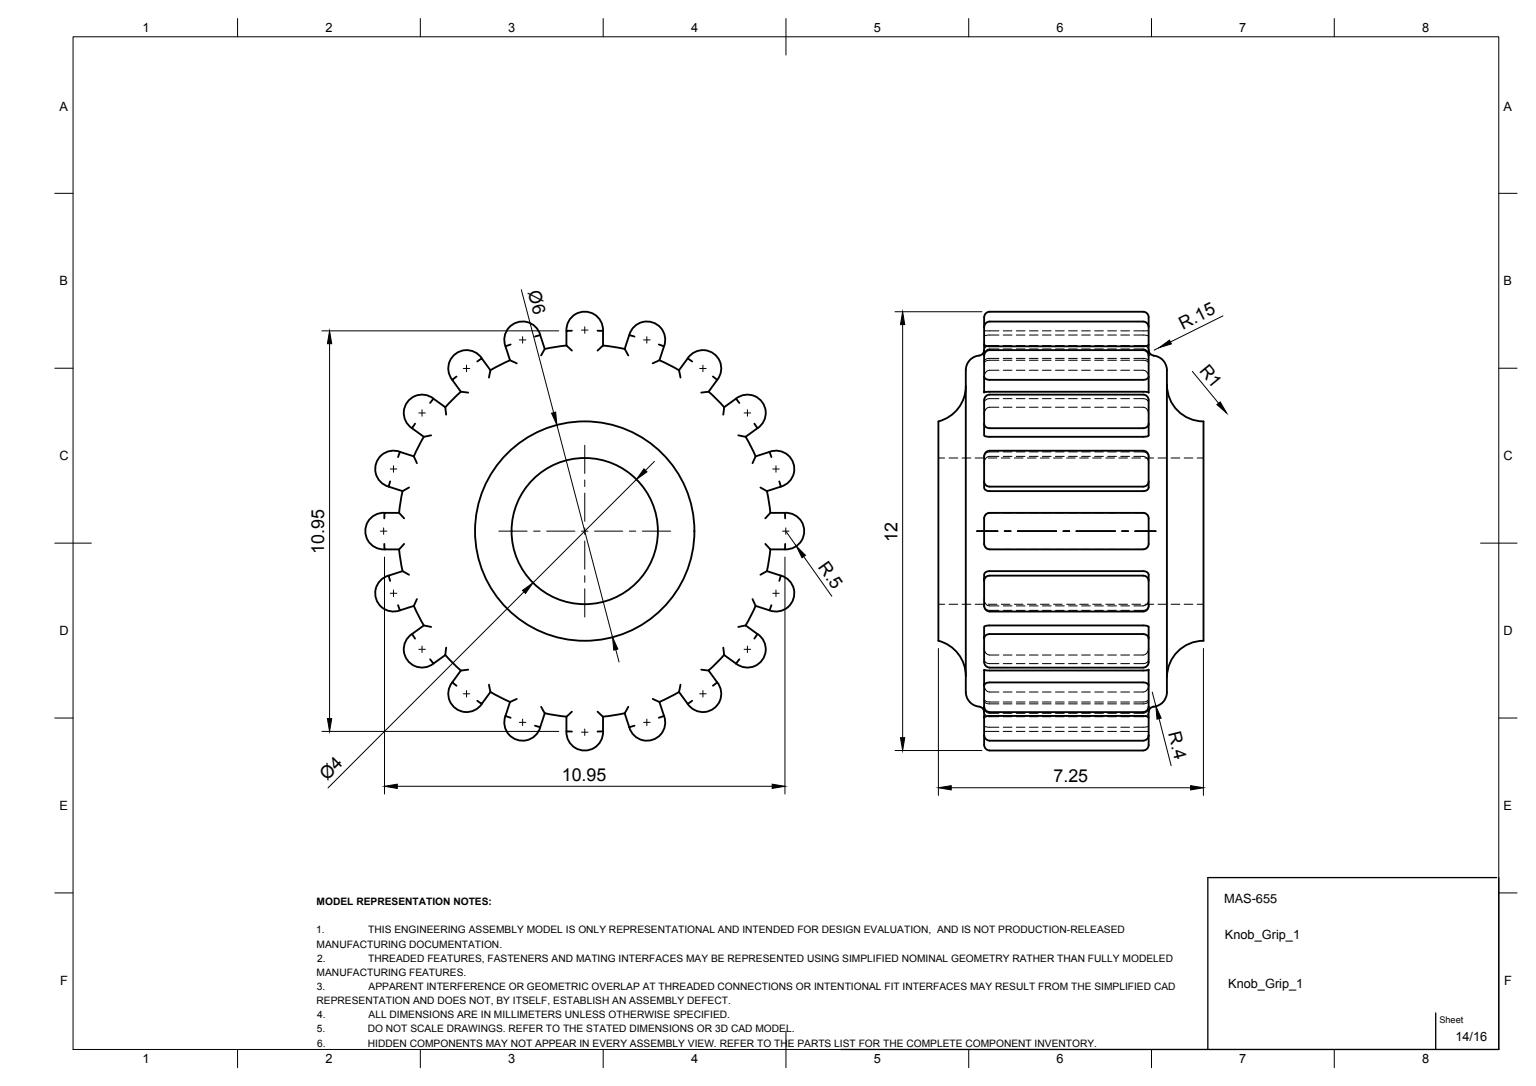
ISO-10303-21;
HEADER;
FILE_DESCRIPTION((''),'2;1');
FILE_NAME('Knob_Grip_1.step','2026-10-09T11:34:15-07:00',(''),(''),'','','');
FILE_SCHEMA (('AUTOMOTIVE_DESIGN { 1 0 10303 214 3 1 1 }'));
ENDSEC;
DATA;
#10=MECHANICAL_DESIGN_GEOMETRIC_PRESENTATION_REPRESENTATION('',(#646),#117170);
#604=SHAPE_REPRESENTATION_RELATIONSHIP('SRR','None',#117259,#625) ;
#625=ADVANCED_BREP_SHAPE_REPRESENTATION('',(#667),#117167) ;
#646=STYLED_ITEM('',(#117355),#667) ;
#667=MANIFOLD_SOLID_BREP('Body1',#49075) ;
#762=FACE_BOUND('',#16420,.T.) ;
#763=FACE_BOUND('',#16423,.T.) ;
#764=FACE_BOUND('',#16425,.T.) ;
#765=FACE_BOUND('',#16427,.T.) ;
#1361=B_SPLINE_CURVE_WITH_KNOTS('',3,(#101754,#101755,#101756,#101757,#101758,
#101759,#101760,#101761,#101762,#101763,#101764,#101765,#101766,#101767,
#101768,#101769),.UNSPECIFIED.,.T.,.F.,(4,1,1,1,1,1,1,1,1,1,1,1,1,4),(-1.37470975898194,
-1.17832265055595,-0.981935542129957,-0.785548433703966,-0.589161325277974,
-0.392774216851983,-0.196387108425991,0.,0.196387108425991,0.589161325277974,
0.785548433703966,0.981935542129957,1.17832265055595,1.37470975898194),
 .UNSPECIFIED.) ;
#1362=B_SPLINE_CURVE_WITH_KNOTS('',3,(#101778,#101779,#101780,#101781,#101782,
#101783,#101784,#101785,#101786,#101787,#101788,#101789,#101790,#101791,
#101792,#101793),.UNSPECIFIED.,.T.,.F.,(4,1,1,1,1,1,1,1,1,1,1,1,1,4),(-1.37470975898194,
-1.17832265055595,-0.981935542129957,-0.785548433703966,-0.589161325277974,
-0.392774216851983,-0.196387108425991,0.,0.196387108425991,0.589161325277974,
0.785548433703966,0.981935542129957,1.17832265055595,1.37470975898194),
 .UNSPECIFIED.) ;
#1363=B_SPLINE_CURVE_WITH_KNOTS('',3,(#101881,#101882,#101883,#101884,#101885),
 .UNSPECIFIED.,.F.,.F.,(4,1,4),(-1.,-0.5,0.),.UNSPECIFIED.) ;
#1364=B_SPLINE_CURVE_WITH_KNOTS('',3,(#101887,#101888,#101889,#101890,#101891,
#101892,#101893),.UNSPECIFIED.,.F.,.F.,(4,1,1,1,4),(-1.37470975898194,-1.17832265055595,
-0.981935542129957,-0.785548433703966,-0.68713324456091),.UNSPECIFIED.) ;
#1365=B_SPLINE_CURVE_WITH_KNOTS('',3,(#101894,#101895,#101896,#101897,#101898,
#101899,#101900,#101901,#101902,#101903,#101904,#101905,#101906),
 .UNSPECIFIED.,.F.,.F.,(4,1,1,1,1,1,1,1,1,1,4),(-0.68713324456091,-0.589161325277974,
-0.196387108425991,0.,0.196387108425991,0.392774216851983,0.589161325277974,
0.785548433703966,0.981935542129957,1.17832265055595,1.37470975898194),
 .UNSPECIFIED.) ;
#1366=B_SPLINE_CURVE_WITH_KNOTS('',3,(#101988,#101989,#101990,#101991,#101992),
 .UNSPECIFIED.,.F.,.F.,(4,1,4),(-1.,-0.5,0.),.UNSPECIFIED.) ;
#1367=B_SPLINE_CURVE_WITH_KNOTS('',3,(#101994,#101995,#101996,#101997,#101998,
#101999,#102000),.UNSPECIFIED.,.F.,.F.,(4,1,1,1,4),(-1.37470975898194,-1.17832265055595,
-0.981935542129957,-0.785548433703966,-0.687210817221056),.UNSPECIFIED.) ;
#1368=B_SPLINE_CURVE_WITH_KNOTS('',3,(#102001,#102002,#102003,#102004,#102005,
#102006,#102007,#102008,#102009,#102010,#102011,#102012,#102013),
 .UNSPECIFIED.,.F.,.F.,(4,1,1,1,1,1,1,1,1,1,4),(-0.687210817221056,-0.589161325277974,
-0.196387108425991,0.,0.196387108425991,0.392774216851983,0.589161325277974,
0.785548433703966,0.981935542129957,1.17832265055595,1.37470975898194),
 .UNSPECIFIED.) ;
#1369=B_SPLINE_CURVE_WITH_KNOTS('',3,(#102019,#102020,#102021,#102022,#102023,
#102024,#102025,#102026,#102027,#102028,#102029,#102030,#102031,#102032),
 .UNSPECIFIED.,.F.,.F.,(4,2,2,2,2,2,4),(-0.0559250143496373,-0.0556883945460747,
-0.0495906031992305,-0.0437546843030053,-0.0372885759081072,-0.0322854917709823,
-0.0278441972730634),.UNSPECIFIED.) ;
#1370=B_SPLINE_CURVE_WITH_KNOTS('',3,(#102035,#102036,#102037,#102038,#102039,
#102040,#102041,#102042,#102043,#102044,#102045,#102046,#102047,#102048),
 .UNSPECIFIED.,.F.,.F.,(4,2,2,2,2,2,4),(-0.000236619804093,0.,0.0060977913471935,
0.0119337102438738,0.018399818639261,0.0234029027767472,0.0278441972749678),
 .UNSPECIFIED.) ;
#1371=B_SPLINE_CURVE_WITH_KNOTS('',3,(#102053,#102054,#102055,#102056,#102057,
#102058,#102059,#102060,#102061,#102062,#102063,#102064,#102065,#102066,
#102067,#102068),.UNSPECIFIED.,.F.,.F.,(4,3,3,3,3,4),(-0.000437598556087367,
0.,0.00562170475705654,0.0114823251607832,0.0173413775084489,0.0231997078489075),
 .UNSPECIFIED.) ;
#1372=B_SPLINE_CURVE_WITH_KNOTS('',3,(#102074,#102075,#102076,#102077,#102078,
#102079,#102080,#102081,#102082,#102083,#102084,#102085,#102086,#102087,
#102088,#102089),.UNSPECIFIED.,.F.,.F.,(4,3,3,3,3,4),(-0.046837014255361,
-0.046399415699481,-0.0407777109422933,-0.0349170905383532,-0.0290580381904547,
-0.0231997078497599),.UNSPECIFIED.) ;
#1373=B_SPLINE_CURVE_WITH_KNOTS('',3,(#102095,#102096,#102097,#102098,#102099,
#102100,#102101,#102102,#102103,#102104,#102105,#102106,#102107,#102108),
 .UNSPECIFIED.,.F.,.F.,(4,2,2,2,2,2,4),(-0.000236619803146698,0.,0.00609779134724104,
0.0119337102438844,0.0183998186389394,0.0234029027761802,0.0278441972742087),
 .UNSPECIFIED.) ;
#1374=B_SPLINE_CURVE_WITH_KNOTS('',3,(#102114,#102115,#102116,#102117,#102118,
#102119,#102120,#102121,#102122,#102123,#102124,#102125,#102126,#102127),
 .UNSPECIFIED.,.F.,.F.,(4,2,2,2,2,2,4),(-0.0559250143496986,-0.0556883945465552,
-0.0495906031994403,-0.0437546843028884,-0.0372885759079096,-0.0322854917707418,
-0.0278441972727803),.UNSPECIFIED.) ;
#1375=B_SPLINE_CURVE_WITH_KNOTS('',3,(#102133,#102134,#102135,#102136,#102137,
#102138,#102139,#102140,#102141,#102142,#102143,#102144,#102145,#102146,
#102147,#102148),.UNSPECIFIED.,.F.,.F.,(4,3,3,3,3,4),(-0.000437598556095027,
0.,0.00562170475708189,0.0114823251608833,0.0173413775086171,0.0231997078491342),
 .UNSPECIFIED.) ;
#1376=B_SPLINE_CURVE_WITH_KNOTS('',3,(#102154,#102155,#102156,#102157,#102158,
#102159,#102160,#102161,#102162,#102163,#102164,#102165,#102166,#102167,
#102168,#102169),.UNSPECIFIED.,.F.,.F.,(4,3,3,3,3,4),(-0.0468370142541051,
-0.0463994156980201,-0.0407777109409428,-0.0349170905371886,-0.0290580381894966,
-0.0231997078490079),.UNSPECIFIED.) ;
#1377=B_SPLINE_CURVE_WITH_KNOTS('',3,(#102175,#102176,#102177,#102178,#102179,
#102180,#102181,#102182,#102183,#102184,#102185,#102186,#102187,#102188),
 .UNSPECIFIED.,.F.,.F.,(4,2,2,2,2,2,4),(-0.000236619803558265,0.,0.00609779134685418,
0.0119337102431074,0.0183998186379772,0.023402902775095,0.0278441972730209),
 .UNSPECIFIED.) ;
#1378=B_SPLINE_CURVE_WITH_KNOTS('',3,(#102194,#102195,#102196,#102197,#102198,
#102199,#102200,#102201,#102202,#102203,#102204,#102205,#102206,#102207),
 .UNSPECIFIED.,.F.,.F.,(4,2,2,2,2,2,4),(-0.0559250143504567,-0.0556883945473107,
-0.0495906032000867,-0.0437546843034773,-0.0372885759084374,-0.0322854917711889,
-0.0278441972731474),.UNSPECIFIED.) ;
#1379=B_SPLINE_CURVE_WITH_KNOTS('',3,(#102213,#102214,#102215,#102216,#102217,
#102218,#102219,#102220,#102221,#102222,#102223,#102224,#102225,#102226,
#102227,#102228),.UNSPECIFIED.,.F.,.F.,(4,3,3,3,3,4),(-0.000437598556114517,
0.,0.00562170475723958,0.0114823251612343,0.0173413775091901,0.0231997078499022),
 .UNSPECIFIED.) ;
#1380=B_SPLINE_CURVE_WITH_KNOTS('',3,(#102234,#102235,#102236,#102237,#102238,
#102239,#102240,#102241,#102242,#102243,#102244,#102245,#102246,#102247,
#102248,#102249),.UNSPECIFIED.,.F.,.F.,(4,3,3,3,3,4),(-0.0468370142516818,
-0.046399415695612,-0.0407777109388244,-0.034917090535398,-0.0290580381880315,
-0.0231997078478665),.UNSPECIFIED.) ;
#1381=B_SPLINE_CURVE_WITH_KNOTS('',3,(#102255,#102256,#102257,#102258,#102259,
#102260,#102261,#102262,#102263,#102264,#102265,#102266,#102267,#102268),
 .UNSPECIFIED.,.F.,.F.,(4,2,2,2,2,2,4),(-0.000236619803559768,0.,0.00609779134686269,
0.0119337102430971,0.0183998186379832,0.0234029027750867,0.0278441972729811),
 .UNSPECIFIED.) ;
#1382=B_SPLINE_CURVE_WITH_KNOTS('',3,(#102274,#102275,#102276,#102277,#102278,
#102279,#102280,#102281,#102282,#102283,#102284,#102285,#102286,#102287),
 .UNSPECIFIED.,.F.,.F.,(4,2,2,2,2,2,4),(-0.0559250143524368,-0.0556883945478243,
-0.0495906032010392,-0.0437546843047665,-0.0372885759096309,-0.0322854917723447,
-0.0278441972742818),.UNSPECIFIED.) ;
#1383=B_SPLINE_CURVE_WITH_KNOTS('',3,(#102293,#102294,#102295,#102296,#102297,
#102298,#102299,#102300,#102301,#102302,#102303,#102304,#102305,#102306,
#102307,#102308),.UNSPECIFIED.,.F.,.F.,(4,3,3,3,3,4),(-0.000437598556131605,
0.,0.00562170475733242,0.0114823251614144,0.0173413775094361,0.0231997078502398),
 .UNSPECIFIED.) ;
#1384=B_SPLINE_CURVE_WITH_KNOTS('',3,(#102314,#102315,#102316,#102317,#102318,
#102319,#102320,#102321,#102322,#102323,#102324,#102325,#102326,#102327,
#102328,#102329),.UNSPECIFIED.,.F.,.F.,(4,3,3,3,3,4),(-0.0468370142582233,
-0.0463994157019922,-0.0407777109444557,-0.0349170905401249,-0.0290580381918459,
-0.0231997078507989),.UNSPECIFIED.) ;
#1385=B_SPLINE_CURVE_WITH_KNOTS('',3,(#102335,#102336,#102337,#102338,#102339,
#102340,#102341,#102342,#102343,#102344,#102345,#102346,#102347,#102348),
 .UNSPECIFIED.,.F.,.F.,(4,2,2,2,2,2,4),(-0.000236619803154501,0.,0.00609779134749395,
0.0119337102444787,0.0183998186399401,0.0234029027774939,0.0278441972757804),
 .UNSPECIFIED.) ;
#1386=B_SPLINE_CURVE_WITH_KNOTS('',3,(#102354,#102355,#102356,#102357,#102358,
#102359,#102360,#102361,#102362,#102363,#102364,#102365,#102366,#102367),
 .UNSPECIFIED.,.F.,.F.,(4,2,2,2,2,2,4),(-0.0559250143516698,-0.055688394548102,
-0.0495906032010132,-0.0437546843045191,-0.0372885759093257,-0.0322854917720022,
-0.0278441972739074),.UNSPECIFIED.) ;
#1387=B_SPLINE_CURVE_WITH_KNOTS('',3,(#102373,#102374,#102375,#102376,#102377,
#102378,#102379,#102380,#102381,#102382,#102383,#102384,#102385,#102386,
#102387,#102388),.UNSPECIFIED.,.F.,.F.,(4,3,3,3,3,4),(-0.000437598556150276,
0.,0.00562170475744494,0.0114823251616921,0.0173413775098778,0.0231997078508276),
 .UNSPECIFIED.) ;
#1388=B_SPLINE_CURVE_WITH_KNOTS('',3,(#102394,#102395,#102396,#102397,#102398,
#102399,#102400,#102401,#102402,#102403,#102404,#102405,#102406,#102407,
#102408,#102409),.UNSPECIFIED.,.F.,.F.,(4,3,3,3,3,4),(-0.0468370142569828,
-0.0463994157014635,-0.0407777109440522,-0.0349170905398014,-0.0290580381915951,
-0.0231997078506218),.UNSPECIFIED.) ;
#1389=B_SPLINE_CURVE_WITH_KNOTS('',3,(#102415,#102416,#102417,#102418,#102419,
#102420,#102421,#102422,#102423,#102424,#102425,#102426,#102427,#102428),
 .UNSPECIFIED.,.F.,.F.,(4,2,2,2,2,2,4),(-0.000236619804616541,0.,0.00609779134700319,
0.0119337102434886,0.0183998186388943,0.0234029027763847,0.0278441972746185),
 .UNSPECIFIED.) ;
#1390=B_SPLINE_CURVE_WITH_KNOTS('',3,(#102434,#102435,#102436,#102437,#102438,
#102439,#102440,#102441,#102442,#102443,#102444,#102445,#102446,#102447),
 .UNSPECIFIED.,.F.,.F.,(4,2,2,2,2,2,4),(-0.0559250143475551,-0.0556883945439973,
-0.049590603197355,-0.0437546843013896,-0.037288575906807,-0.0322854917699323,
-0.0278441972722247),.UNSPECIFIED.) ;
#1391=B_SPLINE_CURVE_WITH_KNOTS('',3,(#102453,#102454,#102455,#102456,#102457,
#102458,#102459,#102460,#102461,#102462,#102463,#102464,#102465,#102466,
#102467,#102468),.UNSPECIFIED.,.F.,.F.,(4,3,3,3,3,4),(-0.000437598556056009,
0.,0.00562170475686937,0.0114823251603833,0.0173413775078316,0.0231997078480834),
 .UNSPECIFIED.) ;
#1392=B_SPLINE_CURVE_WITH_KNOTS('',3,(#102474,#102475,#102476,#102477,#102478,
#102479,#102480,#102481,#102482,#102483,#102484,#102485,#102486,#102487,
#102488,#102489),.UNSPECIFIED.,.F.,.F.,(4,3,3,3,3,4),(-0.0468370142561097,
-0.0463994157004828,-0.0407777109431283,-0.034917090538975,-0.0290580381908889,
-0.0231997078500392),.UNSPECIFIED.) ;
#1393=B_SPLINE_CURVE_WITH_KNOTS('',3,(#102495,#102496,#102497,#102498,#102499,
#102500,#102501,#102502,#102503,#102504,#102505,#102506,#102507,#102508),
 .UNSPECIFIED.,.F.,.F.,(4,2,2,2,2,2,4),(-0.000236619804206572,0.,0.00609779134739848,
0.0119337102443252,0.0183998186399927,0.023402902777706,0.0278441972760964),
 .UNSPECIFIED.) ;
#1394=B_SPLINE_CURVE_WITH_KNOTS('',3,(#102514,#102515,#102516,#102517,#102518,
#102519,#102520,#102521,#102522,#102523,#102524,#102525,#102526,#102527),
 .UNSPECIFIED.,.F.,.F.,(4,2,2,2,2,2,4),(-0.0559250143503367,-0.0556883945467745,
-0.0495906031998185,-0.0437546843034772,-0.0372885759085197,-0.0322854917713411,
-0.0278441972733722),.UNSPECIFIED.) ;
#1395=B_SPLINE_CURVE_WITH_KNOTS('',3,(#102533,#102534,#102535,#102536,#102537,
#102538,#102539,#102540,#102541,#102542,#102543,#102544,#102545,#102546,
#102547,#102548),.UNSPECIFIED.,.F.,.F.,(4,3,3,3,3,4),(-0.000437598556095159,
0.,0.00562170475710087,0.0114823251609001,0.0173413775086179,0.0231997078491324),
 .UNSPECIFIED.) ;
#1396=B_SPLINE_CURVE_WITH_KNOTS('',3,(#102554,#102555,#102556,#102557,#102558,
#102559,#102560,#102561,#102562,#102563,#102564,#102565,#102566,#102567,
#102568,#102569),.UNSPECIFIED.,.F.,.F.,(4,3,3,3,3,4),(-0.0468370142542446,
-0.0463994156981747,-0.0407777109410807,-0.0349170905373078,-0.0290580381895938,
-0.0231997078490836),.UNSPECIFIED.) ;
#1397=B_SPLINE_CURVE_WITH_KNOTS('',3,(#102575,#102576,#102577,#102578,#102579,
#102580,#102581,#102582,#102583,#102584,#102585,#102586,#102587,#102588),
 .UNSPECIFIED.,.F.,.F.,(4,2,2,2,2,2,4),(-0.000236619803563725,0.,0.00609779134693619,
0.0119337102432759,0.0183998186382373,0.0234029027754271,0.027844197273412),
 .UNSPECIFIED.) ;
#1398=B_SPLINE_CURVE_WITH_KNOTS('',3,(#102594,#102595,#102596,#102597,#102598,
#102599,#102600,#102601,#102602,#102603,#102604,#102605,#102606,#102607),
 .UNSPECIFIED.,.F.,.F.,(4,2,2,2,2,2,4),(-0.0559250143564113,-0.0556883945522011,
-0.0495906032047249,-0.0437546843077159,-0.0372885759119513,-0.0322854917741759,
-0.0278441972757216),.UNSPECIFIED.) ;
#1399=B_SPLINE_CURVE_WITH_KNOTS('',3,(#102613,#102614,#102615,#102616,#102617,
#102618,#102619,#102620,#102621,#102622,#102623,#102624,#102625,#102626,
#102627,#102628),.UNSPECIFIED.,.F.,.F.,(4,3,3,3,3,4),(-0.000437598556252948,
0.,0.00562170475756358,0.0114823251619473,0.0173413775102792,0.023199707851373),
 .UNSPECIFIED.) ;
#1400=B_SPLINE_CURVE_WITH_KNOTS('',3,(#102634,#102635,#102636,#102637,#102638,
#102639,#102640,#102641,#102642,#102643,#102644,#102645,#102646,#102647,
#102648,#102649),.UNSPECIFIED.,.F.,.F.,(4,3,3,3,3,4),(-0.0468370142435449,
-0.0463994156880452,-0.0407777109322271,-0.0349170905298351,-0.0290580381834779,
-0.0231997078443083),.UNSPECIFIED.) ;
#1401=B_SPLINE_CURVE_WITH_KNOTS('',3,(#102655,#102656,#102657,#102658,#102659,
#102660,#102661,#102662,#102663,#102664,#102665,#102666,#102667,#102668),
 .UNSPECIFIED.,.F.,.F.,(4,2,2,2,2,2,4),(-0.000236619803545348,0.,0.00609779134648851,
0.0119337102422953,0.0183998186366923,0.0234029027734222,0.0278441972710204),
 .UNSPECIFIED.) ;
#1402=B_SPLINE_CURVE_WITH_KNOTS('',3,(#102674,#102675,#102676,#102677,#102678,
#102679,#102680,#102681,#102682,#102683,#102684,#102685,#102686,#102687),
 .UNSPECIFIED.,.F.,.F.,(4,2,2,2,2,2,4),(-0.0559250143495547,-0.0556883945459923,
-0.0495906031991245,-0.0437546843029074,-0.0372885759080479,-0.0322854917709575,
-0.027844197273083),.UNSPECIFIED.) ;
#1403=B_SPLINE_CURVE_WITH_KNOTS('',3,(#102693,#102694,#102695,#102696,#102697,
#102698,#102699,#102700,#102701,#102702,#102703,#102704,#102705,#102706,
#102707,#102708),.UNSPECIFIED.,.F.,.F.,(4,3,3,3,3,4),(-0.000437598556080383,
0.,0.00562170475701161,0.0114823251606741,0.0173413775082905,0.0231997078487108),
 .UNSPECIFIED.) ;
#1404=B_SPLINE_CURVE_WITH_KNOTS('',3,(#102714,#102715,#102716,#102717,#102718,
#102719,#102720,#102721,#102722,#102723,#102724,#102725,#102726,#102727,
#102728,#102729),.UNSPECIFIED.,.F.,.F.,(4,3,3,3,3,4),(-0.0468370142410635,
-0.046399415685515,-0.0407777109299654,-0.0349170905279156,-0.0290580381819153,
-0.0231997078430871),.UNSPECIFIED.) ;
#1405=B_SPLINE_CURVE_WITH_KNOTS('',3,(#102735,#102736,#102737,#102738,#102739,
#102740,#102741,#102742,#102743,#102744,#102745,#102746,#102747,#102748),
 .UNSPECIFIED.,.F.,.F.,(4,2,2,2,2,2,4),(-0.000236619803553881,0.,0.00609779134648714,
0.0119337102422593,0.0183998186365944,0.0234029027733178,0.0278441972709114),
 .UNSPECIFIED.) ;
#1406=B_SPLINE_CURVE_WITH_KNOTS('',3,(#102754,#102755,#102756,#102757,#102758,
#102759,#102760,#102761,#102762,#102763,#102764,#102765,#102766,#102767),
 .UNSPECIFIED.,.F.,.F.,(4,2,2,2,2,2,4),(-0.0559250143458346,-0.0556883945427038,
-0.0495906031960554,-0.043754684300065,-0.0372885759056522,-0.0322854917688908,
-0.0278441972712752),.UNSPECIFIED.) ;
#1407=B_SPLINE_CURVE_WITH_KNOTS('',3,(#102773,#102774,#102775,#102776,#102777,
#102778,#102779,#102780,#102781,#102782,#102783,#102784,#102785,#102786,
#102787,#102788),.UNSPECIFIED.,.F.,.F.,(4,3,3,3,3,4),(-0.000437598556037642,
0.,0.00562170475676515,0.0114823251601515,0.0173413775075229,0.0231997078477011),
 .UNSPECIFIED.) ;
#1408=B_SPLINE_CURVE_WITH_KNOTS('',3,(#102794,#102795,#102796,#102797,#102798,
#102799,#102800,#102801,#102802,#102803,#102804,#102805,#102806,#102807,
#102808,#102809),.UNSPECIFIED.,.F.,.F.,(4,3,3,3,3,4),(-0.0468370142550307,
-0.046399415699245,-0.0407777109420836,-0.0349170905381485,-0.0290580381902572,
-0.023199707849583),.UNSPECIFIED.) ;
#1409=B_SPLINE_CURVE_WITH_KNOTS('',3,(#102815,#102816,#102817,#102818,#102819,
#102820,#102821,#102822,#102823,#102824,#102825,#102826,#102827,#102828),
 .UNSPECIFIED.,.F.,.F.,(4,2,2,2,2,2,4),(-0.000236619803565948,0.,0.00609779134700125,
0.0119337102434307,0.0183998186384978,0.0234029027757452,0.0278441972737845),
 .UNSPECIFIED.) ;
#1410=B_SPLINE_CURVE_WITH_KNOTS('',3,(#102834,#102835,#102836,#102837,#102838,
#102839,#102840,#102841,#102842,#102843,#102844,#102845,#102846,#102847),
 .UNSPECIFIED.,.F.,.F.,(4,2,2,2,2,2,4),(-0.0559250143492506,-0.0556883945457476,
-0.049590603198939,-0.0437546843027145,-0.0372885759078682,-0.032285491770796,
-0.0278441972729179),.UNSPECIFIED.) ;
#1411=B_SPLINE_CURVE_WITH_KNOTS('',3,(#102854,#102855,#102856,#102857,#102858,
#102859,#102860,#102861,#102862,#102863,#102864,#102865,#102866,#102867,
#102868,#102869),.UNSPECIFIED.,.F.,.F.,(4,3,3,3,3,4),(-0.000437598556107252,
0.,0.00562170475708925,0.0114823251608564,0.0173413775085622,0.0231997078490661),
 .UNSPECIFIED.) ;
#1412=B_SPLINE_CURVE_WITH_KNOTS('',3,(#102875,#102876,#102877,#102878,#102879,
#102880,#102881,#102882,#102883,#102884,#102885,#102886,#102887,#102888,
#102889,#102890),.UNSPECIFIED.,.F.,.F.,(4,3,3,3,3,4),(-0.0468370142553995,
-0.0463994157003126,-0.0407777109430307,-0.0349170905389541,-0.0290580381909493,
-0.0231997078501516),.UNSPECIFIED.) ;
#1413=B_SPLINE_CURVE_WITH_KNOTS('',3,(#102896,#102897,#102898,#102899,#102900,
#102901,#102902,#102903,#102904,#102905,#102906,#102907,#102908,#102909),
 .UNSPECIFIED.,.F.,.F.,(4,2,2,2,2,2,4),(-0.000236619803559952,0.,0.00609779134694098,
0.0119337102432763,0.0183998186382272,0.0234029027754186,0.0278441972733939),
 .UNSPECIFIED.) ;
#1414=B_SPLINE_CURVE_WITH_KNOTS('',3,(#102915,#102916,#102917,#102918,#102919,
#102920,#102921,#102922,#102923,#102924,#102925,#102926,#102927,#102928),
 .UNSPECIFIED.,.F.,.F.,(4,2,2,2,2,2,4),(-0.0559250143507825,-0.0556883945467992,
-0.0495906032001226,-0.043754684304009,-0.0372885759090493,-0.032285491771857,
-0.0278441972738728),.UNSPECIFIED.) ;
#1415=B_SPLINE_CURVE_WITH_KNOTS('',3,(#102934,#102935,#102936,#102937,#102938,
#102939,#102940,#102941,#102942,#102943,#102944,#102945,#102946,#102947,
#102948,#102949),.UNSPECIFIED.,.F.,.F.,(4,3,3,3,3,4),(-0.000437598556095639,
0.,0.00562170475706734,0.0114823251608502,0.0173413775085488,0.0231997078490271),
 .UNSPECIFIED.) ;
#1416=B_SPLINE_CURVE_WITH_KNOTS('',3,(#102955,#102956,#102957,#102958,#102959,
#102960,#102961,#102962,#102963,#102964,#102965,#102966,#102967,#102968,
#102969,#102970),.UNSPECIFIED.,.F.,.F.,(4,3,3,3,3,4),(-0.0468370142543074,
-0.0463994156982126,-0.0407777109411238,-0.0349170905373201,-0.0290580381896051,
-0.0231997078491063),.UNSPECIFIED.) ;
#1417=B_SPLINE_CURVE_WITH_KNOTS('',3,(#102976,#102977,#102978,#102979,#102980,
#102981,#102982,#102983,#102984,#102985,#102986,#102987,#102988,#102989),
 .UNSPECIFIED.,.F.,.F.,(4,2,2,2,2,2,4),(-0.000236619803981649,0.,0.00609779134664719,
0.0119337102427236,0.0183998186376455,0.0234029027747974,0.0278441972727449),
 .UNSPECIFIED.) ;
#1418=B_SPLINE_CURVE_WITH_KNOTS('',3,(#102995,#102996,#102997,#102998,#102999,
#103000,#103001,#103002,#103003,#103004,#103005,#103006,#103007,#103008),
 .UNSPECIFIED.,.F.,.F.,(4,2,2,2,2,2,4),(-0.055925014352087,-0.0556883945480977,
-0.0495906032012405,-0.0437546843049561,-0.0372885759098064,-0.0322854917724869,
-0.0278441972743996),.UNSPECIFIED.) ;
#1419=B_SPLINE_CURVE_WITH_KNOTS('',3,(#103014,#103015,#103016,#103017,#103018,
#103019,#103020,#103021,#103022,#103023,#103024,#103025,#103026,#103027,
#103028,#103029),.UNSPECIFIED.,.F.,.F.,(4,3,3,3,3,4),(-0.000437598556128711,
0.,0.00562170475726701,0.0114823251612751,0.0173413775092439,0.0231997078500064),
 .UNSPECIFIED.) ;
#1420=B_SPLINE_CURVE_WITH_KNOTS('',3,(#103035,#103036,#103037,#103038,#103039,
#103040,#103041,#103042,#103043,#103044,#103045,#103046,#103047,#103048,
#103049,#103050),.UNSPECIFIED.,.F.,.F.,(4,3,3,3,3,4),(-0.0468370142525421,
-0.046399415696666,-0.0407777109397685,-0.0349170905362003,-0.029058038188693,
-0.0231997078483865),.UNSPECIFIED.) ;
#1421=B_SPLINE_CURVE_WITH_KNOTS('',3,(#103056,#103057,#103058,#103059,#103060,
#103061,#103062,#103063,#103064,#103065,#103066,#103067,#103068,#103069),
 .UNSPECIFIED.,.F.,.F.,(4,2,2,2,2,2,4),(-0.000236619803982414,0.,0.00609779134661,
0.0119337102426289,0.0183998186375097,0.0234029027746178,0.0278441972725225),
 .UNSPECIFIED.) ;
#1422=B_SPLINE_CURVE_WITH_KNOTS('',3,(#103075,#103076,#103077,#103078,#103079,
#103080,#103081,#103082,#103083,#103084,#103085,#103086,#103087,#103088),
 .UNSPECIFIED.,.F.,.F.,(4,2,2,2,2,2,4),(-0.0559250143493171,-0.0556883945461739,
-0.0495906031990541,-0.0437546843026118,-0.037288575907723,-0.0322854917706097,
-0.0278441972727174),.UNSPECIFIED.) ;
#1423=B_SPLINE_CURVE_WITH_KNOTS('',3,(#103094,#103095,#103096,#103097,#103098,
#103099,#103100,#103101,#103102,#103103,#103104,#103105,#103106,#103107,
#103108,#103109),.UNSPECIFIED.,.F.,.F.,(4,3,3,3,3,4),(-0.000437598556087196,
0.,0.00562170475699019,0.0114823251606472,0.0173413775082489,0.0231997078486377),
 .UNSPECIFIED.) ;
#1424=B_SPLINE_CURVE_WITH_KNOTS('',3,(#103115,#103116,#103117,#103118,#103119,
#103120,#103121,#103122,#103123,#103124,#103125,#103126,#103127,#103128,
#103129,#103130),.UNSPECIFIED.,.F.,.F.,(4,3,3,3,3,4),(-0.0468370142500863,
-0.0463994156945211,-0.0407777109379294,-0.0349170905346585,-0.0290580381874365,
-0.0231997078474141),.UNSPECIFIED.) ;
#1425=B_SPLINE_CURVE_WITH_KNOTS('',3,(#103136,#103137,#103138,#103139,#103140,
#103141,#103142,#103143,#103144,#103145,#103146,#103147,#103148,#103149),
 .UNSPECIFIED.,.F.,.F.,(4,2,2,2,2,2,4),(-0.000236619803560014,0.,0.00609779134678491,
0.0119337102429536,0.0183998186377476,0.0234029027747679,0.0278441972725981),
 .UNSPECIFIED.) ;
#1426=B_SPLINE_CURVE_WITH_KNOTS('',3,(#103155,#103156,#103157,#103158,#103159,
#103160,#103161,#103162,#103163,#103164,#103165,#103166,#103167,#103168),
 .UNSPECIFIED.,.F.,.F.,(4,2,2,2,2,2,4),(-0.0559250143548778,-0.0556883945506748,
-0.0495906032033264,-0.0437546843064839,-0.0372885759109464,-0.0322854917733345,
-0.0278441972750097),.UNSPECIFIED.) ;
#1427=B_SPLINE_CURVE_WITH_KNOTS('',3,(#103174,#103175,#103176,#103177,#103178,
#103179,#103180,#103181,#103182,#103183,#103184,#103185,#103186,#103187,
#103188,#103189),.UNSPECIFIED.,.F.,.F.,(4,3,3,3,3,4),(-0.000437598556223204,
0.,0.00562170475783914,0.0114823251625445,0.0173413775111918,0.0231997078526027),
 .UNSPECIFIED.) ;
#1428=B_SPLINE_CURVE_WITH_KNOTS('',3,(#103195,#103196,#103197,#103198,#103199,
#103200,#103201,#103202,#103203,#103204,#103205,#103206,#103207,#103208,
#103209,#103210),.UNSPECIFIED.,.F.,.F.,(4,3,3,3,3,4),(-0.0468370142563843,
-0.046399415700489,-0.0407777109431322,-0.0349170905389995,-0.0290580381909307,
-0.0231997078501088),.UNSPECIFIED.) ;
#1429=B_SPLINE_CURVE_WITH_KNOTS('',3,(#103216,#103217,#103218,#103219,#103220,
#103221,#103222,#103223,#103224,#103225,#103226,#103227,#103228,#103229),
 .UNSPECIFIED.,.F.,.F.,(4,2,2,2,2,2,4),(-0.000236619804200277,0.,0.00609779134716414,
0.0119337102438048,0.0183998186391783,0.0234029027766296,0.0278441972748296),
 .UNSPECIFIED.) ;
#1430=B_SPLINE_CURVE_WITH_KNOTS('',3,(#103235,#103236,#103237,#103238,#103239,
#103240,#103241,#103242,#103243,#103244,#103245,#103246,#103247,#103248),
 .UNSPECIFIED.,.F.,.F.,(4,2,2,2,2,2,4),(-0.0559250143496621,-0.0556883945461033,
-0.0495906031992651,-0.0437546843029983,-0.0372885759081094,-0.032285491771005,
-0.02784419727311),.UNSPECIFIED.) ;
#1431=B_SPLINE_CURVE_WITH_KNOTS('',3,(#103254,#103255,#103256,#103257,#103258,
#103259,#103260,#103261,#103262,#103263,#103264,#103265,#103266,#103267,
#103268,#103269),.UNSPECIFIED.,.F.,.F.,(4,3,3,3,3,4),(-0.000437598556084584,
0.,0.00562170475697965,0.0114823251606079,0.0173413775081775,0.0231997078485472),
 .UNSPECIFIED.) ;
#1432=B_SPLINE_CURVE_WITH_KNOTS('',3,(#103275,#103276,#103277,#103278,#103279,
#103280,#103281,#103282,#103283,#103284,#103285,#103286,#103287,#103288,
#103289,#103290),.UNSPECIFIED.,.F.,.F.,(4,3,3,3,3,4),(-0.0468370142549382,
-0.0463994156994604,-0.0407777109422707,-0.0349170905383382,-0.0290580381904463,
-0.023199707849757),.UNSPECIFIED.) ;
#1433=B_SPLINE_CURVE_WITH_KNOTS('',3,(#103296,#103297,#103298,#103299,#103300,
#103301,#103302,#103303,#103304,#103305,#103306,#103307,#103308,#103309),
 .UNSPECIFIED.,.F.,.F.,(4,2,2,2,2,2,4),(-0.000236619803568316,0.,0.00609779134701837,
0.0119337102434465,0.0183998186385035,0.0234029027757473,0.0278441972737745),
 .UNSPECIFIED.) ;
#1434=B_SPLINE_CURVE_WITH_KNOTS('',3,(#103315,#103316,#103317,#103318,#103319,
#103320,#103321,#103322,#103323,#103324,#103325,#103326,#103327,#103328),
 .UNSPECIFIED.,.F.,.F.,(4,2,2,2,2,2,4),(-0.0559250143499934,-0.0556883945464304,
-0.0495906031995064,-0.0437546843032007,-0.037288575908277,-0.032285491771123,
-0.0278441972731808),.UNSPECIFIED.) ;
#1435=B_SPLINE_CURVE_WITH_KNOTS('',3,(#103334,#103335,#103336,#103337,#103338,
#103339,#103340,#103341,#103342,#103343,#103344,#103345,#103346,#103347,
#103348,#103349),.UNSPECIFIED.,.F.,.F.,(4,3,3,3,3,4),(-0.000437598556092419,
0.,0.00562170475702671,0.0114823251607112,0.0173413775083605,0.0231997078487915),
 .UNSPECIFIED.) ;
#1436=B_SPLINE_CURVE_WITH_KNOTS('',3,(#103355,#103356,#103357,#103358,#103359,
#103360,#103361,#103362,#103363,#103364,#103365,#103366,#103367,#103368,
#103369,#103370),.UNSPECIFIED.,.F.,.F.,(4,3,3,3,3,4),(-0.0468370142548351,
-0.0463994156987323,-0.0407777109416122,-0.0349170905377609,-0.0290580381899607,
-0.0231997078493697),.UNSPECIFIED.) ;
#1437=B_SPLINE_CURVE_WITH_KNOTS('',3,(#103376,#103377,#103378,#103379,#103380,
#103381,#103382,#103383,#103384,#103385,#103386,#103387,#103388,#103389),
 .UNSPECIFIED.,.F.,.F.,(4,2,2,2,2,2,4),(-0.000236619803562033,0.,0.00609779134691358,
0.0119337102432247,0.0183998186381566,0.0234029027753094,0.027844197273255),
 .UNSPECIFIED.) ;
#1438=B_SPLINE_CURVE_WITH_KNOTS('',3,(#103395,#103396,#103397,#103398,#103399,
#103400,#103401,#103402,#103403,#103404,#103405,#103406,#103407,#103408),
 .UNSPECIFIED.,.F.,.F.,(4,2,2,2,2,2,4),(-0.0559250143503813,-0.0556883945472345,
-0.0495906032000065,-0.0437546843033907,-0.0372885759083472,-0.0322854917711086,
-0.027844197273083),.UNSPECIFIED.) ;
#1439=B_SPLINE_CURVE_WITH_KNOTS('',3,(#103414,#103415,#103416,#103417,#103418,
#103419,#103420,#103421,#103422,#103423,#103424,#103425,#103426,#103427,
#103428,#103429),.UNSPECIFIED.,.F.,.F.,(4,3,3,3,3,4),(-0.000437598556129241,
0.,0.00562170475730571,0.0114823251613513,0.0173413775093445,0.0231997078501172),
 .UNSPECIFIED.) ;
#1440=B_SPLINE_CURVE_WITH_KNOTS('',3,(#103435,#103436,#103437,#103438,#103439,
#103440,#103441,#103442,#103443,#103444,#103445,#103446,#103447,#103448,
#103449,#103450),.UNSPECIFIED.,.F.,.F.,(4,3,3,3,3,4),(-0.0468370142515845,
-0.0463994156955989,-0.0407777109388572,-0.0349170905354382,-0.0290580381880585,
-0.0231997078478789),.UNSPECIFIED.) ;
#1441=B_SPLINE_CURVE_WITH_KNOTS('',3,(#103456,#103457,#103458,#103459,#103460,
#103461,#103462,#103463,#103464,#103465,#103466,#103467,#103468,#103469),
 .UNSPECIFIED.,.F.,.F.,(4,2,2,2,2,2,4),(-0.000236619803559663,0.,0.0060977913468164,
0.0119337102430072,0.0183998186378663,0.0234029027749556,0.0278441972728503),
 .UNSPECIFIED.) ;
#1442=B_SPLINE_CURVE_WITH_KNOTS('',3,(#103475,#103476,#103477,#103478,#103479,
#103480,#103481,#103482,#103483,#103484,#103485,#103486,#103487,#103488),
 .UNSPECIFIED.,.F.,.F.,(4,2,2,2,2,2,4),(-0.0559250143533661,-0.0556883945491649,
-0.0495906032019838,-0.0437546843053393,-0.0372885759099808,-0.0322854917725361,
-0.0278441972743507),.UNSPECIFIED.) ;
#1443=B_SPLINE_CURVE_WITH_KNOTS('',3,(#103494,#103495,#103496,#103497,#103498,
#103499,#103500,#103501,#103502,#103503,#103504,#103505,#103506,#103507,
#103508,#103509),.UNSPECIFIED.,.F.,.F.,(4,3,3,3,3,4),(-0.00043759855615984,
0.,0.00562170475737693,0.011482325161534,0.017341377509665,0.0231997078505602),
 .UNSPECIFIED.) ;
#1444=B_SPLINE_CURVE_WITH_KNOTS('',3,(#103515,#103516,#103517,#103518,#103519,
#103520,#103521,#103522,#103523,#103524,#103525,#103526,#103527,#103528,
#103529,#103530),.UNSPECIFIED.,.F.,.F.,(4,3,3,3,3,4),(-0.0468370142504761,
-0.0463994156944377,-0.0407777109378315,-0.0349170905345851,-0.0290580381873817,
-0.0231997078473671),.UNSPECIFIED.) ;
#1445=B_SPLINE_CURVE_WITH_KNOTS('',3,(#103536,#103537,#103538,#103539,#103540,
#103541,#103542,#103543,#103544,#103545,#103546,#103547,#103548,#103549),
 .UNSPECIFIED.,.F.,.F.,(4,2,2,2,2,2,4),(-0.000236619803559426,0.,0.00609779134674399,
0.0119337102428204,0.0183998186375428,0.0234029027745216,0.0278441972723019),
 .UNSPECIFIED.) ;
#1446=B_SPLINE_CURVE_WITH_KNOTS('',3,(#103555,#103556,#103557,#103558,#103559,
#103560,#103561,#103562,#103563,#103564,#103565,#103566,#103567,#103568),
 .UNSPECIFIED.,.F.,.F.,(4,2,2,2,2,2,4),(-0.0559250143520313,-0.0556883945484605,
-0.0495906032013131,-0.0437546843047777,-0.037288575909542,-0.0322854917721873,
-0.0278441972740755),.UNSPECIFIED.) ;
#1447=B_SPLINE_CURVE_WITH_KNOTS('',3,(#103574,#103575,#103576,#103577,#103578,
#103579,#103580,#103581,#103582,#103583,#103584,#103585,#103586,#103587,
#103588,#103589),.UNSPECIFIED.,.F.,.F.,(4,3,3,3,3,4),(-0.000437598556142791,
0.,0.00562170475737048,0.011482325161532,0.0173413775096432,0.0231997078505159),
 .UNSPECIFIED.) ;
#1448=B_SPLINE_CURVE_WITH_KNOTS('',3,(#103595,#103596,#103597,#103598,#103599,
#103600,#103601,#103602,#103603,#103604,#103605,#103606,#103607,#103608,
#103609,#103610),.UNSPECIFIED.,.F.,.F.,(4,3,3,3,3,4),(-0.046837014256793,
-0.0463994157012118,-0.0407777109438107,-0.0349170905396121,-0.0290580381914533,
-0.0231997078505249),.UNSPECIFIED.) ;
#1449=B_SPLINE_CURVE_WITH_KNOTS('',3,(#104026,#104027,#104028,#104029,#104030,
#104031,#104032,#104033,#104034,#104035,#104036,#104037,#104038,#104039),
 .UNSPECIFIED.,.F.,.F.,(4,2,2,2,2,2,4),(-0.0559250143525619,-0.0556883945479474,
-0.0495906032011524,-0.0437546843048812,-0.037288575909754,-0.0322854917724513,
-0.027844197274366),.UNSPECIFIED.) ;
#1450=B_SPLINE_CURVE_WITH_KNOTS('',3,(#104042,#104043,#104044,#104045,#104046,
#104047,#104048,#104049,#104050,#104051,#104052,#104053,#104054,#104055),
 .UNSPECIFIED.,.F.,.F.,(4,2,2,2,2,2,4),(-0.000236619803144863,0.,0.00609779134711087,
0.0119337102436339,0.0183998186386153,0.0234029027758149,0.0278441972738027),
 .UNSPECIFIED.) ;
#1451=B_SPLINE_CURVE_WITH_KNOTS('',3,(#104058,#104059,#104060,#104061,#104062,
#104063,#104064,#104065,#104066,#104067,#104068,#104069,#104070,#104071,
#104072,#104073),.UNSPECIFIED.,.F.,.F.,(4,3,3,3,3,4),(-0.000437598556136612,
0.,0.00562170475739987,0.0114823251615695,0.0173413775096577,0.0231997078505359),
 .UNSPECIFIED.) ;
#1452=B_SPLINE_CURVE_WITH_KNOTS('',3,(#104078,#104079,#104080,#104081,#104082,
#104083,#104084,#104085,#104086,#104087,#104088,#104089,#104090,#104091,
#104092,#104093),.UNSPECIFIED.,.F.,.F.,(4,3,3,3,3,4),(0.,0.00585824217054478,
0.0117172063374487,0.0175777385368331,0.0231993586852603,0.0236369506553383),
 .UNSPECIFIED.) ;
#1453=B_SPLINE_CURVE_WITH_KNOTS('',3,(#104095,#104096,#104097,#104098,#104099,
#104100,#104101,#104102,#104103,#104104,#104105,#104106,#104107,#104108),
 .UNSPECIFIED.,.F.,.F.,(4,2,2,2,2,2,4),(-0.000236619803563006,0.,0.00609779134689459,
0.0119337102432047,0.0183998186381472,0.0234029027752928,0.027844197273235),
 .UNSPECIFIED.) ;
#1454=B_SPLINE_CURVE_WITH_KNOTS('',3,(#104111,#104112,#104113,#104114,#104115,
#104116,#104117,#104118,#104119,#104120,#104121,#104122,#104123,#104124,
#104125,#104126),.UNSPECIFIED.,.F.,.F.,(4,3,3,3,3,4),(0.,0.00585824217054169,
0.0117172063374197,0.0175777385367584,0.0231993586851914,0.0236369506552836),
 .UNSPECIFIED.) ;
#1455=B_SPLINE_CURVE_WITH_KNOTS('',3,(#104128,#104129,#104130,#104131,#104132,
#104133,#104134,#104135,#104136,#104137,#104138,#104139,#104140,#104141),
 .UNSPECIFIED.,.F.,.F.,(4,2,2,2,2,2,4),(-0.055925014352618,-0.0556883945495578,
-0.049590603202043,-0.0437546843051378,-0.0372885759097438,-0.032285491772261,
-0.0278441972740487),.UNSPECIFIED.) ;
#1456=B_SPLINE_CURVE_WITH_KNOTS('',3,(#104143,#104144,#104145,#104146,#104147,
#104148,#104149,#104150,#104151,#104152,#104153,#104154,#104155,#104156,
#104157,#104158),.UNSPECIFIED.,.F.,.F.,(4,3,3,3,3,4),(-0.000437598556173687,
0.,0.00562170475743059,0.0114823251616519,0.0173413775098334,0.0231997078507846),
 .UNSPECIFIED.) ;
#1457=B_SPLINE_CURVE_WITH_KNOTS('',3,(#104163,#104164,#104165,#104166,#104167,
#104168,#104169,#104170,#104171,#104172,#104173,#104174,#104175,#104176,
#104177,#104178),.UNSPECIFIED.,.F.,.F.,(4,3,3,3,3,4),(0.,0.0058582421705496,
0.0117172063374621,0.01757773853685,0.0231993586852295,0.0236369506553315),
 .UNSPECIFIED.) ;
#1458=B_SPLINE_CURVE_WITH_KNOTS('',3,(#104179,#104180,#104181,#104182,#104183,
#104184,#104185,#104186,#104187,#104188,#104189,#104190,#104191,#104192),
 .UNSPECIFIED.,.F.,.F.,(4,2,2,2,2,2,4),(-0.000236619803562956,0.,0.00609779134697842,
0.0119337102433575,0.0183998186383507,0.0234029027755715,0.027844197273593),
 .UNSPECIFIED.) ;
#1459=B_SPLINE_CURVE_WITH_KNOTS('',3,(#104194,#104195,#104196,#104197,#104198,
#104199,#104200,#104201,#104202,#104203,#104204,#104205,#104206,#104207),
 .UNSPECIFIED.,.F.,.F.,(4,2,2,2,2,2,4),(-0.00023661980356627,0.,0.0060977913470113,
0.0119337102434447,0.0183998186385308,0.0234029027758003,0.027844197273845),
 .UNSPECIFIED.) ;
#1460=B_SPLINE_CURVE_WITH_KNOTS('',3,(#104208,#104209,#104210,#104211,#104212,
#104213,#104214,#104215,#104216,#104217,#104218,#104219,#104220,#104221,
#104222,#104223),.UNSPECIFIED.,.F.,.F.,(4,3,3,3,3,4),(0.,0.00585824217053873,
0.0117172063374278,0.0175777385368055,0.023199358685178,0.0236369506552736),
 .UNSPECIFIED.) ;
#1461=B_SPLINE_CURVE_WITH_KNOTS('',3,(#104225,#104226,#104227,#104228,#104229,
#104230,#104231,#104232,#104233,#104234,#104235,#104236,#104237,#104238),
 .UNSPECIFIED.,.F.,.F.,(4,2,2,2,2,2,4),(-0.055925014347253,-0.0556883945436994,
-0.0495906031970911,-0.0437546843011451,-0.0372885759065727,-0.0322854917697116,
-0.0278441972720297),.UNSPECIFIED.) ;
#1462=B_SPLINE_CURVE_WITH_KNOTS('',3,(#104240,#104241,#104242,#104243,#104244,
#104245,#104246,#104247,#104248,#104249,#104250,#104251,#104252,#104253,
#104254,#104255),.UNSPECIFIED.,.F.,.F.,(4,3,3,3,3,4),(-0.000437598556065294,
0.,0.00562170475696129,0.0114823251605729,0.0173413775081186,0.0231997078484631),
 .UNSPECIFIED.) ;
#1463=B_SPLINE_CURVE_WITH_KNOTS('',3,(#104260,#104261,#104262,#104263,#104264,
#104265,#104266,#104267,#104268,#104269,#104270,#104271,#104272,#104273,
#104274,#104275),.UNSPECIFIED.,.F.,.F.,(4,3,3,3,3,4),(0.,0.00585824217053423,
0.0117172063374038,0.0175777385367393,0.0231993586850723,0.0236369506551701),
 .UNSPECIFIED.) ;
#1464=B_SPLINE_CURVE_WITH_KNOTS('',3,(#104276,#104277,#104278,#104279,#104280,
#104281,#104282,#104283,#104284,#104285,#104286,#104287,#104288,#104289),
 .UNSPECIFIED.,.F.,.F.,(4,2,2,2,2,2,4),(-0.00023661980315042,0.,0.00609779134723154,
0.0119337102438925,0.0183998186390206,0.0234029027763186,0.027844197274388),
 .UNSPECIFIED.) ;
#1465=B_SPLINE_CURVE_WITH_KNOTS('',3,(#104291,#104292,#104293,#104294,#104295,
#104296,#104297,#104298,#104299,#104300,#104301,#104302,#104303,#104304),
 .UNSPECIFIED.,.F.,.F.,(4,2,2,2,2,2,4),(-0.000236619803568179,0.,0.00609779134706943,
0.011933710243561,0.0183998186387449,0.0234029027760718,0.0278441972741583),
 .UNSPECIFIED.) ;
#1466=B_SPLINE_CURVE_WITH_KNOTS('',3,(#104305,#104306,#104307,#104308,#104309,
#104310,#104311,#104312,#104313,#104314,#104315,#104316,#104317,#104318,
#104319,#104320),.UNSPECIFIED.,.F.,.F.,(4,3,3,3,3,4),(0.,0.00585824217054849,
0.0117172063374606,0.0175777385368388,0.0231993586852149,0.0236369506553345),
 .UNSPECIFIED.) ;
#1467=B_SPLINE_CURVE_WITH_KNOTS('',3,(#104322,#104323,#104324,#104325,#104326,
#104327,#104328,#104329,#104330,#104331,#104332,#104333,#104334,#104335),
 .UNSPECIFIED.,.F.,.F.,(4,2,2,2,2,2,4),(-0.0559250143497057,-0.0556883945461452,
-0.0495906031993172,-0.0437546843030612,-0.0372885759081806,-0.0322854917710824,
-0.0278441972731839),.UNSPECIFIED.) ;
#1468=B_SPLINE_CURVE_WITH_KNOTS('',3,(#104337,#104338,#104339,#104340,#104341,
#104342,#104343,#104344,#104345,#104346,#104347,#104348,#104349,#104350,
#104351,#104352),.UNSPECIFIED.,.F.,.F.,(4,3,3,3,3,4),(-0.000437598556084839,
0.,0.00562170475699754,0.0114823251606981,0.0173413775083502,0.0231997078487964),
 .UNSPECIFIED.) ;
#1469=B_SPLINE_CURVE_WITH_KNOTS('',3,(#104357,#104358,#104359,#104360,#104361,
#104362,#104363,#104364,#104365,#104366,#104367,#104368,#104369,#104370,
#104371,#104372),.UNSPECIFIED.,.F.,.F.,(4,3,3,3,3,4),(0.,0.00585824217054277,
0.0117172063374441,0.0175777385368182,0.0231993586851572,0.0236369506552668),
 .UNSPECIFIED.) ;
#1470=B_SPLINE_CURVE_WITH_KNOTS('',3,(#104373,#104374,#104375,#104376,#104377,
#104378,#104379,#104380,#104381,#104382,#104383,#104384,#104385,#104386),
 .UNSPECIFIED.,.F.,.F.,(4,2,2,2,2,2,4),(-0.00023661980356187,0.,0.00609779134698056,
0.0119337102433812,0.0183998186384326,0.0234029027756759,0.0278441972736905),
 .UNSPECIFIED.) ;
#1471=B_SPLINE_CURVE_WITH_KNOTS('',3,(#104388,#104389,#104390,#104391,#104392,
#104393,#104394,#104395,#104396,#104397,#104398,#104399,#104400,#104401),
 .UNSPECIFIED.,.F.,.F.,(4,2,2,2,2,2,4),(-0.000236619803566785,0.,0.00609779134702904,
0.0119337102434475,0.0183998186384865,0.0234029027757207,0.0278441972737459),
 .UNSPECIFIED.) ;
#1472=B_SPLINE_CURVE_WITH_KNOTS('',3,(#104402,#104403,#104404,#104405,#104406,
#104407,#104408,#104409,#104410,#104411,#104412,#104413,#104414,#104415,
#104416,#104417),.UNSPECIFIED.,.F.,.F.,(4,3,3,3,3,4),(0.,0.00585824217054034,
0.0117172063374279,0.0175777385367946,0.0231993586851777,0.0236369506552812),
 .UNSPECIFIED.) ;
#1473=B_SPLINE_CURVE_WITH_KNOTS('',3,(#104419,#104420,#104421,#104422,#104423,
#104424,#104425,#104426,#104427,#104428,#104429,#104430,#104431,#104432),
 .UNSPECIFIED.,.F.,.F.,(4,2,2,2,2,2,4),(-0.0559250143501053,-0.0556883945465432,
-0.0495906031996281,-0.0437546843033128,-0.0372885759083777,-0.0322854917712189,
-0.0278441972732712),.UNSPECIFIED.) ;
#1474=B_SPLINE_CURVE_WITH_KNOTS('',3,(#104434,#104435,#104436,#104437,#104438,
#104439,#104440,#104441,#104442,#104443,#104444,#104445,#104446,#104447,
#104448,#104449),.UNSPECIFIED.,.F.,.F.,(4,3,3,3,3,4),(-0.000437598556096447,
0.,0.00562170475713416,0.0114823251609764,0.0173413775087778,0.0231997078493695),
 .UNSPECIFIED.) ;
#1475=B_SPLINE_CURVE_WITH_KNOTS('',3,(#104454,#104455,#104456,#104457,#104458,
#104459,#104460,#104461,#104462,#104463,#104464,#104465,#104466,#104467,
#104468,#104469),.UNSPECIFIED.,.F.,.F.,(4,3,3,3,3,4),(0.,0.00585824217053087,
0.0117172063373846,0.0175777385366825,0.0231993586850888,0.0236369506551764),
 .UNSPECIFIED.) ;
#1476=B_SPLINE_CURVE_WITH_KNOTS('',3,(#104470,#104471,#104472,#104473,#104474,
#104475,#104476,#104477,#104478,#104479,#104480,#104481,#104482,#104483),
 .UNSPECIFIED.,.F.,.F.,(4,2,2,2,2,2,4),(-0.000236619803975554,0.,0.00609779134645292,
0.0119337102422305,0.0183998186368445,0.0234029027737468,0.0278441972714777),
 .UNSPECIFIED.) ;
#1477=B_SPLINE_CURVE_WITH_KNOTS('',3,(#104485,#104486,#104487,#104488,#104489,
#104490,#104491,#104492,#104493,#104494,#104495,#104496,#104497,#104498),
 .UNSPECIFIED.,.F.,.F.,(4,2,2,2,2,2,4),(-0.000236619803145561,0.,0.00609779134719067,
0.0119337102437602,0.0183998186387406,0.0234029027759312,0.0278441972739105),
 .UNSPECIFIED.) ;
#1478=B_SPLINE_CURVE_WITH_KNOTS('',3,(#104499,#104500,#104501,#104502,#104503,
#104504,#104505,#104506,#104507,#104508,#104509,#104510,#104511,#104512,
#104513,#104514),.UNSPECIFIED.,.F.,.F.,(4,3,3,3,3,4),(0.,0.00585824217053935,
0.0117172063374137,0.0175777385367471,0.0231993586851797,0.0236369506552624),
 .UNSPECIFIED.) ;
#1479=B_SPLINE_CURVE_WITH_KNOTS('',3,(#104516,#104517,#104518,#104519,#104520,
#104521,#104522,#104523,#104524,#104525,#104526,#104527,#104528,#104529),
 .UNSPECIFIED.,.F.,.F.,(4,2,2,2,2,2,4),(-0.0559250143516561,-0.0556883945480848,
-0.0495906032009887,-0.0437546843044866,-0.0372885759093485,-0.032285491772039,
-0.0278441972739555),.UNSPECIFIED.) ;
#1480=B_SPLINE_CURVE_WITH_KNOTS('',3,(#104531,#104532,#104533,#104534,#104535,
#104536,#104537,#104538,#104539,#104540,#104541,#104542,#104543,#104544,
#104545,#104546),.UNSPECIFIED.,.F.,.F.,(4,3,3,3,3,4),(-0.000437598556137922,
0.,0.00562170475738925,0.0114823251615342,0.0173413775096173,0.0231997078504894),
 .UNSPECIFIED.) ;
#1481=B_SPLINE_CURVE_WITH_KNOTS('',3,(#104551,#104552,#104553,#104554,#104555,
#104556,#104557,#104558,#104559,#104560,#104561,#104562,#104563,#104564,
#104565,#104566),.UNSPECIFIED.,.F.,.F.,(4,3,3,3,3,4),(0.,0.00585824217054286,
0.0117172063374258,0.0175777385367681,0.0231993586851975,0.0236369506552776),
 .UNSPECIFIED.) ;
#1482=B_SPLINE_CURVE_WITH_KNOTS('',3,(#104567,#104568,#104569,#104570,#104571,
#104572,#104573,#104574,#104575,#104576,#104577,#104578,#104579,#104580),
 .UNSPECIFIED.,.F.,.F.,(4,2,2,2,2,2,4),(-0.000236619803141347,0.,0.00609779134719742,
0.0119337102437761,0.0183998186387667,0.0234029027759622,0.0278441972739489),
 .UNSPECIFIED.) ;
#1483=B_SPLINE_CURVE_WITH_KNOTS('',3,(#104582,#104583,#104584,#104585,#104586,
#104587,#104588,#104589,#104590,#104591,#104592,#104593,#104594,#104595),
 .UNSPECIFIED.,.F.,.F.,(4,2,2,2,2,2,4),(-0.000236619803560324,0.,0.00609779134688203,
0.0119337102431469,0.0183998186380461,0.0234029027751694,0.0278441972730812),
 .UNSPECIFIED.) ;
#1484=B_SPLINE_CURVE_WITH_KNOTS('',3,(#104596,#104597,#104598,#104599,#104600,
#104601,#104602,#104603,#104604,#104605,#104606,#104607,#104608,#104609,
#104610,#104611),.UNSPECIFIED.,.F.,.F.,(4,3,3,3,3,4),(0.,0.00585824217053624,
0.0117172063373978,0.017577738536714,0.0231993586851339,0.0236369506552253),
 .UNSPECIFIED.) ;
#1485=B_SPLINE_CURVE_WITH_KNOTS('',3,(#104613,#104614,#104615,#104616,#104617,
#104618,#104619,#104620,#104621,#104622,#104623,#104624,#104625,#104626),
 .UNSPECIFIED.,.F.,.F.,(4,2,2,2,2,2,4),(-0.0559250143527569,-0.0556883945491825,
-0.0495906032019952,-0.0437546843053732,-0.0372885759100185,-0.0322854917725816,
-0.0278441972744026),.UNSPECIFIED.) ;
#1486=B_SPLINE_CURVE_WITH_KNOTS('',3,(#104628,#104629,#104630,#104631,#104632,
#104633,#104634,#104635,#104636,#104637,#104638,#104639,#104640,#104641,
#104642,#104643),.UNSPECIFIED.,.F.,.F.,(4,3,3,3,3,4),(-0.000437598556170072,
0.,0.00562170475739005,0.0114823251615356,0.0173413775096278,0.0231997078504878),
 .UNSPECIFIED.) ;
#1487=B_SPLINE_CURVE_WITH_KNOTS('',3,(#104648,#104649,#104650,#104651,#104652,
#104653,#104654,#104655,#104656,#104657,#104658,#104659,#104660,#104661,
#104662,#104663),.UNSPECIFIED.,.F.,.F.,(4,3,3,3,3,4),(0.,0.00585824217054469,
0.0117172063374513,0.0175777385368039,0.0231993586851361,0.0236369506553527),
 .UNSPECIFIED.) ;
#1488=B_SPLINE_CURVE_WITH_KNOTS('',3,(#104664,#104665,#104666,#104667,#104668,
#104669,#104670,#104671,#104672,#104673,#104674,#104675,#104676,#104677),
 .UNSPECIFIED.,.F.,.F.,(4,2,2,2,2,2,4),(-0.000236619804202799,0.,0.00609779134737763,
0.0119337102442503,0.0183998186398358,0.0234029027774637,0.0278441972757869),
 .UNSPECIFIED.) ;
#1489=B_SPLINE_CURVE_WITH_KNOTS('',3,(#104679,#104680,#104681,#104682,#104683,
#104684,#104685,#104686,#104687,#104688,#104689,#104690,#104691,#104692),
 .UNSPECIFIED.,.F.,.F.,(4,2,2,2,2,2,4),(-0.0002366198042002,0.,0.00609779134724177,
0.0119337102439773,0.0183998186394422,0.0234029027769713,0.027844197275244),
 .UNSPECIFIED.) ;
#1490=B_SPLINE_CURVE_WITH_KNOTS('',3,(#104693,#104694,#104695,#104696,#104697,
#104698,#104699,#104700,#104701,#104702,#104703,#104704,#104705,#104706,
#104707,#104708),.UNSPECIFIED.,.F.,.F.,(4,3,3,3,3,4),(0.,0.00585824217054219,
0.0117172063374448,0.0175777385367976,0.0231993586850719,0.0236369506552122),
 .UNSPECIFIED.) ;
#1491=B_SPLINE_CURVE_WITH_KNOTS('',3,(#104710,#104711,#104712,#104713,#104714,
#104715,#104716,#104717,#104718,#104719,#104720,#104721,#104722,#104723),
 .UNSPECIFIED.,.F.,.F.,(4,2,2,2,2,2,4),(-0.0559250143475747,-0.0556883945440193,
-0.0495906031973805,-0.0437546843014019,-0.0372885759067931,-0.0322854917699036,
-0.0278441972721905),.UNSPECIFIED.) ;
#1492=B_SPLINE_CURVE_WITH_KNOTS('',3,(#104725,#104726,#104727,#104728,#104729,
#104730,#104731,#104732,#104733,#104734,#104735,#104736,#104737,#104738,
#104739,#104740),.UNSPECIFIED.,.F.,.F.,(4,3,3,3,3,4),(-0.000437598556074084,
0.,0.00562170475694653,0.0114823251605845,0.0173413775081531,0.0231997078485162),
 .UNSPECIFIED.) ;
#1493=B_SPLINE_CURVE_WITH_KNOTS('',3,(#104745,#104746,#104747,#104748,#104749,
#104750,#104751,#104752,#104753,#104754,#104755,#104756,#104757,#104758,
#104759,#104760),.UNSPECIFIED.,.F.,.F.,(4,3,3,3,3,4),(0.,0.00585824217053932,
0.0117172063374163,0.0175777385367554,0.0231993586851953,0.0236369506552652),
 .UNSPECIFIED.) ;
#1494=B_SPLINE_CURVE_WITH_KNOTS('',3,(#104761,#104762,#104763,#104764,#104765,
#104766,#104767,#104768,#104769,#104770,#104771,#104772,#104773,#104774),
 .UNSPECIFIED.,.F.,.F.,(4,2,2,2,2,2,4),(-0.000236619803563584,0.,0.00609779134684538,
0.0119337102430664,0.0183998186379667,0.0234029027750871,0.0278441972729952),
 .UNSPECIFIED.) ;
#1495=B_SPLINE_CURVE_WITH_KNOTS('',3,(#104776,#104777,#104778,#104779,#104780,
#104781,#104782,#104783,#104784,#104785,#104786,#104787,#104788,#104789),
 .UNSPECIFIED.,.F.,.F.,(4,2,2,2,2,2,4),(-0.000236619803559064,0.,0.00609779134682761,
0.0119337102430243,0.0183998186378634,0.0234029027749327,0.0278441972727837),
 .UNSPECIFIED.) ;
#1496=B_SPLINE_CURVE_WITH_KNOTS('',3,(#104790,#104791,#104792,#104793,#104794,
#104795,#104796,#104797,#104798,#104799,#104800,#104801,#104802,#104803,
#104804,#104805),.UNSPECIFIED.,.F.,.F.,(4,3,3,3,3,4),(0.,0.00585824217053403,
0.0117172063373908,0.0175777385367026,0.0231993586851274,0.0236369506551984),
 .UNSPECIFIED.) ;
#1497=B_SPLINE_CURVE_WITH_KNOTS('',3,(#104807,#104808,#104809,#104810,#104811,
#104812,#104813,#104814,#104815,#104816,#104817,#104818,#104819,#104820),
 .UNSPECIFIED.,.F.,.F.,(4,2,2,2,2,2,4),(-0.0559250143495183,-0.0556883945459582,
-0.0495906031991357,-0.0437546843029003,-0.0372885759080418,-0.0322854917709563,
-0.0278441972730646),.UNSPECIFIED.) ;
#1498=B_SPLINE_CURVE_WITH_KNOTS('',3,(#104822,#104823,#104824,#104825,#104826,
#104827,#104828,#104829,#104830,#104831,#104832,#104833,#104834,#104835,
#104836,#104837),.UNSPECIFIED.,.F.,.F.,(4,3,3,3,3,4),(-0.000437598556092783,
0.,0.00562170475708721,0.0114823251608936,0.0173413775086511,0.0231997078492032),
 .UNSPECIFIED.) ;
#1499=B_SPLINE_CURVE_WITH_KNOTS('',3,(#104842,#104843,#104844,#104845,#104846,
#104847,#104848,#104849,#104850,#104851,#104852,#104853,#104854,#104855,
#104856,#104857),.UNSPECIFIED.,.F.,.F.,(4,3,3,3,3,4),(0.,0.00585824217054838,
0.0117172063374519,0.0175777385368119,0.0231993586852536,0.0236369506553148),
 .UNSPECIFIED.) ;
#1500=B_SPLINE_CURVE_WITH_KNOTS('',3,(#104858,#104859,#104860,#104861,#104862,
#104863,#104864,#104865,#104866,#104867,#104868,#104869,#104870,#104871),
 .UNSPECIFIED.,.F.,.F.,(4,2,2,2,2,2,4),(-0.000236619803558096,0.,0.00609779134681664,
0.0119337102430081,0.0183998186378316,0.0234029027748886,0.0278441972727373),
 .UNSPECIFIED.) ;
#1501=B_SPLINE_CURVE_WITH_KNOTS('',3,(#104873,#104874,#104875,#104876,#104877,
#104878,#104879,#104880,#104881,#104882,#104883,#104884,#104885,#104886),
 .UNSPECIFIED.,.F.,.F.,(4,2,2,2,2,2,4),(-0.000236619803562333,0.,0.00609779134692135,
0.0119337102432951,0.0183998186383094,0.0234029027755172,0.0278441972735094),
 .UNSPECIFIED.) ;
#1502=B_SPLINE_CURVE_WITH_KNOTS('',3,(#104887,#104888,#104889,#104890,#104891,
#104892,#104893,#104894,#104895,#104896,#104897,#104898,#104899,#104900,
#104901,#104902),.UNSPECIFIED.,.F.,.F.,(4,3,3,3,3,4),(0.,0.00585824217054129,
0.0117172063374373,0.0175777385368199,0.023199358685217,0.0236369506553186),
 .UNSPECIFIED.) ;
#1503=B_SPLINE_CURVE_WITH_KNOTS('',3,(#104904,#104905,#104906,#104907,#104908,
#104909,#104910,#104911,#104912,#104913,#104914,#104915,#104916,#104917),
 .UNSPECIFIED.,.F.,.F.,(4,2,2,2,2,2,4),(-0.0559250143502032,-0.0556883945466394,
-0.0495906031997328,-0.0437546843034414,-0.0372885759084786,-0.0322854917713055,
-0.0278441972733409),.UNSPECIFIED.) ;
#1504=B_SPLINE_CURVE_WITH_KNOTS('',3,(#104919,#104920,#104921,#104922,#104923,
#104924,#104925,#104926,#104927,#104928,#104929,#104930,#104931,#104932,
#104933,#104934),.UNSPECIFIED.,.F.,.F.,(4,3,3,3,3,4),(-0.000437598556094846,
0.,0.00562170475708876,0.0114823251608924,0.0173413775086073,0.0231997078491061),
 .UNSPECIFIED.) ;
#1505=B_SPLINE_CURVE_WITH_KNOTS('',3,(#104936,#104937,#104938,#104939,#104940,
#104941,#104942,#104943,#104944,#104945,#104946,#104947,#104948,#104949,
#104950,#104951),.UNSPECIFIED.,.F.,.F.,(4,3,3,3,3,4),(0.,0.00585824217053639,
0.0117172063374152,0.0175777385367772,0.0231993586851953,0.0236369506552933),
 .UNSPECIFIED.) ;
#1506=B_SPLINE_CURVE_WITH_KNOTS('',3,(#104952,#104953,#104954,#104955,#104956,
#104957,#104958,#104959,#104960,#104961,#104962,#104963,#104964,#104965),
 .UNSPECIFIED.,.F.,.F.,(4,2,2,2,2,2,4),(-0.000236619803922217,0.,0.00609779134654128,
0.0119337102425373,0.018399818637407,0.0234029027744858,0.0278441972723643),
 .UNSPECIFIED.) ;
#1507=B_SPLINE_CURVE_WITH_KNOTS('',3,(#104967,#104968,#104969,#104970,#104971,
#104972,#104973,#104974,#104975,#104976,#104977,#104978,#104979,#104980),
 .UNSPECIFIED.,.F.,.F.,(4,2,2,2,2,2,4),(-0.000236619803561269,0.,0.00609779134692068,
0.0119337102432194,0.0183998186381382,0.02340290277528,0.0278441972732167),
 .UNSPECIFIED.) ;
#1508=B_SPLINE_CURVE_WITH_KNOTS('',3,(#104981,#104982,#104983,#104984,#104985,
#104986,#104987,#104988,#104989,#104990,#104991,#104992,#104993,#104994,
#104995,#104996),.UNSPECIFIED.,.F.,.F.,(4,3,3,3,3,4),(0.,0.00585824217053491,
0.0117172063374156,0.0175777385367886,0.0231993586852222,0.0236369506553088),
 .UNSPECIFIED.) ;
#1509=B_SPLINE_CURVE_WITH_KNOTS('',3,(#104998,#104999,#105000,#105001,#105002,
#105003,#105004,#105005,#105006,#105007,#105008,#105009,#105010,#105011),
 .UNSPECIFIED.,.F.,.F.,(4,2,2,2,2,2,4),(-0.0559250143500672,-0.0556883945469228,
-0.049590603199785,-0.0437546843032336,-0.0372885759082228,-0.0322854917710044,
-0.0278441972729959),.UNSPECIFIED.) ;
#1510=B_SPLINE_CURVE_WITH_KNOTS('',3,(#105013,#105014,#105015,#105016,#105017,
#105018,#105019,#105020,#105021,#105022,#105023,#105024,#105025,#105026,
#105027,#105028),.UNSPECIFIED.,.F.,.F.,(4,3,3,3,3,4),(-0.000437598556138437,
0.,0.00562170475741228,0.0114823251616098,0.0173413775097521,0.0231997078506926),
 .UNSPECIFIED.) ;
#1511=B_SPLINE_CURVE_WITH_KNOTS('',3,(#105034,#105035,#105036,#105037,#105038,
#105039,#105040,#105041,#105042,#105043,#105044,#105045,#105046,#105047),
 .UNSPECIFIED.,.F.,.F.,(4,2,2,2,2,2,4),(-0.0559250143516994,-0.0556883945481287,
-0.0495906032010545,-0.0437546843045533,-0.0372885759093916,-0.0322854917720808,
-0.0278441972739919),.UNSPECIFIED.) ;
#1512=B_SPLINE_CURVE_WITH_KNOTS('',3,(#105051,#105052,#105053,#105054,#105055,
#105056,#105057,#105058,#105059,#105060,#105061,#105062,#105063,#105064,
#105065,#105066),.UNSPECIFIED.,.F.,.F.,(4,3,3,3,3,4),(-0.000437598556144422,
0.,0.00562170475740183,0.0114823251615895,0.0173413775097444,0.0231997078506806),
 .UNSPECIFIED.) ;
#1513=B_SPLINE_CURVE_WITH_KNOTS('',3,(#105073,#105074,#105075,#105076,#105077,
#105078,#105079,#105080,#105081,#105082,#105083,#105084,#105085,#105086),
 .UNSPECIFIED.,.F.,.F.,(4,2,2,2,2,2,4),(-0.0559250143435119,-0.0556883945403911,
-0.0495906031940201,-0.0437546842982849,-0.0372885759042276,-0.0322854917677294,
-0.0278441972703399),.UNSPECIFIED.) ;
#1514=B_SPLINE_CURVE_WITH_KNOTS('',3,(#105090,#105091,#105092,#105093,#105094,
#105095,#105096,#105097,#105098,#105099,#105100,#105101,#105102,#105103,
#105104,#105105),.UNSPECIFIED.,.F.,.F.,(4,3,3,3,3,4),(-0.000437598556018984,
0.,0.00562170475658728,0.0114823251597353,0.0173413775068133,0.0231997078467154),
 .UNSPECIFIED.) ;
#1515=B_SPLINE_CURVE_WITH_KNOTS('',3,(#105112,#105113,#105114,#105115,#105116,
#105117,#105118,#105119,#105120,#105121,#105122,#105123,#105124,#105125),
 .UNSPECIFIED.,.F.,.F.,(4,2,2,2,2,2,4),(-0.0559250143454541,-0.055688394541913,
-0.0495906031955341,-0.0437546842998321,-0.0372885759055476,-0.0322854917689083,
-0.0278441972713927),.UNSPECIFIED.) ;
#1516=B_SPLINE_CURVE_WITH_KNOTS('',3,(#105129,#105130,#105131,#105132,#105133,
#105134,#105135,#105136,#105137,#105138,#105139,#105140,#105141,#105142,
#105143,#105144),.UNSPECIFIED.,.F.,.F.,(4,3,3,3,3,4),(-0.000437598556040506,
0.,0.00562170475667276,0.0114823251599514,0.0173413775071961,0.0231997078472556),
 .UNSPECIFIED.) ;
#1517=B_SPLINE_CURVE_WITH_KNOTS('',3,(#105151,#105152,#105153,#105154,#105155,
#105156,#105157,#105158,#105159,#105160,#105161,#105162,#105163,#105164),
 .UNSPECIFIED.,.F.,.F.,(4,2,2,2,2,2,4),(-0.0559250143503411,-0.0556883945467744,
-0.0495906031998412,-0.0437546843035047,-0.0372885759085466,-0.0322854917713593,
-0.0278441972733858),.UNSPECIFIED.) ;
#1518=B_SPLINE_CURVE_WITH_KNOTS('',3,(#105168,#105169,#105170,#105171,#105172,
#105173,#105174,#105175,#105176,#105177,#105178,#105179,#105180,#105181,
#105182,#105183),.UNSPECIFIED.,.F.,.F.,(4,3,3,3,3,4),(-0.00043759855609295,
0.,0.00562170475705494,0.0114823251608269,0.0173413775085459,0.0231997078490585),
 .UNSPECIFIED.) ;
#1519=B_SPLINE_CURVE_WITH_KNOTS('',3,(#105190,#105191,#105192,#105193,#105194,
#105195,#105196,#105197,#105198,#105199,#105200,#105201,#105202,#105203),
 .UNSPECIFIED.,.F.,.F.,(4,2,2,2,2,2,4),(-0.0559250143576788,-0.0556883945534629,
-0.0495906032058708,-0.0437546843087237,-0.0372885759128067,-0.0322854917749087,
-0.027844197276348),.UNSPECIFIED.) ;
#1520=B_SPLINE_CURVE_WITH_KNOTS('',3,(#105207,#105208,#105209,#105210,#105211,
#105212,#105213,#105214,#105215,#105216,#105217,#105218,#105219,#105220,
#105221,#105222),.UNSPECIFIED.,.F.,.F.,(4,3,3,3,3,4),(-0.000437598556265556,
0.,0.00562170475766576,0.0114823251621366,0.0173413775105401,0.0231997078517073),
 .UNSPECIFIED.) ;
#1521=B_SPLINE_CURVE_WITH_KNOTS('',3,(#105229,#105230,#105231,#105232,#105233,
#105234,#105235,#105236,#105237,#105238,#105239,#105240,#105241,#105242),
 .UNSPECIFIED.,.F.,.F.,(4,2,2,2,2,2,4),(-0.0559250143546525,-0.0556883945504525,
-0.0495906032031384,-0.0437546843063546,-0.0372885759108327,-0.0322854917732639,
-0.0278441972749651),.UNSPECIFIED.) ;
#1522=B_SPLINE_CURVE_WITH_KNOTS('',3,(#105246,#105247,#105248,#105249,#105250,
#105251,#105252,#105253,#105254,#105255,#105256,#105257,#105258,#105259,
#105260,#105261),.UNSPECIFIED.,.F.,.F.,(4,3,3,3,3,4),(-0.000437598556211791,
0.,0.00562170475765983,0.011482325162167,0.0173413775106296,0.0231997078518591),
 .UNSPECIFIED.) ;
#1523=B_SPLINE_CURVE_WITH_KNOTS('',3,(#105268,#105269,#105270,#105271,#105272,
#105273,#105274,#105275,#105276,#105277,#105278,#105279,#105280,#105281),
 .UNSPECIFIED.,.F.,.F.,(4,2,2,2,2,2,4),(-0.0559250143563362,-0.055688394551709,
-0.0495906032045639,-0.0437546843078355,-0.0372885759121675,-0.0322854917744538,
-0.0278441972760254),.UNSPECIFIED.) ;
#1524=B_SPLINE_CURVE_WITH_KNOTS('',3,(#105285,#105286,#105287,#105288,#105289,
#105290,#105291,#105292,#105293,#105294,#105295,#105296,#105297,#105298,
#105299,#105300),.UNSPECIFIED.,.F.,.F.,(4,3,3,3,3,4),(-0.000437598556225459,
0.,0.00562170475744369,0.0114823251616755,0.0173413775098568,0.0231997078508077),
 .UNSPECIFIED.) ;
#1525=B_SPLINE_CURVE_WITH_KNOTS('',3,(#105307,#105308,#105309,#105310,#105311,
#105312,#105313,#105314,#105315,#105316,#105317,#105318,#105319,#105320),
 .UNSPECIFIED.,.F.,.F.,(4,2,2,2,2,2,4),(-0.0559250143492567,-0.0556883945456972,
-0.0495906031988905,-0.0437546843027083,-0.0372885759078583,-0.0322854917707879,
-0.0278441972729168),.UNSPECIFIED.) ;
#1526=B_SPLINE_CURVE_WITH_KNOTS('',3,(#105324,#105325,#105326,#105327,#105328,
#105329,#105330,#105331,#105332,#105333,#105334,#105335,#105336,#105337,
#105338,#105339),.UNSPECIFIED.,.F.,.F.,(4,3,3,3,3,4),(-0.000437598556080345,
0.,0.00562170475697672,0.0114823251606002,0.0173413775081636,0.0231997078485257),
 .UNSPECIFIED.) ;
#1527=B_SPLINE_CURVE_WITH_KNOTS('',3,(#105346,#105347,#105348,#105349,#105350,
#105351,#105352,#105353,#105354,#105355,#105356,#105357,#105358,#105359),
 .UNSPECIFIED.,.F.,.F.,(4,2,2,2,2,2,4),(-0.055925014349952,-0.0556883945463912,
-0.0495906031994983,-0.0437546843032064,-0.0372885759082967,-0.0322854917711481,
-0.0278441972731949),.UNSPECIFIED.) ;
#1528=B_SPLINE_CURVE_WITH_KNOTS('',3,(#105363,#105364,#105365,#105366,#105367,
#105368,#105369,#105370,#105371,#105372,#105373,#105374,#105375,#105376,
#105377,#105378),.UNSPECIFIED.,.F.,.F.,(4,3,3,3,3,4),(-0.000437598556096392,
0.,0.005621704757061,0.0114823251608164,0.0173413775085336,0.0231997078490434),
 .UNSPECIFIED.) ;
#2111=B_SPLINE_SURFACE_WITH_KNOTS('',3,3,((#101800,#101801,#101802,#101803,
#101804,#101805,#101806,#101807,#101808,#101809,#101810,#101811,#101812,
#101813,#101814,#101815),(#101816,#101817,#101818,#101819,#101820,#101821,
#101822,#101823,#101824,#101825,#101826,#101827,#101828,#101829,#101830,
#101831),(#101832,#101833,#101834,#101835,#101836,#101837,#101838,#101839,
#101840,#101841,#101842,#101843,#101844,#101845,#101846,#101847),(#101848,
#101849,#101850,#101851,#101852,#101853,#101854,#101855,#101856,#101857,
#101858,#101859,#101860,#101861,#101862,#101863),(#101864,#101865,#101866,
#101867,#101868,#101869,#101870,#101871,#101872,#101873,#101874,#101875,
#101876,#101877,#101878,#101879)),.UNSPECIFIED.,.F.,.T.,.F.,(4,1,4),(4,
1,1,1,1,1,1,1,1,1,1,1,1,4),(0.,0.5,1.),(-1.37470975898194,-1.17832265055595,
-0.981935542129957,-0.785548433703966,-0.589161325277974,-0.196387108425991,
0.,0.196387108425991,0.392774216851983,0.589161325277974,0.785548433703966,
0.981935542129957,1.17832265055595,1.37470975898194),.UNSPECIFIED.) ;
#2112=B_SPLINE_SURFACE_WITH_KNOTS('',3,3,((#101907,#101908,#101909,#101910,
#101911,#101912,#101913,#101914,#101915,#101916,#101917,#101918,#101919,
#101920,#101921,#101922),(#101923,#101924,#101925,#101926,#101927,#101928,
#101929,#101930,#101931,#101932,#101933,#101934,#101935,#101936,#101937,
#101938),(#101939,#101940,#101941,#101942,#101943,#101944,#101945,#101946,
#101947,#101948,#101949,#101950,#101951,#101952,#101953,#101954),(#101955,
#101956,#101957,#101958,#101959,#101960,#101961,#101962,#101963,#101964,
#101965,#101966,#101967,#101968,#101969,#101970),(#101971,#101972,#101973,
#101974,#101975,#101976,#101977,#101978,#101979,#101980,#101981,#101982,
#101983,#101984,#101985,#101986)),.UNSPECIFIED.,.F.,.T.,.F.,(4,1,4),(4,
1,1,1,1,1,1,1,1,1,1,1,1,4),(0.,0.5,1.),(-1.37470975898194,-1.17832265055595,
-0.981935542129957,-0.785548433703966,-0.589161325277974,-0.196387108425991,
0.,0.196387108425991,0.392774216851983,0.589161325277974,0.785548433703966,
0.981935542129957,1.17832265055595,1.37470975898194),.UNSPECIFIED.) ;
#2858=PLANE('',#54047) ;
#2859=PLANE('',#54052) ;
#2860=PLANE('',#54053) ;
#2861=PLANE('',#54055) ;
#2862=PLANE('',#54217) ;
#2863=PLANE('',#54220) ;
#2864=PLANE('',#54223) ;
#2865=PLANE('',#54226) ;
#2866=PLANE('',#54229) ;
#2867=PLANE('',#54232) ;
#2868=PLANE('',#54235) ;
#2869=PLANE('',#54238) ;
#2870=PLANE('',#54241) ;
#2871=PLANE('',#54244) ;
#2872=PLANE('',#54247) ;
#2873=PLANE('',#54250) ;
#2874=PLANE('',#54253) ;
#2875=PLANE('',#54256) ;
#2876=PLANE('',#54259) ;
#2877=PLANE('',#54262) ;
#2878=PLANE('',#54265) ;
#2879=PLANE('',#54268) ;
#2880=PLANE('',#54271) ;
#2881=PLANE('',#54274) ;
#2882=PLANE('',#54277) ;
#2883=PLANE('',#54279) ;
#2884=PLANE('',#54281) ;
#2885=PLANE('',#54283) ;
#2886=PLANE('',#54285) ;
#2887=PLANE('',#54287) ;
#2888=PLANE('',#54289) ;
#2889=PLANE('',#54291) ;
#2890=PLANE('',#54293) ;
#2891=PLANE('',#54295) ;
#2892=PLANE('',#54297) ;
#2893=PLANE('',#54299) ;
#2894=PLANE('',#54301) ;
#2895=PLANE('',#54303) ;
#2896=PLANE('',#54305) ;
#2897=PLANE('',#54307) ;
#2898=PLANE('',#54309) ;
#2899=PLANE('',#54311) ;
#2900=PLANE('',#54313) ;
#2901=PLANE('',#54319) ;
#2902=PLANE('',#54363) ;
#2903=PLANE('',#54365) ;
#2904=PLANE('',#54367) ;
#2905=PLANE('',#54369) ;
#2906=PLANE('',#54371) ;
#2907=PLANE('',#54373) ;
#2908=PLANE('',#54375) ;
#2909=PLANE('',#54377) ;
#2910=PLANE('',#54379) ;
#2911=PLANE('',#54381) ;
#2912=PLANE('',#54383) ;
#2913=PLANE('',#54385) ;
#2914=PLANE('',#54387) ;
#2915=PLANE('',#54389) ;
#2916=PLANE('',#54391) ;
#2917=PLANE('',#54393) ;
#2918=PLANE('',#54395) ;
#2919=PLANE('',#54397) ;
#2920=PLANE('',#54399) ;
#2921=PLANE('',#54401) ;
#2922=PLANE('',#54504) ;
#2923=PLANE('',#54506) ;
#2924=PLANE('',#54507) ;
#2925=PLANE('',#54508) ;
#2926=PLANE('',#54510) ;
#2927=PLANE('',#54511) ;
#2928=PLANE('',#54513) ;
#2929=PLANE('',#54514) ;
#2930=PLANE('',#54516) ;
#2931=PLANE('',#54517) ;
#2932=PLANE('',#54519) ;
#2933=PLANE('',#54520) ;
#2934=PLANE('',#54522) ;
#2935=PLANE('',#54523) ;
#2936=PLANE('',#54525) ;
#2937=PLANE('',#54526) ;
#2938=PLANE('',#54528) ;
#2939=PLANE('',#54529) ;
#2940=PLANE('',#54531) ;
#2941=PLANE('',#54532) ;
#5754=LINE('',#102051,#8968) ;
#5755=LINE('',#102069,#8969) ;
#5756=LINE('',#102093,#8970) ;
#5757=LINE('',#102109,#8971) ;
#5758=LINE('',#102131,#8972) ;
#5759=LINE('',#102149,#8973) ;
#5760=LINE('',#102173,#8974) ;
#5761=LINE('',#102189,#8975) ;
#5762=LINE('',#102211,#8976) ;
#5763=LINE('',#102229,#8977) ;
#5764=LINE('',#102253,#8978) ;
#5765=LINE('',#102269,#8979) ;
#5766=LINE('',#102291,#8980) ;
#5767=LINE('',#102309,#8981) ;
#5768=LINE('',#102333,#8982) ;
#5769=LINE('',#102349,#8983) ;
#5770=LINE('',#102371,#8984) ;
#5771=LINE('',#102389,#8985) ;
#5772=LINE('',#102413,#8986) ;
#5773=LINE('',#102429,#8987) ;
#5774=LINE('',#102451,#8988) ;
#5775=LINE('',#102469,#8989) ;
#5776=LINE('',#102493,#8990) ;
#5777=LINE('',#102509,#8991) ;
#5778=LINE('',#102531,#8992) ;
#5779=LINE('',#102549,#8993) ;
#5780=LINE('',#102573,#8994) ;
#5781=LINE('',#102589,#8995) ;
#5782=LINE('',#102611,#8996) ;
#5783=LINE('',#102629,#8997) ;
#5784=LINE('',#102653,#8998) ;
#5785=LINE('',#102669,#8999) ;
#5786=LINE('',#102691,#9000) ;
#5787=LINE('',#102709,#9001) ;
#5788=LINE('',#102733,#9002) ;
#5789=LINE('',#102749,#9003) ;
#5790=LINE('',#102771,#9004) ;
#5791=LINE('',#102789,#9005) ;
#5792=LINE('',#102813,#9006) ;
#5793=LINE('',#102829,#9007) ;
#5794=LINE('',#102851,#9008) ;
#5795=LINE('',#102853,#9009) ;
#5796=LINE('',#102893,#9010) ;
#5797=LINE('',#102895,#9011) ;
#5798=LINE('',#102931,#9012) ;
#5799=LINE('',#102933,#9013) ;
#5800=LINE('',#102973,#9014) ;
#5801=LINE('',#102975,#9015) ;
#5802=LINE('',#103011,#9016) ;
#5803=LINE('',#103013,#9017) ;
#5804=LINE('',#103053,#9018) ;
#5805=LINE('',#103055,#9019) ;
#5806=LINE('',#103091,#9020) ;
#5807=LINE('',#103093,#9021) ;
#5808=LINE('',#103133,#9022) ;
#5809=LINE('',#103135,#9023) ;
#5810=LINE('',#103171,#9024) ;
#5811=LINE('',#103173,#9025) ;
#5812=LINE('',#103213,#9026) ;
#5813=LINE('',#103215,#9027) ;
#5814=LINE('',#103251,#9028) ;
#5815=LINE('',#103253,#9029) ;
#5816=LINE('',#103293,#9030) ;
#5817=LINE('',#103295,#9031) ;
#5818=LINE('',#103331,#9032) ;
#5819=LINE('',#103333,#9033) ;
#5820=LINE('',#103373,#9034) ;
#5821=LINE('',#103375,#9035) ;
#5822=LINE('',#103411,#9036) ;
#5823=LINE('',#103413,#9037) ;
#5824=LINE('',#103453,#9038) ;
#5825=LINE('',#103455,#9039) ;
#5826=LINE('',#103491,#9040) ;
#5827=LINE('',#103493,#9041) ;
#5828=LINE('',#103533,#9042) ;
#5829=LINE('',#103535,#9043) ;
#5830=LINE('',#103571,#9044) ;
#5831=LINE('',#103573,#9045) ;
#5832=LINE('',#103612,#9046) ;
#5833=LINE('',#103613,#9047) ;
#5834=LINE('',#103616,#9048) ;
#5835=LINE('',#103618,#9049) ;
#5836=LINE('',#103619,#9050) ;
#5837=LINE('',#103622,#9051) ;
#5838=LINE('',#103626,#9052) ;
#5839=LINE('',#103627,#9053) ;
#5840=LINE('',#103630,#9054) ;
#5841=LINE('',#103634,#9055) ;
#5842=LINE('',#103635,#9056) ;
#5843=LINE('',#103638,#9057) ;
#5844=LINE('',#103642,#9058) ;
#5845=LINE('',#103643,#9059) ;
#5846=LINE('',#103646,#9060) ;
#5847=LINE('',#103650,#9061) ;
#5848=LINE('',#103651,#9062) ;
#5849=LINE('',#103654,#9063) ;
#5850=LINE('',#103658,#9064) ;
#5851=LINE('',#103659,#9065) ;
#5852=LINE('',#103662,#9066) ;
#5853=LINE('',#103666,#9067) ;
#5854=LINE('',#103667,#9068) ;
#5855=LINE('',#103670,#9069) ;
#5856=LINE('',#103674,#9070) ;
#5857=LINE('',#103675,#9071) ;
#5858=LINE('',#103678,#9072) ;
#5859=LINE('',#103682,#9073) ;
#5860=LINE('',#103683,#9074) ;
#5861=LINE('',#103686,#9075) ;
#5862=LINE('',#103690,#9076) ;
#5863=LINE('',#103691,#9077) ;
#5864=LINE('',#103694,#9078) ;
#5865=LINE('',#103698,#9079) ;
#5866=LINE('',#103699,#9080) ;
#5867=LINE('',#103702,#9081) ;
#5868=LINE('',#103706,#9082) ;
#5869=LINE('',#103707,#9083) ;
#5870=LINE('',#103710,#9084) ;
#5871=LINE('',#103714,#9085) ;
#5872=LINE('',#103715,#9086) ;
#5873=LINE('',#103718,#9087) ;
#5874=LINE('',#103722,#9088) ;
#5875=LINE('',#103723,#9089) ;
#5876=LINE('',#103726,#9090) ;
#5877=LINE('',#103730,#9091) ;
#5878=LINE('',#103731,#9092) ;
#5879=LINE('',#103734,#9093) ;
#5880=LINE('',#103738,#9094) ;
#5881=LINE('',#103739,#9095) ;
#5882=LINE('',#103742,#9096) ;
#5883=LINE('',#103746,#9097) ;
#5884=LINE('',#103747,#9098) ;
#5885=LINE('',#103750,#9099) ;
#5886=LINE('',#103754,#9100) ;
#5887=LINE('',#103755,#9101) ;
#5888=LINE('',#103758,#9102) ;
#5889=LINE('',#103762,#9103) ;
#5890=LINE('',#103763,#9104) ;
#5891=LINE('',#103766,#9105) ;
#5892=LINE('',#103770,#9106) ;
#5893=LINE('',#103771,#9107) ;
#5894=LINE('',#103774,#9108) ;
#5895=LINE('',#103906,#9109) ;
#5896=LINE('',#103909,#9110) ;
#5897=LINE('',#103912,#9111) ;
#5898=LINE('',#103915,#9112) ;
#5899=LINE('',#103918,#9113) ;
#5900=LINE('',#103921,#9114) ;
#5901=LINE('',#103924,#9115) ;
#5902=LINE('',#103927,#9116) ;
#5903=LINE('',#103930,#9117) ;
#5904=LINE('',#103933,#9118) ;
#5905=LINE('',#103936,#9119) ;
#5906=LINE('',#103939,#9120) ;
#5907=LINE('',#103942,#9121) ;
#5908=LINE('',#103945,#9122) ;
#5909=LINE('',#103948,#9123) ;
#5910=LINE('',#103951,#9124) ;
#5911=LINE('',#103954,#9125) ;
#5912=LINE('',#103957,#9126) ;
#5913=LINE('',#103960,#9127) ;
#5914=LINE('',#103963,#9128) ;
#5915=LINE('',#103966,#9129) ;
#5916=LINE('',#103969,#9130) ;
#5917=LINE('',#103972,#9131) ;
#5918=LINE('',#103975,#9132) ;
#5919=LINE('',#103978,#9133) ;
#5920=LINE('',#103981,#9134) ;
#5921=LINE('',#103984,#9135) ;
#5922=LINE('',#103987,#9136) ;
#5923=LINE('',#103990,#9137) ;
#5924=LINE('',#103993,#9138) ;
#5925=LINE('',#103996,#9139) ;
#5926=LINE('',#103999,#9140) ;
#5927=LINE('',#104002,#9141) ;
#5928=LINE('',#104005,#9142) ;
#5929=LINE('',#104008,#9143) ;
#5930=LINE('',#104011,#9144) ;
#5931=LINE('',#104014,#9145) ;
#5932=LINE('',#104017,#9146) ;
#5933=LINE('',#104020,#9147) ;
#5934=LINE('',#104023,#9148) ;
#5935=LINE('',#104074,#9149) ;
#5936=LINE('',#104077,#9150) ;
#5937=LINE('',#104110,#9151) ;
#5938=LINE('',#104162,#9152) ;
#5939=LINE('',#104259,#9153) ;
#5940=LINE('',#104356,#9154) ;
#5941=LINE('',#104453,#9155) ;
#5942=LINE('',#104550,#9156) ;
#5943=LINE('',#104647,#9157) ;
#5944=LINE('',#104744,#9158) ;
#5945=LINE('',#104841,#9159) ;
#5946=LINE('',#105050,#9160) ;
#5947=LINE('',#105089,#9161) ;
#5948=LINE('',#105128,#9162) ;
#5949=LINE('',#105167,#9163) ;
#5950=LINE('',#105206,#9164) ;
#5951=LINE('',#105245,#9165) ;
#5952=LINE('',#105284,#9166) ;
#5953=LINE('',#105323,#9167) ;
#5954=LINE('',#105362,#9168) ;
#5955=LINE('',#105384,#9169) ;
#5956=LINE('',#105385,#9170) ;
#5957=LINE('',#105387,#9171) ;
#5958=LINE('',#105389,#9172) ;
#5959=LINE('',#105392,#9173) ;
#5960=LINE('',#105393,#9174) ;
#5961=LINE('',#105395,#9175) ;
#5962=LINE('',#105396,#9176) ;
#5963=LINE('',#105399,#9177) ;
#5964=LINE('',#105400,#9178) ;
#5965=LINE('',#105402,#9179) ;
#5966=LINE('',#105403,#9180) ;
#5967=LINE('',#105406,#9181) ;
#5968=LINE('',#105407,#9182) ;
#5969=LINE('',#105409,#9183) ;
#5970=LINE('',#105410,#9184) ;
#5971=LINE('',#105413,#9185) ;
#5972=LINE('',#105414,#9186) ;
#5973=LINE('',#105416,#9187) ;
#5974=LINE('',#105417,#9188) ;
#5975=LINE('',#105420,#9189) ;
#5976=LINE('',#105421,#9190) ;
#5977=LINE('',#105423,#9191) ;
#5978=LINE('',#105424,#9192) ;
#5979=LINE('',#105427,#9193) ;
#5980=LINE('',#105428,#9194) ;
#5981=LINE('',#105430,#9195) ;
#5982=LINE('',#105431,#9196) ;
#5983=LINE('',#105434,#9197) ;
#5984=LINE('',#105435,#9198) ;
#5985=LINE('',#105437,#9199) ;
#5986=LINE('',#105438,#9200) ;
#5987=LINE('',#105441,#9201) ;
#5988=LINE('',#105442,#9202) ;
#5989=LINE('',#105444,#9203) ;
#5990=LINE('',#105445,#9204) ;
#5991=LINE('',#105448,#9205) ;
#5992=LINE('',#105449,#9206) ;
#5993=LINE('',#105451,#9207) ;
#5994=LINE('',#105463,#9208) ;
#8968=VECTOR('',#67321,10.) ;
#8969=VECTOR('',#67322,10.) ;
#8970=VECTOR('',#67331,10.) ;
#8971=VECTOR('',#67332,10.) ;
#8972=VECTOR('',#67341,10.) ;
#8973=VECTOR('',#67342,10.) ;
#8974=VECTOR('',#67351,10.) ;
#8975=VECTOR('',#67352,10.) ;
#8976=VECTOR('',#67361,10.) ;
#8977=VECTOR('',#67362,10.) ;
#8978=VECTOR('',#67371,10.) ;
#8979=VECTOR('',#67372,10.) ;
#8980=VECTOR('',#67381,10.) ;
#8981=VECTOR('',#67382,9.99999999999999) ;
#8982=VECTOR('',#67391,9.99999999999999) ;
#8983=VECTOR('',#67392,9.99999999999999) ;
#8984=VECTOR('',#67401,9.99999999999999) ;
#8985=VECTOR('',#67402,9.99999999999999) ;
#8986=VECTOR('',#67411,9.99999999999999) ;
#8987=VECTOR('',#67412,9.99999999999999) ;
#8988=VECTOR('',#67421,10.) ;
#8989=VECTOR('',#67422,10.) ;
#8990=VECTOR('',#67431,10.) ;
#8991=VECTOR('',#67432,10.) ;
#8992=VECTOR('',#67441,10.) ;
#8993=VECTOR('',#67442,10.) ;
#8994=VECTOR('',#67451,10.) ;
#8995=VECTOR('',#67452,10.) ;
#8996=VECTOR('',#67461,10.) ;
#8997=VECTOR('',#67462,10.) ;
#8998=VECTOR('',#67471,10.) ;
#8999=VECTOR('',#67472,10.) ;
#9000=VECTOR('',#67481,10.) ;
#9001=VECTOR('',#67482,10.) ;
#9002=VECTOR('',#67491,10.) ;
#9003=VECTOR('',#67492,10.) ;
#9004=VECTOR('',#67501,9.99999999999999) ;
#9005=VECTOR('',#67502,9.99999999999999) ;
#9006=VECTOR('',#67511,9.99999999999999) ;
#9007=VECTOR('',#67512,9.99999999999999) ;
#9008=VECTOR('',#67521,10.) ;
#9009=VECTOR('',#67522,10.) ;
#9010=VECTOR('',#67531,10.) ;
#9011=VECTOR('',#67532,10.) ;
#9012=VECTOR('',#67541,10.) ;
#9013=VECTOR('',#67542,10.) ;
#9014=VECTOR('',#67551,10.) ;
#9015=VECTOR('',#67552,10.) ;
#9016=VECTOR('',#67561,10.) ;
#9017=VECTOR('',#67562,10.) ;
#9018=VECTOR('',#67571,10.) ;
#9019=VECTOR('',#67572,10.) ;
#9020=VECTOR('',#67581,9.99999999999999) ;
#9021=VECTOR('',#67582,9.99999999999999) ;
#9022=VECTOR('',#67591,9.99999999999999) ;
#9023=VECTOR('',#67592,9.99999999999999) ;
#9024=VECTOR('',#67601,9.99999999999999) ;
#9025=VECTOR('',#67602,9.99999999999999) ;
#9026=VECTOR('',#67611,9.99999999999999) ;
#9027=VECTOR('',#67612,9.99999999999999) ;
#9028=VECTOR('',#67621,10.) ;
#9029=VECTOR('',#67622,10.) ;
#9030=VECTOR('',#67631,10.) ;
#9031=VECTOR('',#67632,10.) ;
#9032=VECTOR('',#67641,10.) ;
#9033=VECTOR('',#67642,10.) ;
#9034=VECTOR('',#67651,10.) ;
#9035=VECTOR('',#67652,10.) ;
#9036=VECTOR('',#67661,10.) ;
#9037=VECTOR('',#67662,10.) ;
#9038=VECTOR('',#67671,10.) ;
#9039=VECTOR('',#67672,10.) ;
#9040=VECTOR('',#67681,9.99999999999999) ;
#9041=VECTOR('',#67682,9.99999999999999) ;
#9042=VECTOR('',#67691,9.99999999999999) ;
#9043=VECTOR('',#67692,9.99999999999999) ;
#9044=VECTOR('',#67701,9.99999999999999) ;
#9045=VECTOR('',#67702,9.99999999999999) ;
#9046=VECTOR('',#67711,9.99999999999999) ;
#9047=VECTOR('',#67712,9.99999999999999) ;
#9048=VECTOR('',#67715,10.) ;
#9049=VECTOR('',#67716,10.) ;
#9050=VECTOR('',#67717,10.) ;
#9051=VECTOR('',#67720,10.) ;
#9052=VECTOR('',#67725,10.) ;
#9053=VECTOR('',#67726,10.) ;
#9054=VECTOR('',#67729,10.) ;
#9055=VECTOR('',#67734,10.) ;
#9056=VECTOR('',#67735,10.) ;
#9057=VECTOR('',#67738,10.) ;
#9058=VECTOR('',#67743,10.) ;
#9059=VECTOR('',#67744,10.) ;
#9060=VECTOR('',#67747,10.) ;
#9061=VECTOR('',#67752,10.) ;
#9062=VECTOR('',#67753,10.) ;
#9063=VECTOR('',#67756,10.) ;
#9064=VECTOR('',#67761,10.) ;
#9065=VECTOR('',#67762,10.) ;
#9066=VECTOR('',#67765,10.) ;
#9067=VECTOR('',#67770,10.) ;
#9068=VECTOR('',#67771,9.99999999999999) ;
#9069=VECTOR('',#67774,10.) ;
#9070=VECTOR('',#67779,10.) ;
#9071=VECTOR('',#67780,9.99999999999999) ;
#9072=VECTOR('',#67783,10.) ;
#9073=VECTOR('',#67788,10.) ;
#9074=VECTOR('',#67789,9.99999999999999) ;
#9075=VECTOR('',#67792,10.) ;
#9076=VECTOR('',#67797,10.) ;
#9077=VECTOR('',#67798,9.99999999999999) ;
#9078=VECTOR('',#67801,10.) ;
#9079=VECTOR('',#67806,10.) ;
#9080=VECTOR('',#67807,10.) ;
#9081=VECTOR('',#67810,10.) ;
#9082=VECTOR('',#67815,10.) ;
#9083=VECTOR('',#67816,10.) ;
#9084=VECTOR('',#67819,10.) ;
#9085=VECTOR('',#67824,10.) ;
#9086=VECTOR('',#67825,10.) ;
#9087=VECTOR('',#67828,10.) ;
#9088=VECTOR('',#67833,10.) ;
#9089=VECTOR('',#67834,10.) ;
#9090=VECTOR('',#67837,10.) ;
#9091=VECTOR('',#67842,10.) ;
#9092=VECTOR('',#67843,10.) ;
#9093=VECTOR('',#67846,10.) ;
#9094=VECTOR('',#67851,10.) ;
#9095=VECTOR('',#67852,10.) ;
#9096=VECTOR('',#67855,10.) ;
#9097=VECTOR('',#67860,10.) ;
#9098=VECTOR('',#67861,9.99999999999999) ;
#9099=VECTOR('',#67864,10.) ;
#9100=VECTOR('',#67869,10.) ;
#9101=VECTOR('',#67870,9.99999999999999) ;
#9102=VECTOR('',#67873,10.) ;
#9103=VECTOR('',#67878,10.) ;
#9104=VECTOR('',#67879,9.99999999999999) ;
#9105=VECTOR('',#67882,10.) ;
#9106=VECTOR('',#67887,10.) ;
#9107=VECTOR('',#67888,9.99999999999999) ;
#9108=VECTOR('',#67891,10.) ;
#9109=VECTOR('',#68068,10.) ;
#9110=VECTOR('',#68071,10.) ;
#9111=VECTOR('',#68074,9.99999999999999) ;
#9112=VECTOR('',#68077,9.99999999999999) ;
#9113=VECTOR('',#68080,10.) ;
#9114=VECTOR('',#68083,10.) ;
#9115=VECTOR('',#68086,10.) ;
#9116=VECTOR('',#68089,10.) ;
#9117=VECTOR('',#68092,10.) ;
#9118=VECTOR('',#68095,10.) ;
#9119=VECTOR('',#68098,10.) ;
#9120=VECTOR('',#68101,10.) ;
#9121=VECTOR('',#68104,9.99999999999999) ;
#9122=VECTOR('',#68107,9.99999999999999) ;
#9123=VECTOR('',#68110,9.99999999999999) ;
#9124=VECTOR('',#68113,9.99999999999999) ;
#9125=VECTOR('',#68116,10.) ;
#9126=VECTOR('',#68119,10.) ;
#9127=VECTOR('',#68122,10.) ;
#9128=VECTOR('',#68125,10.) ;
#9129=VECTOR('',#68128,10.) ;
#9130=VECTOR('',#68131,10.) ;
#9131=VECTOR('',#68134,9.99999999999999) ;
#9132=VECTOR('',#68137,9.99999999999999) ;
#9133=VECTOR('',#68140,9.99999999999999) ;
#9134=VECTOR('',#68143,9.99999999999999) ;
#9135=VECTOR('',#68146,10.) ;
#9136=VECTOR('',#68149,10.) ;
#9137=VECTOR('',#68152,10.) ;
#9138=VECTOR('',#68155,10.) ;
#9139=VECTOR('',#68158,10.) ;
#9140=VECTOR('',#68161,10.) ;
#9141=VECTOR('',#68164,9.99999999999999) ;
#9142=VECTOR('',#68167,9.99999999999999) ;
#9143=VECTOR('',#68170,9.99999999999999) ;
#9144=VECTOR('',#68173,9.99999999999999) ;
#9145=VECTOR('',#68176,10.) ;
#9146=VECTOR('',#68179,10.) ;
#9147=VECTOR('',#68182,10.) ;
#9148=VECTOR('',#68185,10.) ;
#9149=VECTOR('',#68192,10.) ;
#9150=VECTOR('',#68195,10.) ;
#9151=VECTOR('',#68198,10.) ;
#9152=VECTOR('',#68205,10.) ;
#9153=VECTOR('',#68214,9.99999999999999) ;
#9154=VECTOR('',#68223,9.99999999999999) ;
#9155=VECTOR('',#68232,10.) ;
#9156=VECTOR('',#68241,10.) ;
#9157=VECTOR('',#68250,10.) ;
#9158=VECTOR('',#68259,10.) ;
#9159=VECTOR('',#68268,9.99999999999999) ;
#9160=VECTOR('',#68293,9.99999999999999) ;
#9161=VECTOR('',#68306,10.) ;
#9162=VECTOR('',#68319,10.) ;
#9163=VECTOR('',#68332,10.) ;
#9164=VECTOR('',#68345,10.) ;
#9165=VECTOR('',#68358,9.99999999999999) ;
#9166=VECTOR('',#68371,9.99999999999999) ;
#9167=VECTOR('',#68384,10.) ;
#9168=VECTOR('',#68397,10.) ;
#9169=VECTOR('',#68408,10.) ;
#9170=VECTOR('',#68409,10.) ;
#9171=VECTOR('',#68412,10.) ;
#9172=VECTOR('',#68415,10.) ;
#9173=VECTOR('',#68420,10.) ;
#9174=VECTOR('',#68421,10.) ;
#9175=VECTOR('',#68424,10.) ;
#9176=VECTOR('',#68425,10.) ;
#9177=VECTOR('',#68430,10.) ;
#9178=VECTOR('',#68431,10.) ;
#9179=VECTOR('',#68434,10.) ;
#9180=VECTOR('',#68435,10.) ;
#9181=VECTOR('',#68440,10.) ;
#9182=VECTOR('',#68441,10.) ;
#9183=VECTOR('',#68444,10.) ;
#9184=VECTOR('',#68445,10.) ;
#9185=VECTOR('',#68450,10.) ;
#9186=VECTOR('',#68451,10.) ;
#9187=VECTOR('',#68454,10.) ;
#9188=VECTOR('',#68455,10.) ;
#9189=VECTOR('',#68460,10.) ;
#9190=VECTOR('',#68461,10.) ;
#9191=VECTOR('',#68464,10.) ;
#9192=VECTOR('',#68465,10.) ;
#9193=VECTOR('',#68470,10.) ;
#9194=VECTOR('',#68471,10.) ;
#9195=VECTOR('',#68474,10.) ;
#9196=VECTOR('',#68475,10.) ;
#9197=VECTOR('',#68480,10.) ;
#9198=VECTOR('',#68481,10.) ;
#9199=VECTOR('',#68484,10.) ;
#9200=VECTOR('',#68485,10.) ;
#9201=VECTOR('',#68490,10.) ;
#9202=VECTOR('',#68491,10.) ;
#9203=VECTOR('',#68494,10.) ;
#9204=VECTOR('',#68495,10.) ;
#9205=VECTOR('',#68500,10.) ;
#9206=VECTOR('',#68501,10.) ;
#9207=VECTOR('',#68504,10.) ;
#9208=VECTOR('',#68527,2.) ;
#10492=CYLINDRICAL_SURFACE('',#54060,0.15) ;
#10493=CYLINDRICAL_SURFACE('',#54064,0.15) ;
#10494=CYLINDRICAL_SURFACE('',#54068,0.15) ;
#10495=CYLINDRICAL_SURFACE('',#54072,0.15) ;
#10496=CYLINDRICAL_SURFACE('',#54076,0.15) ;
#10497=CYLINDRICAL_SURFACE('',#54080,0.15) ;
#10498=CYLINDRICAL_SURFACE('',#54084,0.15) ;
#10499=CYLINDRICAL_SURFACE('',#54088,0.15) ;
#10500=CYLINDRICAL_SURFACE('',#54092,0.15) ;
#10501=CYLINDRICAL_SURFACE('',#54096,0.15) ;
#10502=CYLINDRICAL_SURFACE('',#54100,0.15) ;
#10503=CYLINDRICAL_SURFACE('',#54104,0.15) ;
#10504=CYLINDRICAL_SURFACE('',#54108,0.15) ;
#10505=CYLINDRICAL_SURFACE('',#54112,0.15) ;
#10506=CYLINDRICAL_SURFACE('',#54116,0.15) ;
#10507=CYLINDRICAL_SURFACE('',#54120,0.15) ;
#10508=CYLINDRICAL_SURFACE('',#54124,0.15) ;
#10509=CYLINDRICAL_SURFACE('',#54128,0.15) ;
#10510=CYLINDRICAL_SURFACE('',#54132,0.15) ;
#10511=CYLINDRICAL_SURFACE('',#54136,0.15) ;
#10512=CYLINDRICAL_SURFACE('',#54140,0.15) ;
#10513=CYLINDRICAL_SURFACE('',#54144,0.15) ;
#10514=CYLINDRICAL_SURFACE('',#54148,0.15) ;
#10515=CYLINDRICAL_SURFACE('',#54152,0.15) ;
#10516=CYLINDRICAL_SURFACE('',#54156,0.15) ;
#10517=CYLINDRICAL_SURFACE('',#54160,0.15) ;
#10518=CYLINDRICAL_SURFACE('',#54164,0.15) ;
#10519=CYLINDRICAL_SURFACE('',#54168,0.15) ;
#10520=CYLINDRICAL_SURFACE('',#54172,0.15) ;
#10521=CYLINDRICAL_SURFACE('',#54176,0.15) ;
#10522=CYLINDRICAL_SURFACE('',#54180,0.15) ;
#10523=CYLINDRICAL_SURFACE('',#54184,0.15) ;
#10524=CYLINDRICAL_SURFACE('',#54188,0.15) ;
#10525=CYLINDRICAL_SURFACE('',#54192,0.15) ;
#10526=CYLINDRICAL_SURFACE('',#54196,0.15) ;
#10527=CYLINDRICAL_SURFACE('',#54200,0.15) ;
#10528=CYLINDRICAL_SURFACE('',#54204,0.15) ;
#10529=CYLINDRICAL_SURFACE('',#54208,0.15) ;
#10530=CYLINDRICAL_SURFACE('',#54212,0.15) ;
#10531=CYLINDRICAL_SURFACE('',#54216,0.15) ;
#10532=CYLINDRICAL_SURFACE('',#54218,0.500000000000003) ;
#10533=CYLINDRICAL_SURFACE('',#54221,5.1) ;
#10534=CYLINDRICAL_SURFACE('',#54224,0.500000000000003) ;
#10535=CYLINDRICAL_SURFACE('',#54227,5.1) ;
#10536=CYLINDRICAL_SURFACE('',#54230,0.500000000000003) ;
#10537=CYLINDRICAL_SURFACE('',#54233,5.1) ;
#10538=CYLINDRICAL_SURFACE('',#54236,0.500000000000003) ;
#10539=CYLINDRICAL_SURFACE('',#54239,5.1) ;
#10540=CYLINDRICAL_SURFACE('',#54242,0.500000000000003) ;
#10541=CYLINDRICAL_SURFACE('',#54245,5.1) ;
#10542=CYLINDRICAL_SURFACE('',#54248,0.500000000000003) ;
#10543=CYLINDRICAL_SURFACE('',#54251,5.1) ;
#10544=CYLINDRICAL_SURFACE('',#54254,0.500000000000003) ;
#10545=CYLINDRICAL_SURFACE('',#54257,5.1) ;
#10546=CYLINDRICAL_SURFACE('',#54260,0.500000000000003) ;
#10547=CYLINDRICAL_SURFACE('',#54263,5.1) ;
#10548=CYLINDRICAL_SURFACE('',#54266,0.500000000000003) ;
#10549=CYLINDRICAL_SURFACE('',#54269,5.1) ;
#10550=CYLINDRICAL_SURFACE('',#54272,0.500000000000003) ;
#10551=CYLINDRICAL_SURFACE('',#54275,5.1) ;
#10552=CYLINDRICAL_SURFACE('',#54405,0.15) ;
#10553=CYLINDRICAL_SURFACE('',#54406,0.15) ;
#10554=CYLINDRICAL_SURFACE('',#54407,0.15) ;
#10555=CYLINDRICAL_SURFACE('',#54409,0.15) ;
#10556=CYLINDRICAL_SURFACE('',#54410,0.15) ;
#10557=CYLINDRICAL_SURFACE('',#54411,0.15) ;
#10558=CYLINDRICAL_SURFACE('',#54413,0.15) ;
#10559=CYLINDRICAL_SURFACE('',#54414,0.15) ;
#10560=CYLINDRICAL_SURFACE('',#54415,0.15) ;
#10561=CYLINDRICAL_SURFACE('',#54417,0.15) ;
#10562=CYLINDRICAL_SURFACE('',#54418,0.15) ;
#10563=CYLINDRICAL_SURFACE('',#54419,0.15) ;
#10564=CYLINDRICAL_SURFACE('',#54421,0.15) ;
#10565=CYLINDRICAL_SURFACE('',#54422,0.15) ;
#10566=CYLINDRICAL_SURFACE('',#54423,0.15) ;
#10567=CYLINDRICAL_SURFACE('',#54425,0.15) ;
#10568=CYLINDRICAL_SURFACE('',#54426,0.15) ;
#10569=CYLINDRICAL_SURFACE('',#54427,0.15) ;
#10570=CYLINDRICAL_SURFACE('',#54429,0.15) ;
#10571=CYLINDRICAL_SURFACE('',#54430,0.15) ;
#10572=CYLINDRICAL_SURFACE('',#54431,0.15) ;
#10573=CYLINDRICAL_SURFACE('',#54433,0.15) ;
#10574=CYLINDRICAL_SURFACE('',#54434,0.15) ;
#10575=CYLINDRICAL_SURFACE('',#54435,0.15) ;
#10576=CYLINDRICAL_SURFACE('',#54437,0.15) ;
#10577=CYLINDRICAL_SURFACE('',#54438,0.15) ;
#10578=CYLINDRICAL_SURFACE('',#54439,0.15) ;
#10579=CYLINDRICAL_SURFACE('',#54441,0.15) ;
#10580=CYLINDRICAL_SURFACE('',#54442,0.15) ;
#10581=CYLINDRICAL_SURFACE('',#54443,0.15) ;
#10582=CYLINDRICAL_SURFACE('',#54445,0.15) ;
#10583=CYLINDRICAL_SURFACE('',#54450,0.15) ;
#10584=CYLINDRICAL_SURFACE('',#54456,0.15) ;
#10585=CYLINDRICAL_SURFACE('',#54462,0.15) ;
#10586=CYLINDRICAL_SURFACE('',#54468,0.15) ;
#10587=CYLINDRICAL_SURFACE('',#54474,0.15) ;
#10588=CYLINDRICAL_SURFACE('',#54480,0.15) ;
#10589=CYLINDRICAL_SURFACE('',#54486,0.15) ;
#10590=CYLINDRICAL_SURFACE('',#54492,0.15) ;
#10591=CYLINDRICAL_SURFACE('',#54498,0.15) ;
#10592=CYLINDRICAL_SURFACE('',#54503,5.1) ;
#10593=CYLINDRICAL_SURFACE('',#54505,0.500000000000003) ;
#10594=CYLINDRICAL_SURFACE('',#54509,0.500000000000003) ;
#10595=CYLINDRICAL_SURFACE('',#54512,0.500000000000003) ;
#10596=CYLINDRICAL_SURFACE('',#54515,0.500000000000003) ;
#10597=CYLINDRICAL_SURFACE('',#54518,0.500000000000003) ;
#10598=CYLINDRICAL_SURFACE('',#54521,0.500000000000003) ;
#10599=CYLINDRICAL_SURFACE('',#54524,0.500000000000003) ;
#10600=CYLINDRICAL_SURFACE('',#54527,0.500000000000003) ;
#10601=CYLINDRICAL_SURFACE('',#54530,0.500000000000003) ;
#10602=CYLINDRICAL_SURFACE('',#54533,0.500000000000003) ;
#10603=CYLINDRICAL_SURFACE('',#54534,5.1) ;
#10604=CYLINDRICAL_SURFACE('',#54535,5.1) ;
#10605=CYLINDRICAL_SURFACE('',#54536,5.1) ;
#10606=CYLINDRICAL_SURFACE('',#54537,5.1) ;
#10607=CYLINDRICAL_SURFACE('',#54538,5.1) ;
#10608=CYLINDRICAL_SURFACE('',#54539,5.1) ;
#10609=CYLINDRICAL_SURFACE('',#54540,5.1) ;
#10610=CYLINDRICAL_SURFACE('',#54541,5.1) ;
#10611=CYLINDRICAL_SURFACE('',#54542,5.1) ;
#10612=CYLINDRICAL_SURFACE('',#54543,2.) ;
#13234=FACE_OUTER_BOUND('',#16418,.T.) ;
#13235=FACE_OUTER_BOUND('',#16419,.T.) ;
#13236=FACE_OUTER_BOUND('',#16421,.T.) ;
#13237=FACE_OUTER_BOUND('',#16422,.T.) ;
#13238=FACE_OUTER_BOUND('',#16424,.T.) ;
#13239=FACE_OUTER_BOUND('',#16426,.T.) ;
#13240=FACE_OUTER_BOUND('',#16428,.T.) ;
#13241=FACE_OUTER_BOUND('',#16429,.T.) ;
#13242=FACE_OUTER_BOUND('',#16430,.T.) ;
#13243=FACE_OUTER_BOUND('',#16431,.T.) ;
#13244=FACE_OUTER_BOUND('',#16432,.T.) ;
#13245=FACE_OUTER_BOUND('',#16433,.T.) ;
#13246=FACE_OUTER_BOUND('',#16434,.T.) ;
#13247=FACE_OUTER_BOUND('',#16435,.T.) ;
#13248=FACE_OUTER_BOUND('',#16436,.T.) ;
#13249=FACE_OUTER_BOUND('',#16437,.T.) ;
#13250=FACE_OUTER_BOUND('',#16438,.T.) ;
#13251=FACE_OUTER_BOUND('',#16439,.T.) ;
#13252=FACE_OUTER_BOUND('',#16440,.T.) ;
#13253=FACE_OUTER_BOUND('',#16441,.T.) ;
#13254=FACE_OUTER_BOUND('',#16442,.T.) ;
#13255=FACE_OUTER_BOUND('',#16443,.T.) ;
#13256=FACE_OUTER_BOUND('',#16444,.T.) ;
#13257=FACE_OUTER_BOUND('',#16445,.T.) ;
#13258=FACE_OUTER_BOUND('',#16446,.T.) ;
#13259=FACE_OUTER_BOUND('',#16447,.T.) ;
#13260=FACE_OUTER_BOUND('',#16448,.T.) ;
#13261=FACE_OUTER_BOUND('',#16449,.T.) ;
#13262=FACE_OUTER_BOUND('',#16450,.T.) ;
#13263=FACE_OUTER_BOUND('',#16451,.T.) ;
#13264=FACE_OUTER_BOUND('',#16452,.T.) ;
#13265=FACE_OUTER_BOUND('',#16453,.T.) ;
#13266=FACE_OUTER_BOUND('',#16454,.T.) ;
#13267=FACE_OUTER_BOUND('',#16455,.T.) ;
#13268=FACE_OUTER_BOUND('',#16456,.T.) ;
#13269=FACE_OUTER_BOUND('',#16457,.T.) ;
#13270=FACE_OUTER_BOUND('',#16458,.T.) ;
#13271=FACE_OUTER_BOUND('',#16459,.T.) ;
#13272=FACE_OUTER_BOUND('',#16460,.T.) ;
#13273=FACE_OUTER_BOUND('',#16461,.T.) ;
#13274=FACE_OUTER_BOUND('',#16462,.T.) ;
#13275=FACE_OUTER_BOUND('',#16463,.T.) ;
#13276=FACE_OUTER_BOUND('',#16464,.T.) ;
#13277=FACE_OUTER_BOUND('',#16465,.T.) ;
#13278=FACE_OUTER_BOUND('',#16466,.T.) ;
#13279=FACE_OUTER_BOUND('',#16467,.T.) ;
#13280=FACE_OUTER_BOUND('',#16468,.T.) ;
#13281=FACE_OUTER_BOUND('',#16469,.T.) ;
#13282=FACE_OUTER_BOUND('',#16470,.T.) ;
#13283=FACE_OUTER_BOUND('',#16471,.T.) ;
#13284=FACE_OUTER_BOUND('',#16472,.T.) ;
#13285=FACE_OUTER_BOUND('',#16473,.T.) ;
#13286=FACE_OUTER_BOUND('',#16474,.T.) ;
#13287=FACE_OUTER_BOUND('',#16475,.T.) ;
#13288=FACE_OUTER_BOUND('',#16476,.T.) ;
#13289=FACE_OUTER_BOUND('',#16477,.T.) ;
#13290=FACE_OUTER_BOUND('',#16478,.T.) ;
#13291=FACE_OUTER_BOUND('',#16479,.T.) ;
#13292=FACE_OUTER_BOUND('',#16480,.T.) ;
#13293=FACE_OUTER_BOUND('',#16481,.T.) ;
#13294=FACE_OUTER_BOUND('',#16482,.T.) ;
#13295=FACE_OUTER_BOUND('',#16483,.T.) ;
#13296=FACE_OUTER_BOUND('',#16484,.T.) ;
#13297=FACE_OUTER_BOUND('',#16485,.T.) ;
#13298=FACE_OUTER_BOUND('',#16486,.T.) ;
#13299=FACE_OUTER_BOUND('',#16487,.T.) ;
#13300=FACE_OUTER_BOUND('',#16488,.T.) ;
#13301=FACE_OUTER_BOUND('',#16489,.T.) ;
#13302=FACE_OUTER_BOUND('',#16490,.T.) ;
#13303=FACE_OUTER_BOUND('',#16491,.T.) ;
#13304=FACE_OUTER_BOUND('',#16492,.T.) ;
#13305=FACE_OUTER_BOUND('',#16493,.T.) ;
#13306=FACE_OUTER_BOUND('',#16494,.T.) ;
#13307=FACE_OUTER_BOUND('',#16495,.T.) ;
#13308=FACE_OUTER_BOUND('',#16496,.T.) ;
#13309=FACE_OUTER_BOUND('',#16497,.T.) ;
#13310=FACE_OUTER_BOUND('',#16498,.T.) ;
#13311=FACE_OUTER_BOUND('',#16499,.T.) ;
#13312=FACE_OUTER_BOUND('',#16500,.T.) ;
#13313=FACE_OUTER_BOUND('',#16501,.T.) ;
#13314=FACE_OUTER_BOUND('',#16502,.T.) ;
#13315=FACE_OUTER_BOUND('',#16503,.T.) ;
#13316=FACE_OUTER_BOUND('',#16504,.T.) ;
#13317=FACE_OUTER_BOUND('',#16505,.T.) ;
#13318=FACE_OUTER_BOUND('',#16506,.T.) ;
#13319=FACE_OUTER_BOUND('',#16507,.T.) ;
#13320=FACE_OUTER_BOUND('',#16508,.T.) ;
#13321=FACE_OUTER_BOUND('',#16509,.T.) ;
#13322=FACE_OUTER_BOUND('',#16510,.T.) ;
#13323=FACE_OUTER_BOUND('',#16511,.T.) ;
#13324=FACE_OUTER_BOUND('',#16512,.T.) ;
#13325=FACE_OUTER_BOUND('',#16513,.T.) ;
#13326=FACE_OUTER_BOUND('',#16514,.T.) ;
#13327=FACE_OUTER_BOUND('',#16515,.T.) ;
#13328=FACE_OUTER_BOUND('',#16516,.T.) ;
#13329=FACE_OUTER_BOUND('',#16517,.T.) ;
#13330=FACE_OUTER_BOUND('',#16518,.T.) ;
#13331=FACE_OUTER_BOUND('',#16519,.T.) ;
#13332=FACE_OUTER_BOUND('',#16520,.T.) ;
#13333=FACE_OUTER_BOUND('',#16521,.T.) ;
#13334=FACE_OUTER_BOUND('',#16522,.T.) ;
#13335=FACE_OUTER_BOUND('',#16523,.T.) ;
#13336=FACE_OUTER_BOUND('',#16524,.T.) ;
#13337=FACE_OUTER_BOUND('',#16525,.T.) ;
#13338=FACE_OUTER_BOUND('',#16526,.T.) ;
#13339=FACE_OUTER_BOUND('',#16527,.T.) ;
#13340=FACE_OUTER_BOUND('',#16528,.T.) ;
#13341=FACE_OUTER_BOUND('',#16529,.T.) ;
#13342=FACE_OUTER_BOUND('',#16530,.T.) ;
#13343=FACE_OUTER_BOUND('',#16531,.T.) ;
#13344=FACE_OUTER_BOUND('',#16532,.T.) ;
#13345=FACE_OUTER_BOUND('',#16533,.T.) ;
#13346=FACE_OUTER_BOUND('',#16534,.T.) ;
#13347=FACE_OUTER_BOUND('',#16535,.T.) ;
#13348=FACE_OUTER_BOUND('',#16536,.T.) ;
#13349=FACE_OUTER_BOUND('',#16537,.T.) ;
#13350=FACE_OUTER_BOUND('',#16538,.T.) ;
#13351=FACE_OUTER_BOUND('',#16539,.T.) ;
#13352=FACE_OUTER_BOUND('',#16540,.T.) ;
#13353=FACE_OUTER_BOUND('',#16541,.T.) ;
#13354=FACE_OUTER_BOUND('',#16542,.T.) ;
#13355=FACE_OUTER_BOUND('',#16543,.T.) ;
#13356=FACE_OUTER_BOUND('',#16544,.T.) ;
#13357=FACE_OUTER_BOUND('',#16545,.T.) ;
#13358=FACE_OUTER_BOUND('',#16546,.T.) ;
#13359=FACE_OUTER_BOUND('',#16547,.T.) ;
#13360=FACE_OUTER_BOUND('',#16548,.T.) ;
#13361=FACE_OUTER_BOUND('',#16549,.T.) ;
#13362=FACE_OUTER_BOUND('',#16550,.T.) ;
#13363=FACE_OUTER_BOUND('',#16551,.T.) ;
#13364=FACE_OUTER_BOUND('',#16552,.T.) ;
#13365=FACE_OUTER_BOUND('',#16553,.T.) ;
#13366=FACE_OUTER_BOUND('',#16554,.T.) ;
#13367=FACE_OUTER_BOUND('',#16555,.T.) ;
#13368=FACE_OUTER_BOUND('',#16556,.T.) ;
#13369=FACE_OUTER_BOUND('',#16557,.T.) ;
#13370=FACE_OUTER_BOUND('',#16558,.T.) ;
#13371=FACE_OUTER_BOUND('',#16559,.T.) ;
#13372=FACE_OUTER_BOUND('',#16560,.T.) ;
#13373=FACE_OUTER_BOUND('',#16561,.T.) ;
#13374=FACE_OUTER_BOUND('',#16562,.T.) ;
#13375=FACE_OUTER_BOUND('',#16563,.T.) ;
#13376=FACE_OUTER_BOUND('',#16564,.T.) ;
#13377=FACE_OUTER_BOUND('',#16565,.T.) ;
#13378=FACE_OUTER_BOUND('',#16566,.T.) ;
#13379=FACE_OUTER_BOUND('',#16567,.T.) ;
#13380=FACE_OUTER_BOUND('',#16568,.T.) ;
#13381=FACE_OUTER_BOUND('',#16569,.T.) ;
#13382=FACE_OUTER_BOUND('',#16570,.T.) ;
#13383=FACE_OUTER_BOUND('',#16571,.T.) ;
#13384=FACE_OUTER_BOUND('',#16572,.T.) ;
#13385=FACE_OUTER_BOUND('',#16573,.T.) ;
#13386=FACE_OUTER_BOUND('',#16574,.T.) ;
#13387=FACE_OUTER_BOUND('',#16575,.T.) ;
#13388=FACE_OUTER_BOUND('',#16576,.T.) ;
#13389=FACE_OUTER_BOUND('',#16577,.T.) ;
#13390=FACE_OUTER_BOUND('',#16578,.T.) ;
#13391=FACE_OUTER_BOUND('',#16579,.T.) ;
#13392=FACE_OUTER_BOUND('',#16580,.T.) ;
#13393=FACE_OUTER_BOUND('',#16581,.T.) ;
#13394=FACE_OUTER_BOUND('',#16582,.T.) ;
#13395=FACE_OUTER_BOUND('',#16583,.T.) ;
#13396=FACE_OUTER_BOUND('',#16584,.T.) ;
#13397=FACE_OUTER_BOUND('',#16585,.T.) ;
#13398=FACE_OUTER_BOUND('',#16586,.T.) ;
#13399=FACE_OUTER_BOUND('',#16587,.T.) ;
#13400=FACE_OUTER_BOUND('',#16588,.T.) ;
#13401=FACE_OUTER_BOUND('',#16589,.T.) ;
#13402=FACE_OUTER_BOUND('',#16590,.T.) ;
#13403=FACE_OUTER_BOUND('',#16591,.T.) ;
#13404=FACE_OUTER_BOUND('',#16592,.T.) ;
#13405=FACE_OUTER_BOUND('',#16593,.T.) ;
#13406=FACE_OUTER_BOUND('',#16594,.T.) ;
#13407=FACE_OUTER_BOUND('',#16595,.T.) ;
#13408=FACE_OUTER_BOUND('',#16596,.T.) ;
#13409=FACE_OUTER_BOUND('',#16597,.T.) ;
#13410=FACE_OUTER_BOUND('',#16598,.T.) ;
#13411=FACE_OUTER_BOUND('',#16599,.T.) ;
#13412=FACE_OUTER_BOUND('',#16600,.T.) ;
#13413=FACE_OUTER_BOUND('',#16601,.T.) ;
#13414=FACE_OUTER_BOUND('',#16602,.T.) ;
#13415=FACE_OUTER_BOUND('',#16603,.T.) ;
#13416=FACE_OUTER_BOUND('',#16604,.T.) ;
#13417=FACE_OUTER_BOUND('',#16605,.T.) ;
#13418=FACE_OUTER_BOUND('',#16606,.T.) ;
#13419=FACE_OUTER_BOUND('',#16607,.T.) ;
#13420=FACE_OUTER_BOUND('',#16608,.T.) ;
#13421=FACE_OUTER_BOUND('',#16609,.T.) ;
#13422=FACE_OUTER_BOUND('',#16610,.T.) ;
#13423=FACE_OUTER_BOUND('',#16611,.T.) ;
#13424=FACE_OUTER_BOUND('',#16612,.T.) ;
#13425=FACE_OUTER_BOUND('',#16613,.T.) ;
#13426=FACE_OUTER_BOUND('',#16614,.T.) ;
#13427=FACE_OUTER_BOUND('',#16615,.T.) ;
#13428=FACE_OUTER_BOUND('',#16616,.T.) ;
#13429=FACE_OUTER_BOUND('',#16617,.T.) ;
#13430=FACE_OUTER_BOUND('',#16618,.T.) ;
#13431=FACE_OUTER_BOUND('',#16619,.T.) ;
#13432=FACE_OUTER_BOUND('',#16620,.T.) ;
#13433=FACE_OUTER_BOUND('',#16621,.T.) ;
#13434=FACE_OUTER_BOUND('',#16622,.T.) ;
#13435=FACE_OUTER_BOUND('',#16623,.T.) ;
#13436=FACE_OUTER_BOUND('',#16624,.T.) ;
#13437=FACE_OUTER_BOUND('',#16625,.T.) ;
#13438=FACE_OUTER_BOUND('',#16626,.T.) ;
#13439=FACE_OUTER_BOUND('',#16627,.T.) ;
#13440=FACE_OUTER_BOUND('',#16628,.T.) ;
#13441=FACE_OUTER_BOUND('',#16629,.T.) ;
#13442=FACE_OUTER_BOUND('',#16630,.T.) ;
#13443=FACE_OUTER_BOUND('',#16631,.T.) ;
#13444=FACE_OUTER_BOUND('',#16632,.T.) ;
#13445=FACE_OUTER_BOUND('',#16633,.T.) ;
#13446=FACE_OUTER_BOUND('',#16634,.T.) ;
#13447=FACE_OUTER_BOUND('',#16635,.T.) ;
#13448=FACE_OUTER_BOUND('',#16636,.T.) ;
#13449=FACE_OUTER_BOUND('',#16637,.T.) ;
#13450=FACE_OUTER_BOUND('',#16638,.T.) ;
#13451=FACE_OUTER_BOUND('',#16639,.T.) ;
#13452=FACE_OUTER_BOUND('',#16640,.T.) ;
#13453=FACE_OUTER_BOUND('',#16641,.T.) ;
#13454=FACE_OUTER_BOUND('',#16642,.T.) ;
#13455=FACE_OUTER_BOUND('',#16643,.T.) ;
#13456=FACE_OUTER_BOUND('',#16644,.T.) ;
#13457=FACE_OUTER_BOUND('',#16645,.T.) ;
#13458=FACE_OUTER_BOUND('',#16646,.T.) ;
#13459=FACE_OUTER_BOUND('',#16647,.T.) ;
#13460=FACE_OUTER_BOUND('',#16648,.T.) ;
#13461=FACE_OUTER_BOUND('',#16649,.T.) ;
#13462=FACE_OUTER_BOUND('',#16650,.T.) ;
#13463=FACE_OUTER_BOUND('',#16651,.T.) ;
#13464=FACE_OUTER_BOUND('',#16652,.T.) ;
#13465=FACE_OUTER_BOUND('',#16653,.T.) ;
#13466=FACE_OUTER_BOUND('',#16654,.T.) ;
#13467=FACE_OUTER_BOUND('',#16655,.T.) ;
#13468=FACE_OUTER_BOUND('',#16656,.T.) ;
#13469=FACE_OUTER_BOUND('',#16657,.T.) ;
#13470=FACE_OUTER_BOUND('',#16658,.T.) ;
#13471=FACE_OUTER_BOUND('',#16659,.T.) ;
#13472=FACE_OUTER_BOUND('',#16660,.T.) ;
#13473=FACE_OUTER_BOUND('',#16661,.T.) ;
#13474=FACE_OUTER_BOUND('',#16662,.T.) ;
#13475=FACE_OUTER_BOUND('',#16663,.T.) ;
#13476=FACE_OUTER_BOUND('',#16664,.T.) ;
#13477=FACE_OUTER_BOUND('',#16665,.T.) ;
#13478=FACE_OUTER_BOUND('',#16666,.T.) ;
#13479=FACE_OUTER_BOUND('',#16667,.T.) ;
#13480=FACE_OUTER_BOUND('',#16668,.T.) ;
#13481=FACE_OUTER_BOUND('',#16669,.T.) ;
#13482=FACE_OUTER_BOUND('',#16670,.T.) ;
#13483=FACE_OUTER_BOUND('',#16671,.T.) ;
#13484=FACE_OUTER_BOUND('',#16672,.T.) ;
#13485=FACE_OUTER_BOUND('',#16673,.T.) ;
#13486=FACE_OUTER_BOUND('',#16674,.T.) ;
#13487=FACE_OUTER_BOUND('',#16675,.T.) ;
#13488=FACE_OUTER_BOUND('',#16676,.T.) ;
#13489=FACE_OUTER_BOUND('',#16677,.T.) ;
#13490=FACE_OUTER_BOUND('',#16678,.T.) ;
#13491=FACE_OUTER_BOUND('',#16679,.T.) ;
#13492=FACE_OUTER_BOUND('',#16680,.T.) ;
#13493=FACE_OUTER_BOUND('',#16681,.T.) ;
#13494=FACE_OUTER_BOUND('',#16682,.T.) ;
#13495=FACE_OUTER_BOUND('',#16683,.T.) ;
#13496=FACE_OUTER_BOUND('',#16684,.T.) ;
#13497=FACE_OUTER_BOUND('',#16685,.T.) ;
#13498=FACE_OUTER_BOUND('',#16686,.T.) ;
#13499=FACE_OUTER_BOUND('',#16687,.T.) ;
#13500=FACE_OUTER_BOUND('',#16688,.T.) ;
#13501=FACE_OUTER_BOUND('',#16689,.T.) ;
#13502=FACE_OUTER_BOUND('',#16690,.T.) ;
#13503=FACE_OUTER_BOUND('',#16691,.T.) ;
#13504=FACE_OUTER_BOUND('',#16692,.T.) ;
#13505=FACE_OUTER_BOUND('',#16693,.T.) ;
#13506=FACE_OUTER_BOUND('',#16694,.T.) ;
#13507=FACE_OUTER_BOUND('',#16695,.T.) ;
#13508=FACE_OUTER_BOUND('',#16696,.T.) ;
#13509=FACE_OUTER_BOUND('',#16697,.T.) ;
#13510=FACE_OUTER_BOUND('',#16698,.T.) ;
#13511=FACE_OUTER_BOUND('',#16699,.T.) ;
#13512=FACE_OUTER_BOUND('',#16700,.T.) ;
#13513=FACE_OUTER_BOUND('',#16701,.T.) ;
#13514=FACE_OUTER_BOUND('',#16702,.T.) ;
#13515=FACE_OUTER_BOUND('',#16703,.T.) ;
#13516=FACE_OUTER_BOUND('',#16704,.T.) ;
#13517=FACE_OUTER_BOUND('',#16705,.T.) ;
#13518=FACE_OUTER_BOUND('',#16706,.T.) ;
#13519=FACE_OUTER_BOUND('',#16707,.T.) ;
#13520=FACE_OUTER_BOUND('',#16708,.T.) ;
#13521=FACE_OUTER_BOUND('',#16709,.T.) ;
#13522=FACE_OUTER_BOUND('',#16710,.T.) ;
#13523=FACE_OUTER_BOUND('',#16711,.T.) ;
#13524=FACE_OUTER_BOUND('',#16712,.T.) ;
#16418=EDGE_LOOP('',(#42764,#42765,#42766,#42767)) ;
#16419=EDGE_LOOP('',(#42768)) ;
#16420=EDGE_LOOP('',(#42769)) ;
#16421=EDGE_LOOP('',(#42770,#42771,#42772,#42773)) ;
#16422=EDGE_LOOP('',(#42774)) ;
#16423=EDGE_LOOP('',(#42775)) ;
#16424=EDGE_LOOP('',(#42776)) ;
#16425=EDGE_LOOP('',(#42777)) ;
#16426=EDGE_LOOP('',(#42778)) ;
#16427=EDGE_LOOP('',(#42779)) ;
#16428=EDGE_LOOP('',(#42780,#42781,#42782,#42783,#42784)) ;
#16429=EDGE_LOOP('',(#42785,#42786,#42787,#42788,#42789)) ;
#16430=EDGE_LOOP('',(#42790,#42791,#42792,#42793)) ;
#16431=EDGE_LOOP('',(#42794,#42795,#42796,#42797)) ;
#16432=EDGE_LOOP('',(#42798,#42799,#42800,#42801)) ;
#16433=EDGE_LOOP('',(#42802,#42803,#42804,#42805)) ;
#16434=EDGE_LOOP('',(#42806,#42807,#42808,#42809)) ;
#16435=EDGE_LOOP('',(#42810,#42811,#42812,#42813)) ;
#16436=EDGE_LOOP('',(#42814,#42815,#42816,#42817)) ;
#16437=EDGE_LOOP('',(#42818,#42819,#42820,#42821)) ;
#16438=EDGE_LOOP('',(#42822,#42823,#42824,#42825)) ;
#16439=EDGE_LOOP('',(#42826,#42827,#42828,#42829)) ;
#16440=EDGE_LOOP('',(#42830,#42831,#42832,#42833)) ;
#16441=EDGE_LOOP('',(#42834,#42835,#42836,#42837)) ;
#16442=EDGE_LOOP('',(#42838,#42839,#42840,#42841)) ;
#16443=EDGE_LOOP('',(#42842,#42843,#42844,#42845)) ;
#16444=EDGE_LOOP('',(#42846,#42847,#42848,#42849)) ;
#16445=EDGE_LOOP('',(#42850,#42851,#42852,#42853)) ;
#16446=EDGE_LOOP('',(#42854,#42855,#42856,#42857)) ;
#16447=EDGE_LOOP('',(#42858,#42859,#42860,#42861)) ;
#16448=EDGE_LOOP('',(#42862,#42863,#42864,#42865)) ;
#16449=EDGE_LOOP('',(#42866,#42867,#42868,#42869)) ;
#16450=EDGE_LOOP('',(#42870,#42871,#42872,#42873)) ;
#16451=EDGE_LOOP('',(#42874,#42875,#42876,#42877)) ;
#16452=EDGE_LOOP('',(#42878,#42879,#42880,#42881)) ;
#16453=EDGE_LOOP('',(#42882,#42883,#42884,#42885)) ;
#16454=EDGE_LOOP('',(#42886,#42887,#42888,#42889)) ;
#16455=EDGE_LOOP('',(#42890,#42891,#42892,#42893)) ;
#16456=EDGE_LOOP('',(#42894,#42895,#42896,#42897)) ;
#16457=EDGE_LOOP('',(#42898,#42899,#42900,#42901)) ;
#16458=EDGE_LOOP('',(#42902,#42903,#42904,#42905)) ;
#16459=EDGE_LOOP('',(#42906,#42907,#42908,#42909)) ;
#16460=EDGE_LOOP('',(#42910,#42911,#42912,#42913)) ;
#16461=EDGE_LOOP('',(#42914,#42915,#42916,#42917)) ;
#16462=EDGE_LOOP('',(#42918,#42919,#42920,#42921)) ;
#16463=EDGE_LOOP('',(#42922,#42923,#42924,#42925)) ;
#16464=EDGE_LOOP('',(#42926,#42927,#42928,#42929)) ;
#16465=EDGE_LOOP('',(#42930,#42931,#42932,#42933)) ;
#16466=EDGE_LOOP('',(#42934,#42935,#42936,#42937)) ;
#16467=EDGE_LOOP('',(#42938,#42939,#42940,#42941)) ;
#16468=EDGE_LOOP('',(#42942,#42943,#42944,#42945)) ;
#16469=EDGE_LOOP('',(#42946,#42947,#42948,#42949)) ;
#16470=EDGE_LOOP('',(#42950,#42951,#42952,#42953)) ;
#16471=EDGE_LOOP('',(#42954,#42955,#42956,#42957)) ;
#16472=EDGE_LOOP('',(#42958,#42959,#42960,#42961)) ;
#16473=EDGE_LOOP('',(#42962,#42963,#42964,#42965)) ;
#16474=EDGE_LOOP('',(#42966,#42967,#42968,#42969)) ;
#16475=EDGE_LOOP('',(#42970,#42971,#42972,#42973)) ;
#16476=EDGE_LOOP('',(#42974,#42975,#42976,#42977)) ;
#16477=EDGE_LOOP('',(#42978,#42979,#42980,#42981)) ;
#16478=EDGE_LOOP('',(#42982,#42983,#42984,#42985)) ;
#16479=EDGE_LOOP('',(#42986,#42987,#42988,#42989)) ;
#16480=EDGE_LOOP('',(#42990,#42991,#42992,#42993)) ;
#16481=EDGE_LOOP('',(#42994,#42995,#42996,#42997)) ;
#16482=EDGE_LOOP('',(#42998,#42999,#43000,#43001)) ;
#16483=EDGE_LOOP('',(#43002,#43003,#43004,#43005)) ;
#16484=EDGE_LOOP('',(#43006,#43007,#43008,#43009)) ;
#16485=EDGE_LOOP('',(#43010,#43011,#43012,#43013)) ;
#16486=EDGE_LOOP('',(#43014,#43015,#43016,#43017)) ;
#16487=EDGE_LOOP('',(#43018,#43019,#43020,#43021)) ;
#16488=EDGE_LOOP('',(#43022,#43023,#43024,#43025)) ;
#16489=EDGE_LOOP('',(#43026,#43027,#43028,#43029)) ;
#16490=EDGE_LOOP('',(#43030,#43031,#43032,#43033)) ;
#16491=EDGE_LOOP('',(#43034,#43035,#43036,#43037)) ;
#16492=EDGE_LOOP('',(#43038,#43039,#43040,#43041)) ;
#16493=EDGE_LOOP('',(#43042,#43043,#43044,#43045)) ;
#16494=EDGE_LOOP('',(#43046,#43047,#43048,#43049)) ;
#16495=EDGE_LOOP('',(#43050,#43051,#43052,#43053)) ;
#16496=EDGE_LOOP('',(#43054,#43055,#43056,#43057)) ;
#16497=EDGE_LOOP('',(#43058,#43059,#43060,#43061)) ;
#16498=EDGE_LOOP('',(#43062,#43063,#43064,#43065)) ;
#16499=EDGE_LOOP('',(#43066,#43067,#43068,#43069)) ;
#16500=EDGE_LOOP('',(#43070,#43071,#43072,#43073)) ;
#16501=EDGE_LOOP('',(#43074,#43075,#43076,#43077)) ;
#16502=EDGE_LOOP('',(#43078,#43079,#43080,#43081)) ;
#16503=EDGE_LOOP('',(#43082,#43083,#43084,#43085)) ;
#16504=EDGE_LOOP('',(#43086,#43087,#43088,#43089)) ;
#16505=EDGE_LOOP('',(#43090,#43091,#43092,#43093)) ;
#16506=EDGE_LOOP('',(#43094,#43095,#43096,#43097)) ;
#16507=EDGE_LOOP('',(#43098,#43099,#43100,#43101)) ;
#16508=EDGE_LOOP('',(#43102,#43103,#43104,#43105)) ;
#16509=EDGE_LOOP('',(#43106,#43107,#43108,#43109)) ;
#16510=EDGE_LOOP('',(#43110,#43111,#43112,#43113)) ;
#16511=EDGE_LOOP('',(#43114,#43115,#43116,#43117)) ;
#16512=EDGE_LOOP('',(#43118,#43119,#43120,#43121)) ;
#16513=EDGE_LOOP('',(#43122,#43123,#43124,#43125)) ;
#16514=EDGE_LOOP('',(#43126,#43127,#43128,#43129)) ;
#16515=EDGE_LOOP('',(#43130,#43131,#43132,#43133)) ;
#16516=EDGE_LOOP('',(#43134,#43135,#43136,#43137)) ;
#16517=EDGE_LOOP('',(#43138,#43139,#43140,#43141)) ;
#16518=EDGE_LOOP('',(#43142,#43143,#43144,#43145)) ;
#16519=EDGE_LOOP('',(#43146,#43147,#43148,#43149)) ;
#16520=EDGE_LOOP('',(#43150,#43151,#43152,#43153)) ;
#16521=EDGE_LOOP('',(#43154,#43155,#43156,#43157)) ;
#16522=EDGE_LOOP('',(#43158,#43159,#43160,#43161)) ;
#16523=EDGE_LOOP('',(#43162,#43163,#43164,#43165)) ;
#16524=EDGE_LOOP('',(#43166,#43167,#43168,#43169)) ;
#16525=EDGE_LOOP('',(#43170,#43171,#43172,#43173)) ;
#16526=EDGE_LOOP('',(#43174,#43175,#43176,#43177)) ;
#16527=EDGE_LOOP('',(#43178,#43179,#43180,#43181)) ;
#16528=EDGE_LOOP('',(#43182,#43183,#43184,#43185)) ;
#16529=EDGE_LOOP('',(#43186,#43187,#43188,#43189)) ;
#16530=EDGE_LOOP('',(#43190,#43191,#43192,#43193)) ;
#16531=EDGE_LOOP('',(#43194,#43195,#43196,#43197)) ;
#16532=EDGE_LOOP('',(#43198,#43199,#43200,#43201)) ;
#16533=EDGE_LOOP('',(#43202,#43203,#43204,#43205)) ;
#16534=EDGE_LOOP('',(#43206,#43207,#43208,#43209)) ;
#16535=EDGE_LOOP('',(#43210,#43211,#43212,#43213)) ;
#16536=EDGE_LOOP('',(#43214,#43215,#43216,#43217)) ;
#16537=EDGE_LOOP('',(#43218,#43219,#43220,#43221)) ;
#16538=EDGE_LOOP('',(#43222,#43223,#43224,#43225)) ;
#16539=EDGE_LOOP('',(#43226,#43227,#43228,#43229)) ;
#16540=EDGE_LOOP('',(#43230,#43231,#43232,#43233)) ;
#16541=EDGE_LOOP('',(#43234,#43235,#43236,#43237)) ;
#16542=EDGE_LOOP('',(#43238,#43239,#43240,#43241)) ;
#16543=EDGE_LOOP('',(#43242,#43243,#43244,#43245)) ;
#16544=EDGE_LOOP('',(#43246,#43247,#43248,#43249)) ;
#16545=EDGE_LOOP('',(#43250,#43251,#43252,#43253)) ;
#16546=EDGE_LOOP('',(#43254,#43255,#43256,#43257)) ;
#16547=EDGE_LOOP('',(#43258,#43259,#43260,#43261)) ;
#16548=EDGE_LOOP('',(#43262,#43263,#43264,#43265)) ;
#16549=EDGE_LOOP('',(#43266,#43267,#43268,#43269)) ;
#16550=EDGE_LOOP('',(#43270,#43271,#43272,#43273)) ;
#16551=EDGE_LOOP('',(#43274,#43275,#43276,#43277)) ;
#16552=EDGE_LOOP('',(#43278,#43279,#43280,#43281)) ;
#16553=EDGE_LOOP('',(#43282,#43283,#43284,#43285)) ;
#16554=EDGE_LOOP('',(#43286,#43287,#43288,#43289)) ;
#16555=EDGE_LOOP('',(#43290,#43291,#43292,#43293)) ;
#16556=EDGE_LOOP('',(#43294,#43295,#43296,#43297)) ;
#16557=EDGE_LOOP('',(#43298,#43299,#43300,#43301)) ;
#16558=EDGE_LOOP('',(#43302,#43303,#43304,#43305)) ;
#16559=EDGE_LOOP('',(#43306,#43307,#43308,#43309)) ;
#16560=EDGE_LOOP('',(#43310,#43311,#43312,#43313)) ;
#16561=EDGE_LOOP('',(#43314,#43315,#43316,#43317)) ;
#16562=EDGE_LOOP('',(#43318,#43319,#43320,#43321)) ;
#16563=EDGE_LOOP('',(#43322,#43323,#43324,#43325)) ;
#16564=EDGE_LOOP('',(#43326,#43327,#43328,#43329)) ;
#16565=EDGE_LOOP('',(#43330,#43331,#43332,#43333)) ;
#16566=EDGE_LOOP('',(#43334,#43335,#43336,#43337)) ;
#16567=EDGE_LOOP('',(#43338,#43339,#43340,#43341)) ;
#16568=EDGE_LOOP('',(#43342,#43343,#43344,#43345,#43346)) ;
#16569=EDGE_LOOP('',(#43347,#43348,#43349,#43350,#43351,#43352,#43353,#43354,
#43355,#43356,#43357,#43358,#43359,#43360,#43361,#43362,#43363,#43364,#43365,
#43366,#43367,#43368,#43369,#43370,#43371,#43372,#43373,#43374,#43375,#43376,
#43377,#43378,#43379,#43380,#43381,#43382,#43383,#43384,#43385,#43386,#43387,
#43388,#43389,#43390,#43391)) ;
#16570=EDGE_LOOP('',(#43392,#43393,#43394,#43395)) ;
#16571=EDGE_LOOP('',(#43396,#43397,#43398,#43399,#43400,#43401,#43402,#43403,
#43404,#43405,#43406,#43407,#43408,#43409,#43410,#43411,#43412,#43413,#43414,
#43415,#43416,#43417,#43418,#43419,#43420,#43421,#43422,#43423,#43424,#43425,
#43426,#43427,#43428,#43429,#43430,#43431,#43432,#43433,#43434,#43435,#43436,
#43437,#43438,#43439,#43440)) ;
#16572=EDGE_LOOP('',(#43441,#43442,#43443,#43444)) ;
#16573=EDGE_LOOP('',(#43445,#43446,#43447,#43448)) ;
#16574=EDGE_LOOP('',(#43449,#43450,#43451,#43452)) ;
#16575=EDGE_LOOP('',(#43453,#43454,#43455,#43456)) ;
#16576=EDGE_LOOP('',(#43457,#43458,#43459,#43460)) ;
#16577=EDGE_LOOP('',(#43461,#43462,#43463,#43464)) ;
#16578=EDGE_LOOP('',(#43465,#43466,#43467,#43468)) ;
#16579=EDGE_LOOP('',(#43469,#43470,#43471,#43472)) ;
#16580=EDGE_LOOP('',(#43473,#43474,#43475,#43476)) ;
#16581=EDGE_LOOP('',(#43477,#43478,#43479,#43480)) ;
#16582=EDGE_LOOP('',(#43481,#43482,#43483,#43484)) ;
#16583=EDGE_LOOP('',(#43485,#43486,#43487,#43488)) ;
#16584=EDGE_LOOP('',(#43489,#43490,#43491,#43492)) ;
#16585=EDGE_LOOP('',(#43493,#43494,#43495,#43496)) ;
#16586=EDGE_LOOP('',(#43497,#43498,#43499,#43500)) ;
#16587=EDGE_LOOP('',(#43501,#43502,#43503,#43504)) ;
#16588=EDGE_LOOP('',(#43505,#43506,#43507,#43508)) ;
#16589=EDGE_LOOP('',(#43509,#43510,#43511,#43512)) ;
#16590=EDGE_LOOP('',(#43513,#43514,#43515,#43516)) ;
#16591=EDGE_LOOP('',(#43517,#43518,#43519,#43520,#43521)) ;
#16592=EDGE_LOOP('',(#43522,#43523,#43524,#43525)) ;
#16593=EDGE_LOOP('',(#43526,#43527,#43528,#43529)) ;
#16594=EDGE_LOOP('',(#43530,#43531,#43532,#43533)) ;
#16595=EDGE_LOOP('',(#43534,#43535,#43536,#43537)) ;
#16596=EDGE_LOOP('',(#43538,#43539,#43540,#43541)) ;
#16597=EDGE_LOOP('',(#43542,#43543,#43544,#43545)) ;
#16598=EDGE_LOOP('',(#43546,#43547,#43548,#43549)) ;
#16599=EDGE_LOOP('',(#43550,#43551,#43552,#43553)) ;
#16600=EDGE_LOOP('',(#43554,#43555,#43556,#43557)) ;
#16601=EDGE_LOOP('',(#43558,#43559,#43560,#43561)) ;
#16602=EDGE_LOOP('',(#43562,#43563,#43564,#43565)) ;
#16603=EDGE_LOOP('',(#43566,#43567,#43568,#43569)) ;
#16604=EDGE_LOOP('',(#43570,#43571,#43572,#43573)) ;
#16605=EDGE_LOOP('',(#43574,#43575,#43576,#43577)) ;
#16606=EDGE_LOOP('',(#43578,#43579,#43580,#43581)) ;
#16607=EDGE_LOOP('',(#43582,#43583,#43584,#43585)) ;
#16608=EDGE_LOOP('',(#43586,#43587,#43588,#43589)) ;
#16609=EDGE_LOOP('',(#43590,#43591,#43592,#43593)) ;
#16610=EDGE_LOOP('',(#43594,#43595,#43596,#43597)) ;
#16611=EDGE_LOOP('',(#43598,#43599,#43600,#43601)) ;
#16612=EDGE_LOOP('',(#43602,#43603,#43604,#43605)) ;
#16613=EDGE_LOOP('',(#43606,#43607,#43608,#43609)) ;
#16614=EDGE_LOOP('',(#43610,#43611,#43612,#43613)) ;
#16615=EDGE_LOOP('',(#43614,#43615,#43616,#43617)) ;
#16616=EDGE_LOOP('',(#43618,#43619,#43620,#43621)) ;
#16617=EDGE_LOOP('',(#43622,#43623,#43624,#43625)) ;
#16618=EDGE_LOOP('',(#43626,#43627,#43628,#43629)) ;
#16619=EDGE_LOOP('',(#43630,#43631,#43632,#43633)) ;
#16620=EDGE_LOOP('',(#43634,#43635,#43636,#43637)) ;
#16621=EDGE_LOOP('',(#43638,#43639,#43640,#43641)) ;
#16622=EDGE_LOOP('',(#43642,#43643,#43644,#43645)) ;
#16623=EDGE_LOOP('',(#43646,#43647,#43648,#43649)) ;
#16624=EDGE_LOOP('',(#43650,#43651,#43652,#43653)) ;
#16625=EDGE_LOOP('',(#43654,#43655,#43656,#43657)) ;
#16626=EDGE_LOOP('',(#43658,#43659,#43660,#43661)) ;
#16627=EDGE_LOOP('',(#43662,#43663,#43664,#43665)) ;
#16628=EDGE_LOOP('',(#43666,#43667,#43668,#43669)) ;
#16629=EDGE_LOOP('',(#43670,#43671,#43672,#43673)) ;
#16630=EDGE_LOOP('',(#43674,#43675,#43676,#43677)) ;
#16631=EDGE_LOOP('',(#43678,#43679,#43680,#43681)) ;
#16632=EDGE_LOOP('',(#43682,#43683,#43684,#43685)) ;
#16633=EDGE_LOOP('',(#43686,#43687,#43688,#43689)) ;
#16634=EDGE_LOOP('',(#43690,#43691,#43692,#43693)) ;
#16635=EDGE_LOOP('',(#43694,#43695,#43696,#43697)) ;
#16636=EDGE_LOOP('',(#43698,#43699,#43700,#43701)) ;
#16637=EDGE_LOOP('',(#43702,#43703,#43704,#43705)) ;
#16638=EDGE_LOOP('',(#43706,#43707,#43708,#43709)) ;
#16639=EDGE_LOOP('',(#43710,#43711,#43712,#43713)) ;
#16640=EDGE_LOOP('',(#43714,#43715,#43716,#43717)) ;
#16641=EDGE_LOOP('',(#43718,#43719,#43720,#43721)) ;
#16642=EDGE_LOOP('',(#43722,#43723,#43724,#43725)) ;
#16643=EDGE_LOOP('',(#43726,#43727,#43728,#43729)) ;
#16644=EDGE_LOOP('',(#43730,#43731,#43732,#43733)) ;
#16645=EDGE_LOOP('',(#43734,#43735,#43736,#43737)) ;
#16646=EDGE_LOOP('',(#43738,#43739,#43740,#43741)) ;
#16647=EDGE_LOOP('',(#43742,#43743,#43744,#43745)) ;
#16648=EDGE_LOOP('',(#43746,#43747,#43748,#43749)) ;
#16649=EDGE_LOOP('',(#43750,#43751,#43752,#43753)) ;
#16650=EDGE_LOOP('',(#43754,#43755,#43756,#43757)) ;
#16651=EDGE_LOOP('',(#43758,#43759,#43760,#43761)) ;
#16652=EDGE_LOOP('',(#43762,#43763,#43764,#43765)) ;
#16653=EDGE_LOOP('',(#43766,#43767,#43768,#43769)) ;
#16654=EDGE_LOOP('',(#43770,#43771,#43772,#43773)) ;
#16655=EDGE_LOOP('',(#43774,#43775,#43776,#43777)) ;
#16656=EDGE_LOOP('',(#43778,#43779,#43780,#43781)) ;
#16657=EDGE_LOOP('',(#43782,#43783,#43784,#43785)) ;
#16658=EDGE_LOOP('',(#43786,#43787,#43788,#43789)) ;
#16659=EDGE_LOOP('',(#43790,#43791,#43792,#43793)) ;
#16660=EDGE_LOOP('',(#43794,#43795,#43796,#43797)) ;
#16661=EDGE_LOOP('',(#43798,#43799,#43800,#43801)) ;
#16662=EDGE_LOOP('',(#43802,#43803,#43804,#43805)) ;
#16663=EDGE_LOOP('',(#43806,#43807,#43808,#43809)) ;
#16664=EDGE_LOOP('',(#43810,#43811,#43812,#43813)) ;
#16665=EDGE_LOOP('',(#43814,#43815,#43816,#43817)) ;
#16666=EDGE_LOOP('',(#43818,#43819,#43820,#43821)) ;
#16667=EDGE_LOOP('',(#43822,#43823,#43824,#43825)) ;
#16668=EDGE_LOOP('',(#43826,#43827,#43828,#43829)) ;
#16669=EDGE_LOOP('',(#43830,#43831,#43832,#43833)) ;
#16670=EDGE_LOOP('',(#43834,#43835,#43836,#43837)) ;
#16671=EDGE_LOOP('',(#43838,#43839,#43840,#43841)) ;
#16672=EDGE_LOOP('',(#43842,#43843,#43844,#43845)) ;
#16673=EDGE_LOOP('',(#43846,#43847,#43848,#43849)) ;
#16674=EDGE_LOOP('',(#43850,#43851,#43852,#43853)) ;
#16675=EDGE_LOOP('',(#43854,#43855,#43856,#43857)) ;
#16676=EDGE_LOOP('',(#43858,#43859,#43860,#43861)) ;
#16677=EDGE_LOOP('',(#43862,#43863,#43864,#43865)) ;
#16678=EDGE_LOOP('',(#43866,#43867,#43868,#43869)) ;
#16679=EDGE_LOOP('',(#43870,#43871,#43872,#43873)) ;
#16680=EDGE_LOOP('',(#43874,#43875,#43876,#43877)) ;
#16681=EDGE_LOOP('',(#43878,#43879,#43880,#43881)) ;
#16682=EDGE_LOOP('',(#43882,#43883,#43884,#43885)) ;
#16683=EDGE_LOOP('',(#43886,#43887,#43888,#43889)) ;
#16684=EDGE_LOOP('',(#43890,#43891,#43892,#43893)) ;
#16685=EDGE_LOOP('',(#43894,#43895,#43896,#43897)) ;
#16686=EDGE_LOOP('',(#43898,#43899,#43900,#43901)) ;
#16687=EDGE_LOOP('',(#43902,#43903,#43904,#43905)) ;
#16688=EDGE_LOOP('',(#43906,#43907,#43908,#43909)) ;
#16689=EDGE_LOOP('',(#43910,#43911,#43912,#43913)) ;
#16690=EDGE_LOOP('',(#43914,#43915,#43916,#43917)) ;
#16691=EDGE_LOOP('',(#43918,#43919,#43920,#43921)) ;
#16692=EDGE_LOOP('',(#43922,#43923,#43924,#43925)) ;
#16693=EDGE_LOOP('',(#43926,#43927,#43928,#43929)) ;
#16694=EDGE_LOOP('',(#43930,#43931,#43932,#43933)) ;
#16695=EDGE_LOOP('',(#43934,#43935,#43936,#43937)) ;
#16696=EDGE_LOOP('',(#43938,#43939,#43940,#43941)) ;
#16697=EDGE_LOOP('',(#43942,#43943,#43944,#43945)) ;
#16698=EDGE_LOOP('',(#43946,#43947,#43948,#43949)) ;
#16699=EDGE_LOOP('',(#43950,#43951,#43952,#43953)) ;
#16700=EDGE_LOOP('',(#43954,#43955,#43956,#43957)) ;
#16701=EDGE_LOOP('',(#43958,#43959,#43960,#43961)) ;
#16702=EDGE_LOOP('',(#43962,#43963,#43964,#43965)) ;
#16703=EDGE_LOOP('',(#43966,#43967,#43968,#43969)) ;
#16704=EDGE_LOOP('',(#43970,#43971,#43972,#43973)) ;
#16705=EDGE_LOOP('',(#43974,#43975,#43976,#43977)) ;
#16706=EDGE_LOOP('',(#43978,#43979,#43980,#43981)) ;
#16707=EDGE_LOOP('',(#43982,#43983,#43984,#43985)) ;
#16708=EDGE_LOOP('',(#43986,#43987,#43988,#43989)) ;
#16709=EDGE_LOOP('',(#43990,#43991,#43992,#43993)) ;
#16710=EDGE_LOOP('',(#43994,#43995,#43996,#43997)) ;
#16711=EDGE_LOOP('',(#43998,#43999,#44000,#44001)) ;
#16712=EDGE_LOOP('',(#44002,#44003,#44004,#44005)) ;
#19127=CIRCLE('',#54044,3.) ;
#19128=CIRCLE('',#54045,1.) ;
#19129=CIRCLE('',#54046,3.96824583655185) ;
#19130=CIRCLE('',#54049,4.) ;
#19131=CIRCLE('',#54050,1.) ;
#19132=CIRCLE('',#54051,3.) ;
#19133=CIRCLE('',#54054,2.) ;
#19134=CIRCLE('',#54056,2.) ;
#19135=CIRCLE('',#54058,4.95) ;
#19136=CIRCLE('',#54059,5.1) ;
#19137=CIRCLE('',#54062,0.350000000000003) ;
#19138=CIRCLE('',#54063,0.500000000000003) ;
#19139=CIRCLE('',#54066,4.95) ;
#19140=CIRCLE('',#54067,5.1) ;
#19141=CIRCLE('',#54070,0.350000000000003) ;
#19142=CIRCLE('',#54071,0.500000000000003) ;
#19143=CIRCLE('',#54074,4.95) ;
#19144=CIRCLE('',#54075,5.1) ;
#19145=CIRCLE('',#54078,0.350000000000003) ;
#19146=CIRCLE('',#54079,0.500000000000003) ;
#19147=CIRCLE('',#54082,4.95) ;
#19148=CIRCLE('',#54083,5.1) ;
#19149=CIRCLE('',#54086,0.350000000000003) ;
#19150=CIRCLE('',#54087,0.500000000000003) ;
#19151=CIRCLE('',#54090,4.95) ;
#19152=CIRCLE('',#54091,5.1) ;
#19153=CIRCLE('',#54094,0.350000000000003) ;
#19154=CIRCLE('',#54095,0.500000000000003) ;
#19155=CIRCLE('',#54098,4.95) ;
#19156=CIRCLE('',#54099,5.1) ;
#19157=CIRCLE('',#54102,0.350000000000003) ;
#19158=CIRCLE('',#54103,0.500000000000003) ;
#19159=CIRCLE('',#54106,4.95) ;
#19160=CIRCLE('',#54107,5.1) ;
#19161=CIRCLE('',#54110,0.350000000000003) ;
#19162=CIRCLE('',#54111,0.500000000000003) ;
#19163=CIRCLE('',#54114,4.95) ;
#19164=CIRCLE('',#54115,5.1) ;
#19165=CIRCLE('',#54118,0.350000000000003) ;
#19166=CIRCLE('',#54119,0.500000000000003) ;
#19167=CIRCLE('',#54122,4.95) ;
#19168=CIRCLE('',#54123,5.1) ;
#19169=CIRCLE('',#54126,0.350000000000003) ;
#19170=CIRCLE('',#54127,0.500000000000003) ;
#19171=CIRCLE('',#54130,4.95) ;
#19172=CIRCLE('',#54131,5.1) ;
#19173=CIRCLE('',#54134,0.350000000000003) ;
#19174=CIRCLE('',#54135,0.500000000000003) ;
#19175=CIRCLE('',#54138,4.95) ;
#19176=CIRCLE('',#54139,5.1) ;
#19177=CIRCLE('',#54142,0.500000000000003) ;
#19178=CIRCLE('',#54143,0.350000000000003) ;
#19179=CIRCLE('',#54146,5.1) ;
#19180=CIRCLE('',#54147,4.95) ;
#19181=CIRCLE('',#54150,0.500000000000003) ;
#19182=CIRCLE('',#54151,0.350000000000003) ;
#19183=CIRCLE('',#54154,5.1) ;
#19184=CIRCLE('',#54155,4.95) ;
#19185=CIRCLE('',#54158,0.500000000000003) ;
#19186=CIRCLE('',#54159,0.350000000000003) ;
#19187=CIRCLE('',#54162,5.1) ;
#19188=CIRCLE('',#54163,4.95) ;
#19189=CIRCLE('',#54166,0.500000000000003) ;
#19190=CIRCLE('',#54167,0.350000000000003) ;
#19191=CIRCLE('',#54170,5.1) ;
#19192=CIRCLE('',#54171,4.95) ;
#19193=CIRCLE('',#54174,0.500000000000003) ;
#19194=CIRCLE('',#54175,0.350000000000003) ;
#19195=CIRCLE('',#54178,5.1) ;
#19196=CIRCLE('',#54179,4.95) ;
#19197=CIRCLE('',#54182,0.500000000000003) ;
#19198=CIRCLE('',#54183,0.350000000000003) ;
#19199=CIRCLE('',#54186,5.1) ;
#19200=CIRCLE('',#54187,4.95) ;
#19201=CIRCLE('',#54190,0.500000000000003) ;
#19202=CIRCLE('',#54191,0.350000000000003) ;
#19203=CIRCLE('',#54194,5.1) ;
#19204=CIRCLE('',#54195,4.95) ;
#19205=CIRCLE('',#54198,0.500000000000003) ;
#19206=CIRCLE('',#54199,0.350000000000003) ;
#19207=CIRCLE('',#54202,5.1) ;
#19208=CIRCLE('',#54203,4.95) ;
#19209=CIRCLE('',#54206,0.500000000000003) ;
#19210=CIRCLE('',#54207,0.350000000000003) ;
#19211=CIRCLE('',#54210,5.1) ;
#19212=CIRCLE('',#54211,4.95) ;
#19213=CIRCLE('',#54214,0.500000000000003) ;
#19214=CIRCLE('',#54215,0.350000000000003) ;
#19215=CIRCLE('',#54219,0.500000000000003) ;
#19216=CIRCLE('',#54222,5.1) ;
#19217=CIRCLE('',#54225,0.500000000000003) ;
#19218=CIRCLE('',#54228,5.1) ;
#19219=CIRCLE('',#54231,0.500000000000003) ;
#19220=CIRCLE('',#54234,5.1) ;
#19221=CIRCLE('',#54237,0.500000000000003) ;
#19222=CIRCLE('',#54240,5.1) ;
#19223=CIRCLE('',#54243,0.500000000000003) ;
#19224=CIRCLE('',#54246,5.1) ;
#19225=CIRCLE('',#54249,0.500000000000003) ;
#19226=CIRCLE('',#54252,5.1) ;
#19227=CIRCLE('',#54255,0.500000000000003) ;
#19228=CIRCLE('',#54258,5.1) ;
#19229=CIRCLE('',#54261,0.500000000000003) ;
#19230=CIRCLE('',#54264,5.1) ;
#19231=CIRCLE('',#54267,0.500000000000003) ;
#19232=CIRCLE('',#54270,5.1) ;
#19233=CIRCLE('',#54273,0.500000000000003) ;
#19234=CIRCLE('',#54276,5.1) ;
#19235=CIRCLE('',#54278,4.95) ;
#19236=CIRCLE('',#54280,4.95) ;
#19237=CIRCLE('',#54282,4.95) ;
#19238=CIRCLE('',#54284,4.95) ;
#19239=CIRCLE('',#54286,4.95) ;
#19240=CIRCLE('',#54288,4.95) ;
#19241=CIRCLE('',#54290,4.95) ;
#19242=CIRCLE('',#54292,4.95) ;
#19243=CIRCLE('',#54294,4.95) ;
#19244=CIRCLE('',#54296,4.95) ;
#19245=CIRCLE('',#54298,4.95) ;
#19246=CIRCLE('',#54300,4.95) ;
#19247=CIRCLE('',#54302,4.95) ;
#19248=CIRCLE('',#54304,4.95) ;
#19249=CIRCLE('',#54306,4.95) ;
#19250=CIRCLE('',#54308,4.95) ;
#19251=CIRCLE('',#54310,4.95) ;
#19252=CIRCLE('',#54312,4.95) ;
#19253=CIRCLE('',#54314,4.95) ;
#19254=CIRCLE('',#54315,4.95) ;
#19255=CIRCLE('',#54317,0.15) ;
#19256=CIRCLE('',#54318,4.95) ;
#19257=CIRCLE('',#54321,0.15) ;
#19258=CIRCLE('',#54322,4.95) ;
#19259=CIRCLE('',#54323,4.95) ;
#19260=CIRCLE('',#54324,4.95) ;
#19261=CIRCLE('',#54325,4.95) ;
#19262=CIRCLE('',#54326,4.95) ;
#19263=CIRCLE('',#54327,4.95) ;
#19264=CIRCLE('',#54328,4.95) ;
#19265=CIRCLE('',#54329,4.95) ;
#19266=CIRCLE('',#54330,4.95) ;
#19267=CIRCLE('',#54331,4.95) ;
#19268=CIRCLE('',#54332,4.95) ;
#19269=CIRCLE('',#54333,4.95) ;
#19270=CIRCLE('',#54334,4.95) ;
#19271=CIRCLE('',#54335,4.95) ;
#19272=CIRCLE('',#54336,4.95) ;
#19273=CIRCLE('',#54337,4.95) ;
#19274=CIRCLE('',#54338,4.95) ;
#19275=CIRCLE('',#54339,4.95) ;
#19276=CIRCLE('',#54340,4.95) ;
#19277=CIRCLE('',#54341,4.95) ;
#19278=CIRCLE('',#54342,4.95) ;
#19279=CIRCLE('',#54343,4.95) ;
#19280=CIRCLE('',#54344,4.95) ;
#19281=CIRCLE('',#54345,4.95) ;
#19282=CIRCLE('',#54346,4.95) ;
#19283=CIRCLE('',#54347,4.95) ;
#19284=CIRCLE('',#54348,4.95) ;
#19285=CIRCLE('',#54349,4.95) ;
#19286=CIRCLE('',#54350,4.95) ;
#19287=CIRCLE('',#54351,4.95) ;
#19288=CIRCLE('',#54352,4.95) ;
#19289=CIRCLE('',#54353,4.95) ;
#19290=CIRCLE('',#54354,4.95) ;
#19291=CIRCLE('',#54355,4.95) ;
#19292=CIRCLE('',#54356,4.95) ;
#19293=CIRCLE('',#54357,4.95) ;
#19294=CIRCLE('',#54358,4.95) ;
#19295=CIRCLE('',#54359,4.95) ;
#19296=CIRCLE('',#54360,4.95) ;
#19297=CIRCLE('',#54361,4.95) ;
#19298=CIRCLE('',#54362,4.95) ;
#19299=CIRCLE('',#54364,0.350000000000003) ;
#19300=CIRCLE('',#54366,0.350000000000003) ;
#19301=CIRCLE('',#54368,0.350000000000003) ;
#19302=CIRCLE('',#54370,0.350000000000003) ;
#19303=CIRCLE('',#54372,0.350000000000003) ;
#19304=CIRCLE('',#54374,0.350000000000003) ;
#19305=CIRCLE('',#54376,0.350000000000003) ;
#19306=CIRCLE('',#54378,0.350000000000003) ;
#19307=CIRCLE('',#54380,0.350000000000003) ;
#19308=CIRCLE('',#54382,0.350000000000003) ;
#19309=CIRCLE('',#54384,0.350000000000003) ;
#19310=CIRCLE('',#54386,0.350000000000003) ;
#19311=CIRCLE('',#54388,0.350000000000003) ;
#19312=CIRCLE('',#54390,0.350000000000003) ;
#19313=CIRCLE('',#54392,0.350000000000003) ;
#19314=CIRCLE('',#54394,0.350000000000003) ;
#19315=CIRCLE('',#54396,0.350000000000003) ;
#19316=CIRCLE('',#54398,0.350000000000003) ;
#19317=CIRCLE('',#54400,0.350000000000003) ;
#19318=CIRCLE('',#54402,0.350000000000003) ;
#19319=CIRCLE('',#54404,5.1) ;
#19320=CIRCLE('',#54449,5.1) ;
#19321=CIRCLE('',#54452,0.500000000000003) ;
#19322=CIRCLE('',#54455,5.1) ;
#19323=CIRCLE('',#54458,0.500000000000003) ;
#19324=CIRCLE('',#54461,5.1) ;
#19325=CIRCLE('',#54464,0.500000000000003) ;
#19326=CIRCLE('',#54467,5.1) ;
#19327=CIRCLE('',#54470,0.500000000000003) ;
#19328=CIRCLE('',#54473,5.1) ;
#19329=CIRCLE('',#54476,0.500000000000003) ;
#19330=CIRCLE('',#54479,5.1) ;
#19331=CIRCLE('',#54482,0.500000000000003) ;
#19332=CIRCLE('',#54485,5.1) ;
#19333=CIRCLE('',#54488,0.500000000000003) ;
#19334=CIRCLE('',#54491,5.1) ;
#19335=CIRCLE('',#54494,0.500000000000003) ;
#19336=CIRCLE('',#54497,5.1) ;
#19337=CIRCLE('',#54500,0.500000000000003) ;
#19338=CIRCLE('',#54502,0.500000000000003) ;
#23033=VERTEX_POINT('',#101747) ;
#23034=VERTEX_POINT('',#101749) ;
#23035=VERTEX_POINT('',#101753) ;
#23036=VERTEX_POINT('',#101771) ;
#23037=VERTEX_POINT('',#101773) ;
#23038=VERTEX_POINT('',#101777) ;
#23039=VERTEX_POINT('',#101795) ;
#23040=VERTEX_POINT('',#101798) ;
#23041=VERTEX_POINT('',#101880) ;
#23042=VERTEX_POINT('',#101886) ;
#23043=VERTEX_POINT('',#101987) ;
#23044=VERTEX_POINT('',#101993) ;
#23045=VERTEX_POINT('',#102015) ;
#23046=VERTEX_POINT('',#102016) ;
#23047=VERTEX_POINT('',#102018) ;
#23048=VERTEX_POINT('',#102033) ;
#23049=VERTEX_POINT('',#102050) ;
#23050=VERTEX_POINT('',#102052) ;
#23051=VERTEX_POINT('',#102071) ;
#23052=VERTEX_POINT('',#102073) ;
#23053=VERTEX_POINT('',#102092) ;
#23054=VERTEX_POINT('',#102094) ;
#23055=VERTEX_POINT('',#102111) ;
#23056=VERTEX_POINT('',#102113) ;
#23057=VERTEX_POINT('',#102130) ;
#23058=VERTEX_POINT('',#102132) ;
#23059=VERTEX_POINT('',#102151) ;
#23060=VERTEX_POINT('',#102153) ;
#23061=VERTEX_POINT('',#102172) ;
#23062=VERTEX_POINT('',#102174) ;
#23063=VERTEX_POINT('',#102191) ;
#23064=VERTEX_POINT('',#102193) ;
#23065=VERTEX_POINT('',#102210) ;
#23066=VERTEX_POINT('',#102212) ;
#23067=VERTEX_POINT('',#102231) ;
#23068=VERTEX_POINT('',#102233) ;
#23069=VERTEX_POINT('',#102252) ;
#23070=VERTEX_POINT('',#102254) ;
#23071=VERTEX_POINT('',#102271) ;
#23072=VERTEX_POINT('',#102273) ;
#23073=VERTEX_POINT('',#102290) ;
#23074=VERTEX_POINT('',#102292) ;
#23075=VERTEX_POINT('',#102311) ;
#23076=VERTEX_POINT('',#102313) ;
#23077=VERTEX_POINT('',#102332) ;
#23078=VERTEX_POINT('',#102334) ;
#23079=VERTEX_POINT('',#102351) ;
#23080=VERTEX_POINT('',#102353) ;
#23081=VERTEX_POINT('',#102370) ;
#23082=VERTEX_POINT('',#102372) ;
#23083=VERTEX_POINT('',#102391) ;
#23084=VERTEX_POINT('',#102393) ;
#23085=VERTEX_POINT('',#102412) ;
#23086=VERTEX_POINT('',#102414) ;
#23087=VERTEX_POINT('',#102431) ;
#23088=VERTEX_POINT('',#102433) ;
#23089=VERTEX_POINT('',#102450) ;
#23090=VERTEX_POINT('',#102452) ;
#23091=VERTEX_POINT('',#102471) ;
#23092=VERTEX_POINT('',#102473) ;
#23093=VERTEX_POINT('',#102492) ;
#23094=VERTEX_POINT('',#102494) ;
#23095=VERTEX_POINT('',#102511) ;
#23096=VERTEX_POINT('',#102513) ;
#23097=VERTEX_POINT('',#102530) ;
#23098=VERTEX_POINT('',#102532) ;
#23099=VERTEX_POINT('',#102551) ;
#23100=VERTEX_POINT('',#102553) ;
#23101=VERTEX_POINT('',#102572) ;
#23102=VERTEX_POINT('',#102574) ;
#23103=VERTEX_POINT('',#102591) ;
#23104=VERTEX_POINT('',#102593) ;
#23105=VERTEX_POINT('',#102610) ;
#23106=VERTEX_POINT('',#102612) ;
#23107=VERTEX_POINT('',#102631) ;
#23108=VERTEX_POINT('',#102633) ;
#23109=VERTEX_POINT('',#102652) ;
#23110=VERTEX_POINT('',#102654) ;
#23111=VERTEX_POINT('',#102671) ;
#23112=VERTEX_POINT('',#102673) ;
#23113=VERTEX_POINT('',#102690) ;
#23114=VERTEX_POINT('',#102692) ;
#23115=VERTEX_POINT('',#102711) ;
#23116=VERTEX_POINT('',#102713) ;
#23117=VERTEX_POINT('',#102732) ;
#23118=VERTEX_POINT('',#102734) ;
#23119=VERTEX_POINT('',#102751) ;
#23120=VERTEX_POINT('',#102753) ;
#23121=VERTEX_POINT('',#102770) ;
#23122=VERTEX_POINT('',#102772) ;
#23123=VERTEX_POINT('',#102791) ;
#23124=VERTEX_POINT('',#102793) ;
#23125=VERTEX_POINT('',#102812) ;
#23126=VERTEX_POINT('',#102814) ;
#23127=VERTEX_POINT('',#102831) ;
#23128=VERTEX_POINT('',#102833) ;
#23129=VERTEX_POINT('',#102850) ;
#23130=VERTEX_POINT('',#102852) ;
#23131=VERTEX_POINT('',#102871) ;
#23132=VERTEX_POINT('',#102873) ;
#23133=VERTEX_POINT('',#102892) ;
#23134=VERTEX_POINT('',#102894) ;
#23135=VERTEX_POINT('',#102911) ;
#23136=VERTEX_POINT('',#102913) ;
#23137=VERTEX_POINT('',#102930) ;
#23138=VERTEX_POINT('',#102932) ;
#23139=VERTEX_POINT('',#102951) ;
#23140=VERTEX_POINT('',#102953) ;
#23141=VERTEX_POINT('',#102972) ;
#23142=VERTEX_POINT('',#102974) ;
#23143=VERTEX_POINT('',#102991) ;
#23144=VERTEX_POINT('',#102993) ;
#23145=VERTEX_POINT('',#103010) ;
#23146=VERTEX_POINT('',#103012) ;
#23147=VERTEX_POINT('',#103031) ;
#23148=VERTEX_POINT('',#103033) ;
#23149=VERTEX_POINT('',#103052) ;
#23150=VERTEX_POINT('',#103054) ;
#23151=VERTEX_POINT('',#103071) ;
#23152=VERTEX_POINT('',#103073) ;
#23153=VERTEX_POINT('',#103090) ;
#23154=VERTEX_POINT('',#103092) ;
#23155=VERTEX_POINT('',#103111) ;
#23156=VERTEX_POINT('',#103113) ;
#23157=VERTEX_POINT('',#103132) ;
#23158=VERTEX_POINT('',#103134) ;
#23159=VERTEX_POINT('',#103151) ;
#23160=VERTEX_POINT('',#103153) ;
#23161=VERTEX_POINT('',#103170) ;
#23162=VERTEX_POINT('',#103172) ;
#23163=VERTEX_POINT('',#103191) ;
#23164=VERTEX_POINT('',#103193) ;
#23165=VERTEX_POINT('',#103212) ;
#23166=VERTEX_POINT('',#103214) ;
#23167=VERTEX_POINT('',#103231) ;
#23168=VERTEX_POINT('',#103233) ;
#23169=VERTEX_POINT('',#103250) ;
#23170=VERTEX_POINT('',#103252) ;
#23171=VERTEX_POINT('',#103271) ;
#23172=VERTEX_POINT('',#103273) ;
#23173=VERTEX_POINT('',#103292) ;
#23174=VERTEX_POINT('',#103294) ;
#23175=VERTEX_POINT('',#103311) ;
#23176=VERTEX_POINT('',#103313) ;
#23177=VERTEX_POINT('',#103330) ;
#23178=VERTEX_POINT('',#103332) ;
#23179=VERTEX_POINT('',#103351) ;
#23180=VERTEX_POINT('',#103353) ;
#23181=VERTEX_POINT('',#103372) ;
#23182=VERTEX_POINT('',#103374) ;
#23183=VERTEX_POINT('',#103391) ;
#23184=VERTEX_POINT('',#103393) ;
#23185=VERTEX_POINT('',#103410) ;
#23186=VERTEX_POINT('',#103412) ;
#23187=VERTEX_POINT('',#103431) ;
#23188=VERTEX_POINT('',#103433) ;
#23189=VERTEX_POINT('',#103452) ;
#23190=VERTEX_POINT('',#103454) ;
#23191=VERTEX_POINT('',#103471) ;
#23192=VERTEX_POINT('',#103473) ;
#23193=VERTEX_POINT('',#103490) ;
#23194=VERTEX_POINT('',#103492) ;
#23195=VERTEX_POINT('',#103511) ;
#23196=VERTEX_POINT('',#103513) ;
#23197=VERTEX_POINT('',#103532) ;
#23198=VERTEX_POINT('',#103534) ;
#23199=VERTEX_POINT('',#103551) ;
#23200=VERTEX_POINT('',#103553) ;
#23201=VERTEX_POINT('',#103570) ;
#23202=VERTEX_POINT('',#103572) ;
#23203=VERTEX_POINT('',#103591) ;
#23204=VERTEX_POINT('',#103593) ;
#23205=VERTEX_POINT('',#103615) ;
#23206=VERTEX_POINT('',#103617) ;
#23207=VERTEX_POINT('',#103621) ;
#23208=VERTEX_POINT('',#103625) ;
#23209=VERTEX_POINT('',#103629) ;
#23210=VERTEX_POINT('',#103633) ;
#23211=VERTEX_POINT('',#103637) ;
#23212=VERTEX_POINT('',#103641) ;
#23213=VERTEX_POINT('',#103645) ;
#23214=VERTEX_POINT('',#103649) ;
#23215=VERTEX_POINT('',#103653) ;
#23216=VERTEX_POINT('',#103657) ;
#23217=VERTEX_POINT('',#103661) ;
#23218=VERTEX_POINT('',#103665) ;
#23219=VERTEX_POINT('',#103669) ;
#23220=VERTEX_POINT('',#103673) ;
#23221=VERTEX_POINT('',#103677) ;
#23222=VERTEX_POINT('',#103681) ;
#23223=VERTEX_POINT('',#103685) ;
#23224=VERTEX_POINT('',#103689) ;
#23225=VERTEX_POINT('',#103693) ;
#23226=VERTEX_POINT('',#103697) ;
#23227=VERTEX_POINT('',#103701) ;
#23228=VERTEX_POINT('',#103705) ;
#23229=VERTEX_POINT('',#103709) ;
#23230=VERTEX_POINT('',#103713) ;
#23231=VERTEX_POINT('',#103717) ;
#23232=VERTEX_POINT('',#103721) ;
#23233=VERTEX_POINT('',#103725) ;
#23234=VERTEX_POINT('',#103729) ;
#23235=VERTEX_POINT('',#103733) ;
#23236=VERTEX_POINT('',#103737) ;
#23237=VERTEX_POINT('',#103741) ;
#23238=VERTEX_POINT('',#103745) ;
#23239=VERTEX_POINT('',#103749) ;
#23240=VERTEX_POINT('',#103753) ;
#23241=VERTEX_POINT('',#103757) ;
#23242=VERTEX_POINT('',#103761) ;
#23243=VERTEX_POINT('',#103765) ;
#23244=VERTEX_POINT('',#103769) ;
#23245=VERTEX_POINT('',#103773) ;
#23246=VERTEX_POINT('',#103813) ;
#23247=VERTEX_POINT('',#103821) ;
#23248=VERTEX_POINT('',#103823) ;
#23249=VERTEX_POINT('',#103825) ;
#23250=VERTEX_POINT('',#103827) ;
#23251=VERTEX_POINT('',#103829) ;
#23252=VERTEX_POINT('',#103831) ;
#23253=VERTEX_POINT('',#103833) ;
#23254=VERTEX_POINT('',#103835) ;
#23255=VERTEX_POINT('',#103837) ;
#23256=VERTEX_POINT('',#103839) ;
#23257=VERTEX_POINT('',#103841) ;
#23258=VERTEX_POINT('',#103843) ;
#23259=VERTEX_POINT('',#103845) ;
#23260=VERTEX_POINT('',#103847) ;
#23261=VERTEX_POINT('',#103849) ;
#23262=VERTEX_POINT('',#103851) ;
#23263=VERTEX_POINT('',#103853) ;
#23264=VERTEX_POINT('',#103855) ;
#23265=VERTEX_POINT('',#103857) ;
#23266=VERTEX_POINT('',#103859) ;
#23267=VERTEX_POINT('',#103861) ;
#23268=VERTEX_POINT('',#103863) ;
#23269=VERTEX_POINT('',#103865) ;
#23270=VERTEX_POINT('',#103867) ;
#23271=VERTEX_POINT('',#103869) ;
#23272=VERTEX_POINT('',#103871) ;
#23273=VERTEX_POINT('',#103873) ;
#23274=VERTEX_POINT('',#103875) ;
#23275=VERTEX_POINT('',#103877) ;
#23276=VERTEX_POINT('',#103879) ;
#23277=VERTEX_POINT('',#103881) ;
#23278=VERTEX_POINT('',#103883) ;
#23279=VERTEX_POINT('',#103885) ;
#23280=VERTEX_POINT('',#103887) ;
#23281=VERTEX_POINT('',#103889) ;
#23282=VERTEX_POINT('',#103891) ;
#23283=VERTEX_POINT('',#103893) ;
#23284=VERTEX_POINT('',#103895) ;
#23285=VERTEX_POINT('',#103897) ;
#23286=VERTEX_POINT('',#103899) ;
#23287=VERTEX_POINT('',#103901) ;
#23288=VERTEX_POINT('',#103905) ;
#23289=VERTEX_POINT('',#103907) ;
#23290=VERTEX_POINT('',#103911) ;
#23291=VERTEX_POINT('',#103913) ;
#23292=VERTEX_POINT('',#103917) ;
#23293=VERTEX_POINT('',#103919) ;
#23294=VERTEX_POINT('',#103923) ;
#23295=VERTEX_POINT('',#103925) ;
#23296=VERTEX_POINT('',#103929) ;
#23297=VERTEX_POINT('',#103931) ;
#23298=VERTEX_POINT('',#103935) ;
#23299=VERTEX_POINT('',#103937) ;
#23300=VERTEX_POINT('',#103941) ;
#23301=VERTEX_POINT('',#103943) ;
#23302=VERTEX_POINT('',#103947) ;
#23303=VERTEX_POINT('',#103949) ;
#23304=VERTEX_POINT('',#103953) ;
#23305=VERTEX_POINT('',#103955) ;
#23306=VERTEX_POINT('',#103959) ;
#23307=VERTEX_POINT('',#103961) ;
#23308=VERTEX_POINT('',#103965) ;
#23309=VERTEX_POINT('',#103967) ;
#23310=VERTEX_POINT('',#103971) ;
#23311=VERTEX_POINT('',#103973) ;
#23312=VERTEX_POINT('',#103977) ;
#23313=VERTEX_POINT('',#103979) ;
#23314=VERTEX_POINT('',#103983) ;
#23315=VERTEX_POINT('',#103985) ;
#23316=VERTEX_POINT('',#103989) ;
#23317=VERTEX_POINT('',#103991) ;
#23318=VERTEX_POINT('',#103995) ;
#23319=VERTEX_POINT('',#103997) ;
#23320=VERTEX_POINT('',#104001) ;
#23321=VERTEX_POINT('',#104003) ;
#23322=VERTEX_POINT('',#104007) ;
#23323=VERTEX_POINT('',#104009) ;
#23324=VERTEX_POINT('',#104013) ;
#23325=VERTEX_POINT('',#104015) ;
#23326=VERTEX_POINT('',#104019) ;
#23327=VERTEX_POINT('',#104021) ;
#23328=VERTEX_POINT('',#104025) ;
#23329=VERTEX_POINT('',#104040) ;
#23330=VERTEX_POINT('',#104057) ;
#23331=VERTEX_POINT('',#104076) ;
#23332=VERTEX_POINT('',#104109) ;
#23333=VERTEX_POINT('',#104160) ;
#23334=VERTEX_POINT('',#104161) ;
#23335=VERTEX_POINT('',#104257) ;
#23336=VERTEX_POINT('',#104258) ;
#23337=VERTEX_POINT('',#104354) ;
#23338=VERTEX_POINT('',#104355) ;
#23339=VERTEX_POINT('',#104451) ;
#23340=VERTEX_POINT('',#104452) ;
#23341=VERTEX_POINT('',#104548) ;
#23342=VERTEX_POINT('',#104549) ;
#23343=VERTEX_POINT('',#104645) ;
#23344=VERTEX_POINT('',#104646) ;
#23345=VERTEX_POINT('',#104742) ;
#23346=VERTEX_POINT('',#104743) ;
#23347=VERTEX_POINT('',#104839) ;
#23348=VERTEX_POINT('',#104840) ;
#23349=VERTEX_POINT('',#105032) ;
#23350=VERTEX_POINT('',#105049) ;
#23351=VERTEX_POINT('',#105071) ;
#23352=VERTEX_POINT('',#105088) ;
#23353=VERTEX_POINT('',#105110) ;
#23354=VERTEX_POINT('',#105127) ;
#23355=VERTEX_POINT('',#105149) ;
#23356=VERTEX_POINT('',#105166) ;
#23357=VERTEX_POINT('',#105188) ;
#23358=VERTEX_POINT('',#105205) ;
#23359=VERTEX_POINT('',#105227) ;
#23360=VERTEX_POINT('',#105244) ;
#23361=VERTEX_POINT('',#105266) ;
#23362=VERTEX_POINT('',#105283) ;
#23363=VERTEX_POINT('',#105305) ;
#23364=VERTEX_POINT('',#105322) ;
#23365=VERTEX_POINT('',#105344) ;
#23366=VERTEX_POINT('',#105361) ;
#29660=EDGE_CURVE('',#23033,#23033,#19127,.T.) ;
#29661=EDGE_CURVE('',#23033,#23034,#19128,.T.) ;
#29662=EDGE_CURVE('',#23034,#23034,#19129,.T.) ;
#29663=EDGE_CURVE('',#23035,#23035,#1361,.T.) ;
#29664=EDGE_CURVE('',#23036,#23036,#19130,.T.) ;
#29665=EDGE_CURVE('',#23036,#23037,#19131,.T.) ;
#29666=EDGE_CURVE('',#23037,#23037,#19132,.T.) ;
#29667=EDGE_CURVE('',#23038,#23038,#1362,.T.) ;
#29668=EDGE_CURVE('',#23039,#23039,#19133,.T.) ;
#29669=EDGE_CURVE('',#23040,#23040,#19134,.T.) ;
#29670=EDGE_CURVE('',#23035,#23041,#1363,.T.) ;
#29671=EDGE_CURVE('',#23041,#23042,#1364,.T.) ;
#29672=EDGE_CURVE('',#23042,#23041,#1365,.T.) ;
#29673=EDGE_CURVE('',#23038,#23043,#1366,.T.) ;
#29674=EDGE_CURVE('',#23043,#23044,#1367,.T.) ;
#29675=EDGE_CURVE('',#23044,#23043,#1368,.T.) ;
#29676=EDGE_CURVE('',#23045,#23046,#19135,.T.) ;
#29677=EDGE_CURVE('',#23045,#23047,#1369,.T.) ;
#29678=EDGE_CURVE('',#23047,#23048,#19136,.T.) ;
#29679=EDGE_CURVE('',#23046,#23048,#1370,.T.) ;
#29680=EDGE_CURVE('',#23045,#23049,#5754,.T.) ;
#29681=EDGE_CURVE('',#23049,#23050,#1371,.T.) ;
#29682=EDGE_CURVE('',#23050,#23047,#5755,.T.) ;
#29683=EDGE_CURVE('',#23049,#23051,#19137,.T.) ;
#29684=EDGE_CURVE('',#23051,#23052,#1372,.T.) ;
#29685=EDGE_CURVE('',#23052,#23050,#19138,.T.) ;
#29686=EDGE_CURVE('',#23051,#23053,#5756,.T.) ;
#29687=EDGE_CURVE('',#23053,#23054,#1373,.T.) ;
#29688=EDGE_CURVE('',#23054,#23052,#5757,.T.) ;
#29689=EDGE_CURVE('',#23055,#23053,#19139,.T.) ;
#29690=EDGE_CURVE('',#23055,#23056,#1374,.T.) ;
#29691=EDGE_CURVE('',#23056,#23054,#19140,.T.) ;
#29692=EDGE_CURVE('',#23055,#23057,#5758,.T.) ;
#29693=EDGE_CURVE('',#23057,#23058,#1375,.T.) ;
#29694=EDGE_CURVE('',#23058,#23056,#5759,.T.) ;
#29695=EDGE_CURVE('',#23057,#23059,#19141,.T.) ;
#29696=EDGE_CURVE('',#23059,#23060,#1376,.T.) ;
#29697=EDGE_CURVE('',#23060,#23058,#19142,.T.) ;
#29698=EDGE_CURVE('',#23059,#23061,#5760,.T.) ;
#29699=EDGE_CURVE('',#23061,#23062,#1377,.T.) ;
#29700=EDGE_CURVE('',#23062,#23060,#5761,.T.) ;
#29701=EDGE_CURVE('',#23063,#23061,#19143,.T.) ;
#29702=EDGE_CURVE('',#23063,#23064,#1378,.T.) ;
#29703=EDGE_CURVE('',#23064,#23062,#19144,.T.) ;
#29704=EDGE_CURVE('',#23063,#23065,#5762,.T.) ;
#29705=EDGE_CURVE('',#23065,#23066,#1379,.T.) ;
#29706=EDGE_CURVE('',#23066,#23064,#5763,.T.) ;
#29707=EDGE_CURVE('',#23065,#23067,#19145,.T.) ;
#29708=EDGE_CURVE('',#23067,#23068,#1380,.T.) ;
#29709=EDGE_CURVE('',#23068,#23066,#19146,.T.) ;
#29710=EDGE_CURVE('',#23067,#23069,#5764,.T.) ;
#29711=EDGE_CURVE('',#23069,#23070,#1381,.T.) ;
#29712=EDGE_CURVE('',#23070,#23068,#5765,.T.) ;
#29713=EDGE_CURVE('',#23071,#23069,#19147,.T.) ;
#29714=EDGE_CURVE('',#23071,#23072,#1382,.T.) ;
#29715=EDGE_CURVE('',#23072,#23070,#19148,.T.) ;
#29716=EDGE_CURVE('',#23071,#23073,#5766,.T.) ;
#29717=EDGE_CURVE('',#23073,#23074,#1383,.T.) ;
#29718=EDGE_CURVE('',#23074,#23072,#5767,.T.) ;
#29719=EDGE_CURVE('',#23073,#23075,#19149,.T.) ;
#29720=EDGE_CURVE('',#23075,#23076,#1384,.T.) ;
#29721=EDGE_CURVE('',#23076,#23074,#19150,.T.) ;
#29722=EDGE_CURVE('',#23075,#23077,#5768,.T.) ;
#29723=EDGE_CURVE('',#23077,#23078,#1385,.T.) ;
#29724=EDGE_CURVE('',#23078,#23076,#5769,.T.) ;
#29725=EDGE_CURVE('',#23079,#23077,#19151,.T.) ;
#29726=EDGE_CURVE('',#23079,#23080,#1386,.T.) ;
#29727=EDGE_CURVE('',#23080,#23078,#19152,.T.) ;
#29728=EDGE_CURVE('',#23079,#23081,#5770,.T.) ;
#29729=EDGE_CURVE('',#23081,#23082,#1387,.T.) ;
#29730=EDGE_CURVE('',#23082,#23080,#5771,.T.) ;
#29731=EDGE_CURVE('',#23081,#23083,#19153,.T.) ;
#29732=EDGE_CURVE('',#23083,#23084,#1388,.T.) ;
#29733=EDGE_CURVE('',#23084,#23082,#19154,.T.) ;
#29734=EDGE_CURVE('',#23083,#23085,#5772,.T.) ;
#29735=EDGE_CURVE('',#23085,#23086,#1389,.T.) ;
#29736=EDGE_CURVE('',#23086,#23084,#5773,.T.) ;
#29737=EDGE_CURVE('',#23087,#23085,#19155,.T.) ;
#29738=EDGE_CURVE('',#23087,#23088,#1390,.T.) ;
#29739=EDGE_CURVE('',#23088,#23086,#19156,.T.) ;
#29740=EDGE_CURVE('',#23087,#23089,#5774,.T.) ;
#29741=EDGE_CURVE('',#23089,#23090,#1391,.T.) ;
#29742=EDGE_CURVE('',#23090,#23088,#5775,.T.) ;
#29743=EDGE_CURVE('',#23089,#23091,#19157,.T.) ;
#29744=EDGE_CURVE('',#23091,#23092,#1392,.T.) ;
#29745=EDGE_CURVE('',#23092,#23090,#19158,.T.) ;
#29746=EDGE_CURVE('',#23091,#23093,#5776,.T.) ;
#29747=EDGE_CURVE('',#23093,#23094,#1393,.T.) ;
#29748=EDGE_CURVE('',#23094,#23092,#5777,.T.) ;
#29749=EDGE_CURVE('',#23095,#23093,#19159,.T.) ;
#29750=EDGE_CURVE('',#23095,#23096,#1394,.T.) ;
#29751=EDGE_CURVE('',#23096,#23094,#19160,.T.) ;
#29752=EDGE_CURVE('',#23095,#23097,#5778,.T.) ;
#29753=EDGE_CURVE('',#23097,#23098,#1395,.T.) ;
#29754=EDGE_CURVE('',#23098,#23096,#5779,.T.) ;
#29755=EDGE_CURVE('',#23097,#23099,#19161,.T.) ;
#29756=EDGE_CURVE('',#23099,#23100,#1396,.T.) ;
#29757=EDGE_CURVE('',#23100,#23098,#19162,.T.) ;
#29758=EDGE_CURVE('',#23099,#23101,#5780,.T.) ;
#29759=EDGE_CURVE('',#23101,#23102,#1397,.T.) ;
#29760=EDGE_CURVE('',#23102,#23100,#5781,.T.) ;
#29761=EDGE_CURVE('',#23103,#23101,#19163,.T.) ;
#29762=EDGE_CURVE('',#23103,#23104,#1398,.T.) ;
#29763=EDGE_CURVE('',#23104,#23102,#19164,.T.) ;
#29764=EDGE_CURVE('',#23103,#23105,#5782,.T.) ;
#29765=EDGE_CURVE('',#23105,#23106,#1399,.T.) ;
#29766=EDGE_CURVE('',#23106,#23104,#5783,.T.) ;
#29767=EDGE_CURVE('',#23105,#23107,#19165,.T.) ;
#29768=EDGE_CURVE('',#23107,#23108,#1400,.T.) ;
#29769=EDGE_CURVE('',#23108,#23106,#19166,.T.) ;
#29770=EDGE_CURVE('',#23107,#23109,#5784,.T.) ;
#29771=EDGE_CURVE('',#23109,#23110,#1401,.T.) ;
#29772=EDGE_CURVE('',#23110,#23108,#5785,.T.) ;
#29773=EDGE_CURVE('',#23111,#23109,#19167,.T.) ;
#29774=EDGE_CURVE('',#23111,#23112,#1402,.T.) ;
#29775=EDGE_CURVE('',#23112,#23110,#19168,.T.) ;
#29776=EDGE_CURVE('',#23111,#23113,#5786,.T.) ;
#29777=EDGE_CURVE('',#23113,#23114,#1403,.T.) ;
#29778=EDGE_CURVE('',#23114,#23112,#5787,.T.) ;
#29779=EDGE_CURVE('',#23113,#23115,#19169,.T.) ;
#29780=EDGE_CURVE('',#23115,#23116,#1404,.T.) ;
#29781=EDGE_CURVE('',#23116,#23114,#19170,.T.) ;
#29782=EDGE_CURVE('',#23115,#23117,#5788,.T.) ;
#29783=EDGE_CURVE('',#23117,#23118,#1405,.T.) ;
#29784=EDGE_CURVE('',#23118,#23116,#5789,.T.) ;
#29785=EDGE_CURVE('',#23119,#23117,#19171,.T.) ;
#29786=EDGE_CURVE('',#23119,#23120,#1406,.T.) ;
#29787=EDGE_CURVE('',#23120,#23118,#19172,.T.) ;
#29788=EDGE_CURVE('',#23119,#23121,#5790,.T.) ;
#29789=EDGE_CURVE('',#23121,#23122,#1407,.T.) ;
#29790=EDGE_CURVE('',#23122,#23120,#5791,.T.) ;
#29791=EDGE_CURVE('',#23121,#23123,#19173,.T.) ;
#29792=EDGE_CURVE('',#23123,#23124,#1408,.T.) ;
#29793=EDGE_CURVE('',#23124,#23122,#19174,.T.) ;
#29794=EDGE_CURVE('',#23123,#23125,#5792,.T.) ;
#29795=EDGE_CURVE('',#23125,#23126,#1409,.T.) ;
#29796=EDGE_CURVE('',#23126,#23124,#5793,.T.) ;
#29797=EDGE_CURVE('',#23127,#23125,#19175,.T.) ;
#29798=EDGE_CURVE('',#23127,#23128,#1410,.T.) ;
#29799=EDGE_CURVE('',#23128,#23126,#19176,.T.) ;
#29800=EDGE_CURVE('',#23129,#23128,#5794,.T.) ;
#29801=EDGE_CURVE('',#23127,#23130,#5795,.T.) ;
#29802=EDGE_CURVE('',#23130,#23129,#1411,.T.) ;
#29803=EDGE_CURVE('',#23131,#23129,#19177,.T.) ;
#29804=EDGE_CURVE('',#23130,#23132,#19178,.T.) ;
#29805=EDGE_CURVE('',#23132,#23131,#1412,.T.) ;
#29806=EDGE_CURVE('',#23133,#23131,#5796,.T.) ;
#29807=EDGE_CURVE('',#23132,#23134,#5797,.T.) ;
#29808=EDGE_CURVE('',#23134,#23133,#1413,.T.) ;
#29809=EDGE_CURVE('',#23135,#23133,#19179,.T.) ;
#29810=EDGE_CURVE('',#23136,#23134,#19180,.T.) ;
#29811=EDGE_CURVE('',#23136,#23135,#1414,.T.) ;
#29812=EDGE_CURVE('',#23137,#23135,#5798,.T.) ;
#29813=EDGE_CURVE('',#23136,#23138,#5799,.T.) ;
#29814=EDGE_CURVE('',#23138,#23137,#1415,.T.) ;
#29815=EDGE_CURVE('',#23139,#23137,#19181,.T.) ;
#29816=EDGE_CURVE('',#23138,#23140,#19182,.T.) ;
#29817=EDGE_CURVE('',#23140,#23139,#1416,.T.) ;
#29818=EDGE_CURVE('',#23141,#23139,#5800,.T.) ;
#29819=EDGE_CURVE('',#23140,#23142,#5801,.T.) ;
#29820=EDGE_CURVE('',#23142,#23141,#1417,.T.) ;
#29821=EDGE_CURVE('',#23143,#23141,#19183,.T.) ;
#29822=EDGE_CURVE('',#23144,#23142,#19184,.T.) ;
#29823=EDGE_CURVE('',#23144,#23143,#1418,.T.) ;
#29824=EDGE_CURVE('',#23145,#23143,#5802,.T.) ;
#29825=EDGE_CURVE('',#23144,#23146,#5803,.T.) ;
#29826=EDGE_CURVE('',#23146,#23145,#1419,.T.) ;
#29827=EDGE_CURVE('',#23147,#23145,#19185,.T.) ;
#29828=EDGE_CURVE('',#23146,#23148,#19186,.T.) ;
#29829=EDGE_CURVE('',#23148,#23147,#1420,.T.) ;
#29830=EDGE_CURVE('',#23149,#23147,#5804,.T.) ;
#29831=EDGE_CURVE('',#23148,#23150,#5805,.T.) ;
#29832=EDGE_CURVE('',#23150,#23149,#1421,.T.) ;
#29833=EDGE_CURVE('',#23151,#23149,#19187,.T.) ;
#29834=EDGE_CURVE('',#23152,#23150,#19188,.T.) ;
#29835=EDGE_CURVE('',#23152,#23151,#1422,.T.) ;
#29836=EDGE_CURVE('',#23153,#23151,#5806,.T.) ;
#29837=EDGE_CURVE('',#23152,#23154,#5807,.T.) ;
#29838=EDGE_CURVE('',#23154,#23153,#1423,.T.) ;
#29839=EDGE_CURVE('',#23155,#23153,#19189,.T.) ;
#29840=EDGE_CURVE('',#23154,#23156,#19190,.T.) ;
#29841=EDGE_CURVE('',#23156,#23155,#1424,.T.) ;
#29842=EDGE_CURVE('',#23157,#23155,#5808,.T.) ;
#29843=EDGE_CURVE('',#23156,#23158,#5809,.T.) ;
#29844=EDGE_CURVE('',#23158,#23157,#1425,.T.) ;
#29845=EDGE_CURVE('',#23159,#23157,#19191,.T.) ;
#29846=EDGE_CURVE('',#23160,#23158,#19192,.T.) ;
#29847=EDGE_CURVE('',#23160,#23159,#1426,.T.) ;
#29848=EDGE_CURVE('',#23161,#23159,#5810,.T.) ;
#29849=EDGE_CURVE('',#23160,#23162,#5811,.T.) ;
#29850=EDGE_CURVE('',#23162,#23161,#1427,.T.) ;
#29851=EDGE_CURVE('',#23163,#23161,#19193,.T.) ;
#29852=EDGE_CURVE('',#23162,#23164,#19194,.T.) ;
#29853=EDGE_CURVE('',#23164,#23163,#1428,.T.) ;
#29854=EDGE_CURVE('',#23165,#23163,#5812,.T.) ;
#29855=EDGE_CURVE('',#23164,#23166,#5813,.T.) ;
#29856=EDGE_CURVE('',#23166,#23165,#1429,.T.) ;
#29857=EDGE_CURVE('',#23167,#23165,#19195,.T.) ;
#29858=EDGE_CURVE('',#23168,#23166,#19196,.T.) ;
#29859=EDGE_CURVE('',#23168,#23167,#1430,.T.) ;
#29860=EDGE_CURVE('',#23169,#23167,#5814,.T.) ;
#29861=EDGE_CURVE('',#23168,#23170,#5815,.T.) ;
#29862=EDGE_CURVE('',#23170,#23169,#1431,.T.) ;
#29863=EDGE_CURVE('',#23171,#23169,#19197,.T.) ;
#29864=EDGE_CURVE('',#23170,#23172,#19198,.T.) ;
#29865=EDGE_CURVE('',#23172,#23171,#1432,.T.) ;
#29866=EDGE_CURVE('',#23173,#23171,#5816,.T.) ;
#29867=EDGE_CURVE('',#23172,#23174,#5817,.T.) ;
#29868=EDGE_CURVE('',#23174,#23173,#1433,.T.) ;
#29869=EDGE_CURVE('',#23175,#23173,#19199,.T.) ;
#29870=EDGE_CURVE('',#23176,#23174,#19200,.T.) ;
#29871=EDGE_CURVE('',#23176,#23175,#1434,.T.) ;
#29872=EDGE_CURVE('',#23177,#23175,#5818,.T.) ;
#29873=EDGE_CURVE('',#23176,#23178,#5819,.T.) ;
#29874=EDGE_CURVE('',#23178,#23177,#1435,.T.) ;
#29875=EDGE_CURVE('',#23179,#23177,#19201,.T.) ;
#29876=EDGE_CURVE('',#23178,#23180,#19202,.T.) ;
#29877=EDGE_CURVE('',#23180,#23179,#1436,.T.) ;
#29878=EDGE_CURVE('',#23181,#23179,#5820,.T.) ;
#29879=EDGE_CURVE('',#23180,#23182,#5821,.T.) ;
#29880=EDGE_CURVE('',#23182,#23181,#1437,.T.) ;
#29881=EDGE_CURVE('',#23183,#23181,#19203,.T.) ;
#29882=EDGE_CURVE('',#23184,#23182,#19204,.T.) ;
#29883=EDGE_CURVE('',#23184,#23183,#1438,.T.) ;
#29884=EDGE_CURVE('',#23185,#23183,#5822,.T.) ;
#29885=EDGE_CURVE('',#23184,#23186,#5823,.T.) ;
#29886=EDGE_CURVE('',#23186,#23185,#1439,.T.) ;
#29887=EDGE_CURVE('',#23187,#23185,#19205,.T.) ;
#29888=EDGE_CURVE('',#23186,#23188,#19206,.T.) ;
#29889=EDGE_CURVE('',#23188,#23187,#1440,.T.) ;
#29890=EDGE_CURVE('',#23189,#23187,#5824,.T.) ;
#29891=EDGE_CURVE('',#23188,#23190,#5825,.T.) ;
#29892=EDGE_CURVE('',#23190,#23189,#1441,.T.) ;
#29893=EDGE_CURVE('',#23191,#23189,#19207,.T.) ;
#29894=EDGE_CURVE('',#23192,#23190,#19208,.T.) ;
#29895=EDGE_CURVE('',#23192,#23191,#1442,.T.) ;
#29896=EDGE_CURVE('',#23193,#23191,#5826,.T.) ;
#29897=EDGE_CURVE('',#23192,#23194,#5827,.T.) ;
#29898=EDGE_CURVE('',#23194,#23193,#1443,.T.) ;
#29899=EDGE_CURVE('',#23195,#23193,#19209,.T.) ;
#29900=EDGE_CURVE('',#23194,#23196,#19210,.T.) ;
#29901=EDGE_CURVE('',#23196,#23195,#1444,.T.) ;
#29902=EDGE_CURVE('',#23197,#23195,#5828,.T.) ;
#29903=EDGE_CURVE('',#23196,#23198,#5829,.T.) ;
#29904=EDGE_CURVE('',#23198,#23197,#1445,.T.) ;
#29905=EDGE_CURVE('',#23199,#23197,#19211,.T.) ;
#29906=EDGE_CURVE('',#23200,#23198,#19212,.T.) ;
#29907=EDGE_CURVE('',#23200,#23199,#1446,.T.) ;
#29908=EDGE_CURVE('',#23201,#23199,#5830,.T.) ;
#29909=EDGE_CURVE('',#23200,#23202,#5831,.T.) ;
#29910=EDGE_CURVE('',#23202,#23201,#1447,.T.) ;
#29911=EDGE_CURVE('',#23203,#23201,#19213,.T.) ;
#29912=EDGE_CURVE('',#23202,#23204,#19214,.T.) ;
#29913=EDGE_CURVE('',#23204,#23203,#1448,.T.) ;
#29914=EDGE_CURVE('',#23048,#23203,#5832,.T.) ;
#29915=EDGE_CURVE('',#23204,#23046,#5833,.T.) ;
#29916=EDGE_CURVE('',#23205,#23129,#5834,.T.) ;
#29917=EDGE_CURVE('',#23206,#23205,#5835,.T.) ;
#29918=EDGE_CURVE('',#23128,#23206,#5836,.T.) ;
#29919=EDGE_CURVE('',#23207,#23131,#5837,.T.) ;
#29920=EDGE_CURVE('',#23205,#23207,#19215,.T.) ;
#29921=EDGE_CURVE('',#23208,#23133,#5838,.T.) ;
#29922=EDGE_CURVE('',#23207,#23208,#5839,.T.) ;
#29923=EDGE_CURVE('',#23135,#23209,#5840,.T.) ;
#29924=EDGE_CURVE('',#23208,#23209,#19216,.T.) ;
#29925=EDGE_CURVE('',#23210,#23137,#5841,.T.) ;
#29926=EDGE_CURVE('',#23209,#23210,#5842,.T.) ;
#29927=EDGE_CURVE('',#23211,#23139,#5843,.T.) ;
#29928=EDGE_CURVE('',#23210,#23211,#19217,.T.) ;
#29929=EDGE_CURVE('',#23212,#23141,#5844,.T.) ;
#29930=EDGE_CURVE('',#23211,#23212,#5845,.T.) ;
#29931=EDGE_CURVE('',#23143,#23213,#5846,.T.) ;
#29932=EDGE_CURVE('',#23212,#23213,#19218,.T.) ;
#29933=EDGE_CURVE('',#23214,#23145,#5847,.T.) ;
#29934=EDGE_CURVE('',#23213,#23214,#5848,.T.) ;
#29935=EDGE_CURVE('',#23215,#23147,#5849,.T.) ;
#29936=EDGE_CURVE('',#23214,#23215,#19219,.T.) ;
#29937=EDGE_CURVE('',#23216,#23149,#5850,.T.) ;
#29938=EDGE_CURVE('',#23215,#23216,#5851,.T.) ;
#29939=EDGE_CURVE('',#23151,#23217,#5852,.T.) ;
#29940=EDGE_CURVE('',#23216,#23217,#19220,.T.) ;
#29941=EDGE_CURVE('',#23218,#23153,#5853,.T.) ;
#29942=EDGE_CURVE('',#23217,#23218,#5854,.T.) ;
#29943=EDGE_CURVE('',#23219,#23155,#5855,.T.) ;
#29944=EDGE_CURVE('',#23218,#23219,#19221,.T.) ;
#29945=EDGE_CURVE('',#23220,#23157,#5856,.T.) ;
#29946=EDGE_CURVE('',#23219,#23220,#5857,.T.) ;
#29947=EDGE_CURVE('',#23159,#23221,#5858,.T.) ;
#29948=EDGE_CURVE('',#23220,#23221,#19222,.T.) ;
#29949=EDGE_CURVE('',#23222,#23161,#5859,.T.) ;
#29950=EDGE_CURVE('',#23221,#23222,#5860,.T.) ;
#29951=EDGE_CURVE('',#23223,#23163,#5861,.T.) ;
#29952=EDGE_CURVE('',#23222,#23223,#19223,.T.) ;
#29953=EDGE_CURVE('',#23224,#23165,#5862,.T.) ;
#29954=EDGE_CURVE('',#23223,#23224,#5863,.T.) ;
#29955=EDGE_CURVE('',#23167,#23225,#5864,.T.) ;
#29956=EDGE_CURVE('',#23224,#23225,#19224,.T.) ;
#29957=EDGE_CURVE('',#23226,#23169,#5865,.T.) ;
#29958=EDGE_CURVE('',#23225,#23226,#5866,.T.) ;
#29959=EDGE_CURVE('',#23227,#23171,#5867,.T.) ;
#29960=EDGE_CURVE('',#23226,#23227,#19225,.T.) ;
#29961=EDGE_CURVE('',#23228,#23173,#5868,.T.) ;
#29962=EDGE_CURVE('',#23227,#23228,#5869,.T.) ;
#29963=EDGE_CURVE('',#23175,#23229,#5870,.T.) ;
#29964=EDGE_CURVE('',#23228,#23229,#19226,.T.) ;
#29965=EDGE_CURVE('',#23230,#23177,#5871,.T.) ;
#29966=EDGE_CURVE('',#23229,#23230,#5872,.T.) ;
#29967=EDGE_CURVE('',#23231,#23179,#5873,.T.) ;
#29968=EDGE_CURVE('',#23230,#23231,#19227,.T.) ;
#29969=EDGE_CURVE('',#23232,#23181,#5874,.T.) ;
#29970=EDGE_CURVE('',#23231,#23232,#5875,.T.) ;
#29971=EDGE_CURVE('',#23183,#23233,#5876,.T.) ;
#29972=EDGE_CURVE('',#23232,#23233,#19228,.T.) ;
#29973=EDGE_CURVE('',#23234,#23185,#5877,.T.) ;
#29974=EDGE_CURVE('',#23233,#23234,#5878,.T.) ;
#29975=EDGE_CURVE('',#23235,#23187,#5879,.T.) ;
#29976=EDGE_CURVE('',#23234,#23235,#19229,.T.) ;
#29977=EDGE_CURVE('',#23236,#23189,#5880,.T.) ;
#29978=EDGE_CURVE('',#23235,#23236,#5881,.T.) ;
#29979=EDGE_CURVE('',#23191,#23237,#5882,.T.) ;
#29980=EDGE_CURVE('',#23236,#23237,#19230,.T.) ;
#29981=EDGE_CURVE('',#23238,#23193,#5883,.T.) ;
#29982=EDGE_CURVE('',#23237,#23238,#5884,.T.) ;
#29983=EDGE_CURVE('',#23239,#23195,#5885,.T.) ;
#29984=EDGE_CURVE('',#23238,#23239,#19231,.T.) ;
#29985=EDGE_CURVE('',#23240,#23197,#5886,.T.) ;
#29986=EDGE_CURVE('',#23239,#23240,#5887,.T.) ;
#29987=EDGE_CURVE('',#23199,#23241,#5888,.T.) ;
#29988=EDGE_CURVE('',#23240,#23241,#19232,.T.) ;
#29989=EDGE_CURVE('',#23242,#23201,#5889,.T.) ;
#29990=EDGE_CURVE('',#23241,#23242,#5890,.T.) ;
#29991=EDGE_CURVE('',#23243,#23203,#5891,.T.) ;
#29992=EDGE_CURVE('',#23242,#23243,#19233,.T.) ;
#29993=EDGE_CURVE('',#23244,#23048,#5892,.T.) ;
#29994=EDGE_CURVE('',#23243,#23244,#5893,.T.) ;
#29995=EDGE_CURVE('',#23047,#23245,#5894,.T.) ;
#29996=EDGE_CURVE('',#23244,#23245,#19234,.T.) ;
#29997=EDGE_CURVE('',#23134,#23127,#19235,.T.) ;
#29998=EDGE_CURVE('',#23142,#23136,#19236,.T.) ;
#29999=EDGE_CURVE('',#23125,#23119,#19237,.T.) ;
#30000=EDGE_CURVE('',#23150,#23144,#19238,.T.) ;
#30001=EDGE_CURVE('',#23117,#23111,#19239,.T.) ;
#30002=EDGE_CURVE('',#23158,#23152,#19240,.T.) ;
#30003=EDGE_CURVE('',#23109,#23103,#19241,.T.) ;
#30004=EDGE_CURVE('',#23166,#23160,#19242,.T.) ;
#30005=EDGE_CURVE('',#23101,#23095,#19243,.T.) ;
#30006=EDGE_CURVE('',#23174,#23168,#19244,.T.) ;
#30007=EDGE_CURVE('',#23093,#23087,#19245,.T.) ;
#30008=EDGE_CURVE('',#23182,#23176,#19246,.T.) ;
#30009=EDGE_CURVE('',#23085,#23079,#19247,.T.) ;
#30010=EDGE_CURVE('',#23190,#23184,#19248,.T.) ;
#30011=EDGE_CURVE('',#23077,#23071,#19249,.T.) ;
#30012=EDGE_CURVE('',#23198,#23192,#19250,.T.) ;
#30013=EDGE_CURVE('',#23069,#23063,#19251,.T.) ;
#30014=EDGE_CURVE('',#23046,#23200,#19252,.T.) ;
#30015=EDGE_CURVE('',#23246,#23055,#19253,.T.) ;
#30016=EDGE_CURVE('',#23061,#23246,#19254,.T.) ;
#30017=EDGE_CURVE('',#23042,#23246,#19255,.T.) ;
#30018=EDGE_CURVE('',#23053,#23045,#19256,.T.) ;
#30019=EDGE_CURVE('',#23044,#23247,#19257,.T.) ;
#30020=EDGE_CURVE('',#23247,#23248,#19258,.T.) ;
#30021=EDGE_CURVE('',#23249,#23248,#19259,.T.) ;
#30022=EDGE_CURVE('',#23249,#23250,#19260,.T.) ;
#30023=EDGE_CURVE('',#23251,#23250,#19261,.T.) ;
#30024=EDGE_CURVE('',#23251,#23252,#19262,.T.) ;
#30025=EDGE_CURVE('',#23253,#23252,#19263,.T.) ;
#30026=EDGE_CURVE('',#23253,#23254,#19264,.T.) ;
#30027=EDGE_CURVE('',#23255,#23254,#19265,.T.) ;
#30028=EDGE_CURVE('',#23255,#23256,#19266,.T.) ;
#30029=EDGE_CURVE('',#23257,#23256,#19267,.T.) ;
#30030=EDGE_CURVE('',#23257,#23258,#19268,.T.) ;
#30031=EDGE_CURVE('',#23259,#23258,#19269,.T.) ;
#30032=EDGE_CURVE('',#23259,#23260,#19270,.T.) ;
#30033=EDGE_CURVE('',#23261,#23260,#19271,.T.) ;
#30034=EDGE_CURVE('',#23261,#23262,#19272,.T.) ;
#30035=EDGE_CURVE('',#23263,#23262,#19273,.T.) ;
#30036=EDGE_CURVE('',#23263,#23264,#19274,.T.) ;
#30037=EDGE_CURVE('',#23265,#23264,#19275,.T.) ;
#30038=EDGE_CURVE('',#23265,#23266,#19276,.T.) ;
#30039=EDGE_CURVE('',#23267,#23266,#19277,.T.) ;
#30040=EDGE_CURVE('',#23267,#23268,#19278,.T.) ;
#30041=EDGE_CURVE('',#23269,#23268,#19279,.T.) ;
#30042=EDGE_CURVE('',#23269,#23270,#19280,.T.) ;
#30043=EDGE_CURVE('',#23271,#23270,#19281,.T.) ;
#30044=EDGE_CURVE('',#23271,#23272,#19282,.T.) ;
#30045=EDGE_CURVE('',#23273,#23272,#19283,.T.) ;
#30046=EDGE_CURVE('',#23273,#23274,#19284,.T.) ;
#30047=EDGE_CURVE('',#23275,#23274,#19285,.T.) ;
#30048=EDGE_CURVE('',#23275,#23276,#19286,.T.) ;
#30049=EDGE_CURVE('',#23277,#23276,#19287,.T.) ;
#30050=EDGE_CURVE('',#23277,#23278,#19288,.T.) ;
#30051=EDGE_CURVE('',#23279,#23278,#19289,.T.) ;
#30052=EDGE_CURVE('',#23279,#23280,#19290,.T.) ;
#30053=EDGE_CURVE('',#23281,#23280,#19291,.T.) ;
#30054=EDGE_CURVE('',#23281,#23282,#19292,.T.) ;
#30055=EDGE_CURVE('',#23283,#23282,#19293,.T.) ;
#30056=EDGE_CURVE('',#23283,#23284,#19294,.T.) ;
#30057=EDGE_CURVE('',#23285,#23284,#19295,.T.) ;
#30058=EDGE_CURVE('',#23285,#23286,#19296,.T.) ;
#30059=EDGE_CURVE('',#23287,#23286,#19297,.T.) ;
#30060=EDGE_CURVE('',#23287,#23247,#19298,.T.) ;
#30061=EDGE_CURVE('',#23288,#23285,#5895,.T.) ;
#30062=EDGE_CURVE('',#23289,#23288,#19299,.T.) ;
#30063=EDGE_CURVE('',#23286,#23289,#5896,.T.) ;
#30064=EDGE_CURVE('',#23290,#23283,#5897,.T.) ;
#30065=EDGE_CURVE('',#23291,#23290,#19300,.T.) ;
#30066=EDGE_CURVE('',#23284,#23291,#5898,.T.) ;
#30067=EDGE_CURVE('',#23292,#23281,#5899,.T.) ;
#30068=EDGE_CURVE('',#23293,#23292,#19301,.T.) ;
#30069=EDGE_CURVE('',#23282,#23293,#5900,.T.) ;
#30070=EDGE_CURVE('',#23294,#23279,#5901,.T.) ;
#30071=EDGE_CURVE('',#23295,#23294,#19302,.T.) ;
#30072=EDGE_CURVE('',#23280,#23295,#5902,.T.) ;
#30073=EDGE_CURVE('',#23296,#23277,#5903,.T.) ;
#30074=EDGE_CURVE('',#23297,#23296,#19303,.T.) ;
#30075=EDGE_CURVE('',#23278,#23297,#5904,.T.) ;
#30076=EDGE_CURVE('',#23298,#23275,#5905,.T.) ;
#30077=EDGE_CURVE('',#23299,#23298,#19304,.T.) ;
#30078=EDGE_CURVE('',#23276,#23299,#5906,.T.) ;
#30079=EDGE_CURVE('',#23300,#23273,#5907,.T.) ;
#30080=EDGE_CURVE('',#23301,#23300,#19305,.T.) ;
#30081=EDGE_CURVE('',#23274,#23301,#5908,.T.) ;
#30082=EDGE_CURVE('',#23302,#23271,#5909,.T.) ;
#30083=EDGE_CURVE('',#23303,#23302,#19306,.T.) ;
#30084=EDGE_CURVE('',#23272,#23303,#5910,.T.) ;
#30085=EDGE_CURVE('',#23304,#23269,#5911,.T.) ;
#30086=EDGE_CURVE('',#23305,#23304,#19307,.T.) ;
#30087=EDGE_CURVE('',#23270,#23305,#5912,.T.) ;
#30088=EDGE_CURVE('',#23306,#23267,#5913,.T.) ;
#30089=EDGE_CURVE('',#23307,#23306,#19308,.T.) ;
#30090=EDGE_CURVE('',#23268,#23307,#5914,.T.) ;
#30091=EDGE_CURVE('',#23308,#23265,#5915,.T.) ;
#30092=EDGE_CURVE('',#23309,#23308,#19309,.T.) ;
#30093=EDGE_CURVE('',#23266,#23309,#5916,.T.) ;
#30094=EDGE_CURVE('',#23310,#23263,#5917,.T.) ;
#30095=EDGE_CURVE('',#23311,#23310,#19310,.T.) ;
#30096=EDGE_CURVE('',#23264,#23311,#5918,.T.) ;
#30097=EDGE_CURVE('',#23312,#23261,#5919,.T.) ;
#30098=EDGE_CURVE('',#23313,#23312,#19311,.T.) ;
#30099=EDGE_CURVE('',#23262,#23313,#5920,.T.) ;
#30100=EDGE_CURVE('',#23314,#23259,#5921,.T.) ;
#30101=EDGE_CURVE('',#23315,#23314,#19312,.T.) ;
#30102=EDGE_CURVE('',#23260,#23315,#5922,.T.) ;
#30103=EDGE_CURVE('',#23316,#23257,#5923,.T.) ;
#30104=EDGE_CURVE('',#23317,#23316,#19313,.T.) ;
#30105=EDGE_CURVE('',#23258,#23317,#5924,.T.) ;
#30106=EDGE_CURVE('',#23318,#23255,#5925,.T.) ;
#30107=EDGE_CURVE('',#23319,#23318,#19314,.T.) ;
#30108=EDGE_CURVE('',#23256,#23319,#5926,.T.) ;
#30109=EDGE_CURVE('',#23320,#23253,#5927,.T.) ;
#30110=EDGE_CURVE('',#23321,#23320,#19315,.T.) ;
#30111=EDGE_CURVE('',#23254,#23321,#5928,.T.) ;
#30112=EDGE_CURVE('',#23322,#23251,#5929,.T.) ;
#30113=EDGE_CURVE('',#23323,#23322,#19316,.T.) ;
#30114=EDGE_CURVE('',#23252,#23323,#5930,.T.) ;
#30115=EDGE_CURVE('',#23324,#23249,#5931,.T.) ;
#30116=EDGE_CURVE('',#23325,#23324,#19317,.T.) ;
#30117=EDGE_CURVE('',#23250,#23325,#5932,.T.) ;
#30118=EDGE_CURVE('',#23326,#23287,#5933,.T.) ;
#30119=EDGE_CURVE('',#23327,#23326,#19318,.T.) ;
#30120=EDGE_CURVE('',#23248,#23327,#5934,.T.) ;
#30121=EDGE_CURVE('',#23266,#23328,#1449,.T.) ;
#30122=EDGE_CURVE('',#23328,#23329,#19319,.T.) ;
#30123=EDGE_CURVE('',#23267,#23329,#1450,.T.) ;
#30124=EDGE_CURVE('',#23309,#23330,#1451,.T.) ;
#30125=EDGE_CURVE('',#23330,#23328,#5935,.T.) ;
#30126=EDGE_CURVE('',#23329,#23331,#5936,.T.) ;
#30127=EDGE_CURVE('',#23331,#23306,#1452,.T.) ;
#30128=EDGE_CURVE('',#23265,#23245,#1453,.T.) ;
#30129=EDGE_CURVE('',#23245,#23332,#5937,.T.) ;
#30130=EDGE_CURVE('',#23332,#23308,#1454,.T.) ;
#30131=EDGE_CURVE('',#23264,#23244,#1455,.T.) ;
#30132=EDGE_CURVE('',#23311,#23243,#1456,.T.) ;
#30133=EDGE_CURVE('',#23333,#23334,#5938,.T.) ;
#30134=EDGE_CURVE('',#23334,#23304,#1457,.T.) ;
#30135=EDGE_CURVE('',#23269,#23333,#1458,.T.) ;
#30136=EDGE_CURVE('',#23263,#23241,#1459,.T.) ;
#30137=EDGE_CURVE('',#23242,#23310,#1460,.T.) ;
#30138=EDGE_CURVE('',#23262,#23240,#1461,.T.) ;
#30139=EDGE_CURVE('',#23313,#23239,#1462,.T.) ;
#30140=EDGE_CURVE('',#23335,#23336,#5939,.T.) ;
#30141=EDGE_CURVE('',#23336,#23302,#1463,.T.) ;
#30142=EDGE_CURVE('',#23271,#23335,#1464,.T.) ;
#30143=EDGE_CURVE('',#23261,#23237,#1465,.T.) ;
#30144=EDGE_CURVE('',#23238,#23312,#1466,.T.) ;
#30145=EDGE_CURVE('',#23260,#23236,#1467,.T.) ;
#30146=EDGE_CURVE('',#23315,#23235,#1468,.T.) ;
#30147=EDGE_CURVE('',#23337,#23338,#5940,.T.) ;
#30148=EDGE_CURVE('',#23338,#23300,#1469,.T.) ;
#30149=EDGE_CURVE('',#23273,#23337,#1470,.T.) ;
#30150=EDGE_CURVE('',#23259,#23233,#1471,.T.) ;
#30151=EDGE_CURVE('',#23234,#23314,#1472,.T.) ;
#30152=EDGE_CURVE('',#23258,#23232,#1473,.T.) ;
#30153=EDGE_CURVE('',#23317,#23231,#1474,.T.) ;
#30154=EDGE_CURVE('',#23339,#23340,#5941,.T.) ;
#30155=EDGE_CURVE('',#23340,#23298,#1475,.T.) ;
#30156=EDGE_CURVE('',#23275,#23339,#1476,.T.) ;
#30157=EDGE_CURVE('',#23257,#23229,#1477,.T.) ;
#30158=EDGE_CURVE('',#23230,#23316,#1478,.T.) ;
#30159=EDGE_CURVE('',#23256,#23228,#1479,.T.) ;
#30160=EDGE_CURVE('',#23319,#23227,#1480,.T.) ;
#30161=EDGE_CURVE('',#23341,#23342,#5942,.T.) ;
#30162=EDGE_CURVE('',#23342,#23296,#1481,.T.) ;
#30163=EDGE_CURVE('',#23277,#23341,#1482,.T.) ;
#30164=EDGE_CURVE('',#23255,#23225,#1483,.T.) ;
#30165=EDGE_CURVE('',#23226,#23318,#1484,.T.) ;
#30166=EDGE_CURVE('',#23254,#23224,#1485,.T.) ;
#30167=EDGE_CURVE('',#23321,#23223,#1486,.T.) ;
#30168=EDGE_CURVE('',#23343,#23344,#5943,.T.) ;
#30169=EDGE_CURVE('',#23344,#23294,#1487,.T.) ;
#30170=EDGE_CURVE('',#23279,#23343,#1488,.T.) ;
#30171=EDGE_CURVE('',#23253,#23221,#1489,.T.) ;
#30172=EDGE_CURVE('',#23222,#23320,#1490,.T.) ;
#30173=EDGE_CURVE('',#23252,#23220,#1491,.T.) ;
#30174=EDGE_CURVE('',#23323,#23219,#1492,.T.) ;
#30175=EDGE_CURVE('',#23345,#23346,#5944,.T.) ;
#30176=EDGE_CURVE('',#23346,#23292,#1493,.T.) ;
#30177=EDGE_CURVE('',#23281,#23345,#1494,.T.) ;
#30178=EDGE_CURVE('',#23251,#23217,#1495,.T.) ;
#30179=EDGE_CURVE('',#23218,#23322,#1496,.T.) ;
#30180=EDGE_CURVE('',#23250,#23216,#1497,.T.) ;
#30181=EDGE_CURVE('',#23325,#23215,#1498,.T.) ;
#30182=EDGE_CURVE('',#23347,#23348,#5945,.T.) ;
#30183=EDGE_CURVE('',#23348,#23290,#1499,.T.) ;
#30184=EDGE_CURVE('',#23283,#23347,#1500,.T.) ;
#30185=EDGE_CURVE('',#23249,#23213,#1501,.T.) ;
#30186=EDGE_CURVE('',#23214,#23324,#1502,.T.) ;
#30187=EDGE_CURVE('',#23248,#23212,#1503,.T.) ;
#30188=EDGE_CURVE('',#23327,#23211,#1504,.T.) ;
#30189=EDGE_CURVE('',#23205,#23288,#1505,.T.) ;
#30190=EDGE_CURVE('',#23285,#23206,#1506,.T.) ;
#30191=EDGE_CURVE('',#23287,#23209,#1507,.T.) ;
#30192=EDGE_CURVE('',#23210,#23326,#1508,.T.) ;
#30193=EDGE_CURVE('',#23286,#23208,#1509,.T.) ;
#30194=EDGE_CURVE('',#23289,#23207,#1510,.T.) ;
#30195=EDGE_CURVE('',#23349,#23206,#19320,.T.) ;
#30196=EDGE_CURVE('',#23284,#23349,#1511,.T.) ;
#30197=EDGE_CURVE('',#23350,#23349,#5946,.T.) ;
#30198=EDGE_CURVE('',#23291,#23350,#1512,.T.) ;
#30199=EDGE_CURVE('',#23348,#23350,#19321,.T.) ;
#30200=EDGE_CURVE('',#23351,#23347,#19322,.T.) ;
#30201=EDGE_CURVE('',#23282,#23351,#1513,.T.) ;
#30202=EDGE_CURVE('',#23352,#23351,#5947,.T.) ;
#30203=EDGE_CURVE('',#23293,#23352,#1514,.T.) ;
#30204=EDGE_CURVE('',#23346,#23352,#19323,.T.) ;
#30205=EDGE_CURVE('',#23353,#23345,#19324,.T.) ;
#30206=EDGE_CURVE('',#23280,#23353,#1515,.T.) ;
#30207=EDGE_CURVE('',#23354,#23353,#5948,.T.) ;
#30208=EDGE_CURVE('',#23295,#23354,#1516,.T.) ;
#30209=EDGE_CURVE('',#23344,#23354,#19325,.T.) ;
#30210=EDGE_CURVE('',#23355,#23343,#19326,.T.) ;
#30211=EDGE_CURVE('',#23278,#23355,#1517,.T.) ;
#30212=EDGE_CURVE('',#23356,#23355,#5949,.T.) ;
#30213=EDGE_CURVE('',#23297,#23356,#1518,.T.) ;
#30214=EDGE_CURVE('',#23342,#23356,#19327,.T.) ;
#30215=EDGE_CURVE('',#23357,#23341,#19328,.T.) ;
#30216=EDGE_CURVE('',#23276,#23357,#1519,.T.) ;
#30217=EDGE_CURVE('',#23358,#23357,#5950,.T.) ;
#30218=EDGE_CURVE('',#23299,#23358,#1520,.T.) ;
#30219=EDGE_CURVE('',#23340,#23358,#19329,.T.) ;
#30220=EDGE_CURVE('',#23359,#23339,#19330,.T.) ;
#30221=EDGE_CURVE('',#23274,#23359,#1521,.T.) ;
#30222=EDGE_CURVE('',#23360,#23359,#5951,.T.) ;
#30223=EDGE_CURVE('',#23301,#23360,#1522,.T.) ;
#30224=EDGE_CURVE('',#23338,#23360,#19331,.T.) ;
#30225=EDGE_CURVE('',#23361,#23337,#19332,.T.) ;
#30226=EDGE_CURVE('',#23272,#23361,#1523,.T.) ;
#30227=EDGE_CURVE('',#23362,#23361,#5952,.T.) ;
#30228=EDGE_CURVE('',#23303,#23362,#1524,.T.) ;
#30229=EDGE_CURVE('',#23336,#23362,#19333,.T.) ;
#30230=EDGE_CURVE('',#23363,#23335,#19334,.T.) ;
#30231=EDGE_CURVE('',#23270,#23363,#1525,.T.) ;
#30232=EDGE_CURVE('',#23364,#23363,#5953,.T.) ;
#30233=EDGE_CURVE('',#23305,#23364,#1526,.T.) ;
#30234=EDGE_CURVE('',#23334,#23364,#19335,.T.) ;
#30235=EDGE_CURVE('',#23365,#23333,#19336,.T.) ;
#30236=EDGE_CURVE('',#23268,#23365,#1527,.T.) ;
#30237=EDGE_CURVE('',#23366,#23365,#5954,.T.) ;
#30238=EDGE_CURVE('',#23307,#23366,#1528,.T.) ;
#30239=EDGE_CURVE('',#23331,#23366,#19337,.T.) ;
#30240=EDGE_CURVE('',#23332,#23330,#19338,.T.) ;
#30241=EDGE_CURVE('',#23056,#23329,#5955,.T.) ;
#30242=EDGE_CURVE('',#23328,#23054,#5956,.T.) ;
#30243=EDGE_CURVE('',#23330,#23052,#5957,.T.) ;
#30244=EDGE_CURVE('',#23332,#23050,#5958,.T.) ;
#30245=EDGE_CURVE('',#23349,#23126,#5959,.T.) ;
#30246=EDGE_CURVE('',#23350,#23124,#5960,.T.) ;
#30247=EDGE_CURVE('',#23348,#23122,#5961,.T.) ;
#30248=EDGE_CURVE('',#23120,#23347,#5962,.T.) ;
#30249=EDGE_CURVE('',#23351,#23118,#5963,.T.) ;
#30250=EDGE_CURVE('',#23352,#23116,#5964,.T.) ;
#30251=EDGE_CURVE('',#23346,#23114,#5965,.T.) ;
#30252=EDGE_CURVE('',#23112,#23345,#5966,.T.) ;
#30253=EDGE_CURVE('',#23353,#23110,#5967,.T.) ;
#30254=EDGE_CURVE('',#23354,#23108,#5968,.T.) ;
#30255=EDGE_CURVE('',#23344,#23106,#5969,.T.) ;
#30256=EDGE_CURVE('',#23104,#23343,#5970,.T.) ;
#30257=EDGE_CURVE('',#23355,#23102,#5971,.T.) ;
#30258=EDGE_CURVE('',#23356,#23100,#5972,.T.) ;
#30259=EDGE_CURVE('',#23342,#23098,#5973,.T.) ;
#30260=EDGE_CURVE('',#23096,#23341,#5974,.T.) ;
#30261=EDGE_CURVE('',#23357,#23094,#5975,.T.) ;
#30262=EDGE_CURVE('',#23358,#23092,#5976,.T.) ;
#30263=EDGE_CURVE('',#23340,#23090,#5977,.T.) ;
#30264=EDGE_CURVE('',#23088,#23339,#5978,.T.) ;
#30265=EDGE_CURVE('',#23359,#23086,#5979,.T.) ;
#30266=EDGE_CURVE('',#23360,#23084,#5980,.T.) ;
#30267=EDGE_CURVE('',#23338,#23082,#5981,.T.) ;
#30268=EDGE_CURVE('',#23080,#23337,#5982,.T.) ;
#30269=EDGE_CURVE('',#23361,#23078,#5983,.T.) ;
#30270=EDGE_CURVE('',#23362,#23076,#5984,.T.) ;
#30271=EDGE_CURVE('',#23336,#23074,#5985,.T.) ;
#30272=EDGE_CURVE('',#23072,#23335,#5986,.T.) ;
#30273=EDGE_CURVE('',#23363,#23070,#5987,.T.) ;
#30274=EDGE_CURVE('',#23364,#23068,#5988,.T.) ;
#30275=EDGE_CURVE('',#23334,#23066,#5989,.T.) ;
#30276=EDGE_CURVE('',#23064,#23333,#5990,.T.) ;
#30277=EDGE_CURVE('',#23365,#23062,#5991,.T.) ;
#30278=EDGE_CURVE('',#23366,#23060,#5992,.T.) ;
#30279=EDGE_CURVE('',#23331,#23058,#5993,.T.) ;
#30280=EDGE_CURVE('',#23039,#23040,#5994,.T.) ;
#42764=ORIENTED_EDGE('',*,*,#29660,.F.) ;
#42765=ORIENTED_EDGE('',*,*,#29661,.T.) ;
#42766=ORIENTED_EDGE('',*,*,#29662,.T.) ;
#42767=ORIENTED_EDGE('',*,*,#29661,.F.) ;
#42768=ORIENTED_EDGE('',*,*,#29663,.F.) ;
#42769=ORIENTED_EDGE('',*,*,#29662,.F.) ;
#42770=ORIENTED_EDGE('',*,*,#29664,.T.) ;
#42771=ORIENTED_EDGE('',*,*,#29665,.T.) ;
#42772=ORIENTED_EDGE('',*,*,#29666,.F.) ;
#42773=ORIENTED_EDGE('',*,*,#29665,.F.) ;
#42774=ORIENTED_EDGE('',*,*,#29667,.F.) ;
#42775=ORIENTED_EDGE('',*,*,#29664,.F.) ;
#42776=ORIENTED_EDGE('',*,*,#29666,.T.) ;
#42777=ORIENTED_EDGE('',*,*,#29668,.T.) ;
#42778=ORIENTED_EDGE('',*,*,#29660,.T.) ;
#42779=ORIENTED_EDGE('',*,*,#29669,.T.) ;
#42780=ORIENTED_EDGE('',*,*,#29670,.T.) ;
#42781=ORIENTED_EDGE('',*,*,#29671,.T.) ;
#42782=ORIENTED_EDGE('',*,*,#29672,.T.) ;
#42783=ORIENTED_EDGE('',*,*,#29670,.F.) ;
#42784=ORIENTED_EDGE('',*,*,#29663,.T.) ;
#42785=ORIENTED_EDGE('',*,*,#29673,.T.) ;
#42786=ORIENTED_EDGE('',*,*,#29674,.T.) ;
#42787=ORIENTED_EDGE('',*,*,#29675,.T.) ;
#42788=ORIENTED_EDGE('',*,*,#29673,.F.) ;
#42789=ORIENTED_EDGE('',*,*,#29667,.T.) ;
#42790=ORIENTED_EDGE('',*,*,#29676,.F.) ;
#42791=ORIENTED_EDGE('',*,*,#29677,.T.) ;
#42792=ORIENTED_EDGE('',*,*,#29678,.T.) ;
#42793=ORIENTED_EDGE('',*,*,#29679,.F.) ;
#42794=ORIENTED_EDGE('',*,*,#29680,.T.) ;
#42795=ORIENTED_EDGE('',*,*,#29681,.T.) ;
#42796=ORIENTED_EDGE('',*,*,#29682,.T.) ;
#42797=ORIENTED_EDGE('',*,*,#29677,.F.) ;
#42798=ORIENTED_EDGE('',*,*,#29683,.T.) ;
#42799=ORIENTED_EDGE('',*,*,#29684,.T.) ;
#42800=ORIENTED_EDGE('',*,*,#29685,.T.) ;
#42801=ORIENTED_EDGE('',*,*,#29681,.F.) ;
#42802=ORIENTED_EDGE('',*,*,#29686,.T.) ;
#42803=ORIENTED_EDGE('',*,*,#29687,.T.) ;
#42804=ORIENTED_EDGE('',*,*,#29688,.T.) ;
#42805=ORIENTED_EDGE('',*,*,#29684,.F.) ;
#42806=ORIENTED_EDGE('',*,*,#29689,.F.) ;
#42807=ORIENTED_EDGE('',*,*,#29690,.T.) ;
#42808=ORIENTED_EDGE('',*,*,#29691,.T.) ;
#42809=ORIENTED_EDGE('',*,*,#29687,.F.) ;
#42810=ORIENTED_EDGE('',*,*,#29692,.T.) ;
#42811=ORIENTED_EDGE('',*,*,#29693,.T.) ;
#42812=ORIENTED_EDGE('',*,*,#29694,.T.) ;
#42813=ORIENTED_EDGE('',*,*,#29690,.F.) ;
#42814=ORIENTED_EDGE('',*,*,#29695,.T.) ;
#42815=ORIENTED_EDGE('',*,*,#29696,.T.) ;
#42816=ORIENTED_EDGE('',*,*,#29697,.T.) ;
#42817=ORIENTED_EDGE('',*,*,#29693,.F.) ;
#42818=ORIENTED_EDGE('',*,*,#29698,.T.) ;
#42819=ORIENTED_EDGE('',*,*,#29699,.T.) ;
#42820=ORIENTED_EDGE('',*,*,#29700,.T.) ;
#42821=ORIENTED_EDGE('',*,*,#29696,.F.) ;
#42822=ORIENTED_EDGE('',*,*,#29701,.F.) ;
#42823=ORIENTED_EDGE('',*,*,#29702,.T.) ;
#42824=ORIENTED_EDGE('',*,*,#29703,.T.) ;
#42825=ORIENTED_EDGE('',*,*,#29699,.F.) ;
#42826=ORIENTED_EDGE('',*,*,#29704,.T.) ;
#42827=ORIENTED_EDGE('',*,*,#29705,.T.) ;
#42828=ORIENTED_EDGE('',*,*,#29706,.T.) ;
#42829=ORIENTED_EDGE('',*,*,#29702,.F.) ;
#42830=ORIENTED_EDGE('',*,*,#29707,.T.) ;
#42831=ORIENTED_EDGE('',*,*,#29708,.T.) ;
#42832=ORIENTED_EDGE('',*,*,#29709,.T.) ;
#42833=ORIENTED_EDGE('',*,*,#29705,.F.) ;
#42834=ORIENTED_EDGE('',*,*,#29710,.T.) ;
#42835=ORIENTED_EDGE('',*,*,#29711,.T.) ;
#42836=ORIENTED_EDGE('',*,*,#29712,.T.) ;
#42837=ORIENTED_EDGE('',*,*,#29708,.F.) ;
#42838=ORIENTED_EDGE('',*,*,#29713,.F.) ;
#42839=ORIENTED_EDGE('',*,*,#29714,.T.) ;
#42840=ORIENTED_EDGE('',*,*,#29715,.T.) ;
#42841=ORIENTED_EDGE('',*,*,#29711,.F.) ;
#42842=ORIENTED_EDGE('',*,*,#29716,.T.) ;
#42843=ORIENTED_EDGE('',*,*,#29717,.T.) ;
#42844=ORIENTED_EDGE('',*,*,#29718,.T.) ;
#42845=ORIENTED_EDGE('',*,*,#29714,.F.) ;
#42846=ORIENTED_EDGE('',*,*,#29719,.T.) ;
#42847=ORIENTED_EDGE('',*,*,#29720,.T.) ;
#42848=ORIENTED_EDGE('',*,*,#29721,.T.) ;
#42849=ORIENTED_EDGE('',*,*,#29717,.F.) ;
#42850=ORIENTED_EDGE('',*,*,#29722,.T.) ;
#42851=ORIENTED_EDGE('',*,*,#29723,.T.) ;
#42852=ORIENTED_EDGE('',*,*,#29724,.T.) ;
#42853=ORIENTED_EDGE('',*,*,#29720,.F.) ;
#42854=ORIENTED_EDGE('',*,*,#29725,.F.) ;
#42855=ORIENTED_EDGE('',*,*,#29726,.T.) ;
#42856=ORIENTED_EDGE('',*,*,#29727,.T.) ;
#42857=ORIENTED_EDGE('',*,*,#29723,.F.) ;
#42858=ORIENTED_EDGE('',*,*,#29728,.T.) ;
#42859=ORIENTED_EDGE('',*,*,#29729,.T.) ;
#42860=ORIENTED_EDGE('',*,*,#29730,.T.) ;
#42861=ORIENTED_EDGE('',*,*,#29726,.F.) ;
#42862=ORIENTED_EDGE('',*,*,#29731,.T.) ;
#42863=ORIENTED_EDGE('',*,*,#29732,.T.) ;
#42864=ORIENTED_EDGE('',*,*,#29733,.T.) ;
#42865=ORIENTED_EDGE('',*,*,#29729,.F.) ;
#42866=ORIENTED_EDGE('',*,*,#29734,.T.) ;
#42867=ORIENTED_EDGE('',*,*,#29735,.T.) ;
#42868=ORIENTED_EDGE('',*,*,#29736,.T.) ;
#42869=ORIENTED_EDGE('',*,*,#29732,.F.) ;
#42870=ORIENTED_EDGE('',*,*,#29737,.F.) ;
#42871=ORIENTED_EDGE('',*,*,#29738,.T.) ;
#42872=ORIENTED_EDGE('',*,*,#29739,.T.) ;
#42873=ORIENTED_EDGE('',*,*,#29735,.F.) ;
#42874=ORIENTED_EDGE('',*,*,#29740,.T.) ;
#42875=ORIENTED_EDGE('',*,*,#29741,.T.) ;
#42876=ORIENTED_EDGE('',*,*,#29742,.T.) ;
#42877=ORIENTED_EDGE('',*,*,#29738,.F.) ;
#42878=ORIENTED_EDGE('',*,*,#29743,.T.) ;
#42879=ORIENTED_EDGE('',*,*,#29744,.T.) ;
#42880=ORIENTED_EDGE('',*,*,#29745,.T.) ;
#42881=ORIENTED_EDGE('',*,*,#29741,.F.) ;
#42882=ORIENTED_EDGE('',*,*,#29746,.T.) ;
#42883=ORIENTED_EDGE('',*,*,#29747,.T.) ;
#42884=ORIENTED_EDGE('',*,*,#29748,.T.) ;
#42885=ORIENTED_EDGE('',*,*,#29744,.F.) ;
#42886=ORIENTED_EDGE('',*,*,#29749,.F.) ;
#42887=ORIENTED_EDGE('',*,*,#29750,.T.) ;
#42888=ORIENTED_EDGE('',*,*,#29751,.T.) ;
#42889=ORIENTED_EDGE('',*,*,#29747,.F.) ;
#42890=ORIENTED_EDGE('',*,*,#29752,.T.) ;
#42891=ORIENTED_EDGE('',*,*,#29753,.T.) ;
#42892=ORIENTED_EDGE('',*,*,#29754,.T.) ;
#42893=ORIENTED_EDGE('',*,*,#29750,.F.) ;
#42894=ORIENTED_EDGE('',*,*,#29755,.T.) ;
#42895=ORIENTED_EDGE('',*,*,#29756,.T.) ;
#42896=ORIENTED_EDGE('',*,*,#29757,.T.) ;
#42897=ORIENTED_EDGE('',*,*,#29753,.F.) ;
#42898=ORIENTED_EDGE('',*,*,#29758,.T.) ;
#42899=ORIENTED_EDGE('',*,*,#29759,.T.) ;
#42900=ORIENTED_EDGE('',*,*,#29760,.T.) ;
#42901=ORIENTED_EDGE('',*,*,#29756,.F.) ;
#42902=ORIENTED_EDGE('',*,*,#29761,.F.) ;
#42903=ORIENTED_EDGE('',*,*,#29762,.T.) ;
#42904=ORIENTED_EDGE('',*,*,#29763,.T.) ;
#42905=ORIENTED_EDGE('',*,*,#29759,.F.) ;
#42906=ORIENTED_EDGE('',*,*,#29764,.T.) ;
#42907=ORIENTED_EDGE('',*,*,#29765,.T.) ;
#42908=ORIENTED_EDGE('',*,*,#29766,.T.) ;
#42909=ORIENTED_EDGE('',*,*,#29762,.F.) ;
#42910=ORIENTED_EDGE('',*,*,#29767,.T.) ;
#42911=ORIENTED_EDGE('',*,*,#29768,.T.) ;
#42912=ORIENTED_EDGE('',*,*,#29769,.T.) ;
#42913=ORIENTED_EDGE('',*,*,#29765,.F.) ;
#42914=ORIENTED_EDGE('',*,*,#29770,.T.) ;
#42915=ORIENTED_EDGE('',*,*,#29771,.T.) ;
#42916=ORIENTED_EDGE('',*,*,#29772,.T.) ;
#42917=ORIENTED_EDGE('',*,*,#29768,.F.) ;
#42918=ORIENTED_EDGE('',*,*,#29773,.F.) ;
#42919=ORIENTED_EDGE('',*,*,#29774,.T.) ;
#42920=ORIENTED_EDGE('',*,*,#29775,.T.) ;
#42921=ORIENTED_EDGE('',*,*,#29771,.F.) ;
#42922=ORIENTED_EDGE('',*,*,#29776,.T.) ;
#42923=ORIENTED_EDGE('',*,*,#29777,.T.) ;
#42924=ORIENTED_EDGE('',*,*,#29778,.T.) ;
#42925=ORIENTED_EDGE('',*,*,#29774,.F.) ;
#42926=ORIENTED_EDGE('',*,*,#29779,.T.) ;
#42927=ORIENTED_EDGE('',*,*,#29780,.T.) ;
#42928=ORIENTED_EDGE('',*,*,#29781,.T.) ;
#42929=ORIENTED_EDGE('',*,*,#29777,.F.) ;
#42930=ORIENTED_EDGE('',*,*,#29782,.T.) ;
#42931=ORIENTED_EDGE('',*,*,#29783,.T.) ;
#42932=ORIENTED_EDGE('',*,*,#29784,.T.) ;
#42933=ORIENTED_EDGE('',*,*,#29780,.F.) ;
#42934=ORIENTED_EDGE('',*,*,#29785,.F.) ;
#42935=ORIENTED_EDGE('',*,*,#29786,.T.) ;
#42936=ORIENTED_EDGE('',*,*,#29787,.T.) ;
#42937=ORIENTED_EDGE('',*,*,#29783,.F.) ;
#42938=ORIENTED_EDGE('',*,*,#29788,.T.) ;
#42939=ORIENTED_EDGE('',*,*,#29789,.T.) ;
#42940=ORIENTED_EDGE('',*,*,#29790,.T.) ;
#42941=ORIENTED_EDGE('',*,*,#29786,.F.) ;
#42942=ORIENTED_EDGE('',*,*,#29791,.T.) ;
#42943=ORIENTED_EDGE('',*,*,#29792,.T.) ;
#42944=ORIENTED_EDGE('',*,*,#29793,.T.) ;
#42945=ORIENTED_EDGE('',*,*,#29789,.F.) ;
#42946=ORIENTED_EDGE('',*,*,#29794,.T.) ;
#42947=ORIENTED_EDGE('',*,*,#29795,.T.) ;
#42948=ORIENTED_EDGE('',*,*,#29796,.T.) ;
#42949=ORIENTED_EDGE('',*,*,#29792,.F.) ;
#42950=ORIENTED_EDGE('',*,*,#29797,.F.) ;
#42951=ORIENTED_EDGE('',*,*,#29798,.T.) ;
#42952=ORIENTED_EDGE('',*,*,#29799,.T.) ;
#42953=ORIENTED_EDGE('',*,*,#29795,.F.) ;
#42954=ORIENTED_EDGE('',*,*,#29800,.T.) ;
#42955=ORIENTED_EDGE('',*,*,#29798,.F.) ;
#42956=ORIENTED_EDGE('',*,*,#29801,.T.) ;
#42957=ORIENTED_EDGE('',*,*,#29802,.T.) ;
#42958=ORIENTED_EDGE('',*,*,#29803,.T.) ;
#42959=ORIENTED_EDGE('',*,*,#29802,.F.) ;
#42960=ORIENTED_EDGE('',*,*,#29804,.T.) ;
#42961=ORIENTED_EDGE('',*,*,#29805,.T.) ;
#42962=ORIENTED_EDGE('',*,*,#29806,.T.) ;
#42963=ORIENTED_EDGE('',*,*,#29805,.F.) ;
#42964=ORIENTED_EDGE('',*,*,#29807,.T.) ;
#42965=ORIENTED_EDGE('',*,*,#29808,.T.) ;
#42966=ORIENTED_EDGE('',*,*,#29809,.T.) ;
#42967=ORIENTED_EDGE('',*,*,#29808,.F.) ;
#42968=ORIENTED_EDGE('',*,*,#29810,.F.) ;
#42969=ORIENTED_EDGE('',*,*,#29811,.T.) ;
#42970=ORIENTED_EDGE('',*,*,#29812,.T.) ;
#42971=ORIENTED_EDGE('',*,*,#29811,.F.) ;
#42972=ORIENTED_EDGE('',*,*,#29813,.T.) ;
#42973=ORIENTED_EDGE('',*,*,#29814,.T.) ;
#42974=ORIENTED_EDGE('',*,*,#29815,.T.) ;
#42975=ORIENTED_EDGE('',*,*,#29814,.F.) ;
#42976=ORIENTED_EDGE('',*,*,#29816,.T.) ;
#42977=ORIENTED_EDGE('',*,*,#29817,.T.) ;
#42978=ORIENTED_EDGE('',*,*,#29818,.T.) ;
#42979=ORIENTED_EDGE('',*,*,#29817,.F.) ;
#42980=ORIENTED_EDGE('',*,*,#29819,.T.) ;
#42981=ORIENTED_EDGE('',*,*,#29820,.T.) ;
#42982=ORIENTED_EDGE('',*,*,#29821,.T.) ;
#42983=ORIENTED_EDGE('',*,*,#29820,.F.) ;
#42984=ORIENTED_EDGE('',*,*,#29822,.F.) ;
#42985=ORIENTED_EDGE('',*,*,#29823,.T.) ;
#42986=ORIENTED_EDGE('',*,*,#29824,.T.) ;
#42987=ORIENTED_EDGE('',*,*,#29823,.F.) ;
#42988=ORIENTED_EDGE('',*,*,#29825,.T.) ;
#42989=ORIENTED_EDGE('',*,*,#29826,.T.) ;
#42990=ORIENTED_EDGE('',*,*,#29827,.T.) ;
#42991=ORIENTED_EDGE('',*,*,#29826,.F.) ;
#42992=ORIENTED_EDGE('',*,*,#29828,.T.) ;
#42993=ORIENTED_EDGE('',*,*,#29829,.T.) ;
#42994=ORIENTED_EDGE('',*,*,#29830,.T.) ;
#42995=ORIENTED_EDGE('',*,*,#29829,.F.) ;
#42996=ORIENTED_EDGE('',*,*,#29831,.T.) ;
#42997=ORIENTED_EDGE('',*,*,#29832,.T.) ;
#42998=ORIENTED_EDGE('',*,*,#29833,.T.) ;
#42999=ORIENTED_EDGE('',*,*,#29832,.F.) ;
#43000=ORIENTED_EDGE('',*,*,#29834,.F.) ;
#43001=ORIENTED_EDGE('',*,*,#29835,.T.) ;
#43002=ORIENTED_EDGE('',*,*,#29836,.T.) ;
#43003=ORIENTED_EDGE('',*,*,#29835,.F.) ;
#43004=ORIENTED_EDGE('',*,*,#29837,.T.) ;
#43005=ORIENTED_EDGE('',*,*,#29838,.T.) ;
#43006=ORIENTED_EDGE('',*,*,#29839,.T.) ;
#43007=ORIENTED_EDGE('',*,*,#29838,.F.) ;
#43008=ORIENTED_EDGE('',*,*,#29840,.T.) ;
#43009=ORIENTED_EDGE('',*,*,#29841,.T.) ;
#43010=ORIENTED_EDGE('',*,*,#29842,.T.) ;
#43011=ORIENTED_EDGE('',*,*,#29841,.F.) ;
#43012=ORIENTED_EDGE('',*,*,#29843,.T.) ;
#43013=ORIENTED_EDGE('',*,*,#29844,.T.) ;
#43014=ORIENTED_EDGE('',*,*,#29845,.T.) ;
#43015=ORIENTED_EDGE('',*,*,#29844,.F.) ;
#43016=ORIENTED_EDGE('',*,*,#29846,.F.) ;
#43017=ORIENTED_EDGE('',*,*,#29847,.T.) ;
#43018=ORIENTED_EDGE('',*,*,#29848,.T.) ;
#43019=ORIENTED_EDGE('',*,*,#29847,.F.) ;
#43020=ORIENTED_EDGE('',*,*,#29849,.T.) ;
#43021=ORIENTED_EDGE('',*,*,#29850,.T.) ;
#43022=ORIENTED_EDGE('',*,*,#29851,.T.) ;
#43023=ORIENTED_EDGE('',*,*,#29850,.F.) ;
#43024=ORIENTED_EDGE('',*,*,#29852,.T.) ;
#43025=ORIENTED_EDGE('',*,*,#29853,.T.) ;
#43026=ORIENTED_EDGE('',*,*,#29854,.T.) ;
#43027=ORIENTED_EDGE('',*,*,#29853,.F.) ;
#43028=ORIENTED_EDGE('',*,*,#29855,.T.) ;
#43029=ORIENTED_EDGE('',*,*,#29856,.T.) ;
#43030=ORIENTED_EDGE('',*,*,#29857,.T.) ;
#43031=ORIENTED_EDGE('',*,*,#29856,.F.) ;
#43032=ORIENTED_EDGE('',*,*,#29858,.F.) ;
#43033=ORIENTED_EDGE('',*,*,#29859,.T.) ;
#43034=ORIENTED_EDGE('',*,*,#29860,.T.) ;
#43035=ORIENTED_EDGE('',*,*,#29859,.F.) ;
#43036=ORIENTED_EDGE('',*,*,#29861,.T.) ;
#43037=ORIENTED_EDGE('',*,*,#29862,.T.) ;
#43038=ORIENTED_EDGE('',*,*,#29863,.T.) ;
#43039=ORIENTED_EDGE('',*,*,#29862,.F.) ;
#43040=ORIENTED_EDGE('',*,*,#29864,.T.) ;
#43041=ORIENTED_EDGE('',*,*,#29865,.T.) ;
#43042=ORIENTED_EDGE('',*,*,#29866,.T.) ;
#43043=ORIENTED_EDGE('',*,*,#29865,.F.) ;
#43044=ORIENTED_EDGE('',*,*,#29867,.T.) ;
#43045=ORIENTED_EDGE('',*,*,#29868,.T.) ;
#43046=ORIENTED_EDGE('',*,*,#29869,.T.) ;
#43047=ORIENTED_EDGE('',*,*,#29868,.F.) ;
#43048=ORIENTED_EDGE('',*,*,#29870,.F.) ;
#43049=ORIENTED_EDGE('',*,*,#29871,.T.) ;
#43050=ORIENTED_EDGE('',*,*,#29872,.T.) ;
#43051=ORIENTED_EDGE('',*,*,#29871,.F.) ;
#43052=ORIENTED_EDGE('',*,*,#29873,.T.) ;
#43053=ORIENTED_EDGE('',*,*,#29874,.T.) ;
#43054=ORIENTED_EDGE('',*,*,#29875,.T.) ;
#43055=ORIENTED_EDGE('',*,*,#29874,.F.) ;
#43056=ORIENTED_EDGE('',*,*,#29876,.T.) ;
#43057=ORIENTED_EDGE('',*,*,#29877,.T.) ;
#43058=ORIENTED_EDGE('',*,*,#29878,.T.) ;
#43059=ORIENTED_EDGE('',*,*,#29877,.F.) ;
#43060=ORIENTED_EDGE('',*,*,#29879,.T.) ;
#43061=ORIENTED_EDGE('',*,*,#29880,.T.) ;
#43062=ORIENTED_EDGE('',*,*,#29881,.T.) ;
#43063=ORIENTED_EDGE('',*,*,#29880,.F.) ;
#43064=ORIENTED_EDGE('',*,*,#29882,.F.) ;
#43065=ORIENTED_EDGE('',*,*,#29883,.T.) ;
#43066=ORIENTED_EDGE('',*,*,#29884,.T.) ;
#43067=ORIENTED_EDGE('',*,*,#29883,.F.) ;
#43068=ORIENTED_EDGE('',*,*,#29885,.T.) ;
#43069=ORIENTED_EDGE('',*,*,#29886,.T.) ;
#43070=ORIENTED_EDGE('',*,*,#29887,.T.) ;
#43071=ORIENTED_EDGE('',*,*,#29886,.F.) ;
#43072=ORIENTED_EDGE('',*,*,#29888,.T.) ;
#43073=ORIENTED_EDGE('',*,*,#29889,.T.) ;
#43074=ORIENTED_EDGE('',*,*,#29890,.T.) ;
#43075=ORIENTED_EDGE('',*,*,#29889,.F.) ;
#43076=ORIENTED_EDGE('',*,*,#29891,.T.) ;
#43077=ORIENTED_EDGE('',*,*,#29892,.T.) ;
#43078=ORIENTED_EDGE('',*,*,#29893,.T.) ;
#43079=ORIENTED_EDGE('',*,*,#29892,.F.) ;
#43080=ORIENTED_EDGE('',*,*,#29894,.F.) ;
#43081=ORIENTED_EDGE('',*,*,#29895,.T.) ;
#43082=ORIENTED_EDGE('',*,*,#29896,.T.) ;
#43083=ORIENTED_EDGE('',*,*,#29895,.F.) ;
#43084=ORIENTED_EDGE('',*,*,#29897,.T.) ;
#43085=ORIENTED_EDGE('',*,*,#29898,.T.) ;
#43086=ORIENTED_EDGE('',*,*,#29899,.T.) ;
#43087=ORIENTED_EDGE('',*,*,#29898,.F.) ;
#43088=ORIENTED_EDGE('',*,*,#29900,.T.) ;
#43089=ORIENTED_EDGE('',*,*,#29901,.T.) ;
#43090=ORIENTED_EDGE('',*,*,#29902,.T.) ;
#43091=ORIENTED_EDGE('',*,*,#29901,.F.) ;
#43092=ORIENTED_EDGE('',*,*,#29903,.T.) ;
#43093=ORIENTED_EDGE('',*,*,#29904,.T.) ;
#43094=ORIENTED_EDGE('',*,*,#29905,.T.) ;
#43095=ORIENTED_EDGE('',*,*,#29904,.F.) ;
#43096=ORIENTED_EDGE('',*,*,#29906,.F.) ;
#43097=ORIENTED_EDGE('',*,*,#29907,.T.) ;
#43098=ORIENTED_EDGE('',*,*,#29908,.T.) ;
#43099=ORIENTED_EDGE('',*,*,#29907,.F.) ;
#43100=ORIENTED_EDGE('',*,*,#29909,.T.) ;
#43101=ORIENTED_EDGE('',*,*,#29910,.T.) ;
#43102=ORIENTED_EDGE('',*,*,#29911,.T.) ;
#43103=ORIENTED_EDGE('',*,*,#29910,.F.) ;
#43104=ORIENTED_EDGE('',*,*,#29912,.T.) ;
#43105=ORIENTED_EDGE('',*,*,#29913,.T.) ;
#43106=ORIENTED_EDGE('',*,*,#29914,.T.) ;
#43107=ORIENTED_EDGE('',*,*,#29913,.F.) ;
#43108=ORIENTED_EDGE('',*,*,#29915,.T.) ;
#43109=ORIENTED_EDGE('',*,*,#29679,.T.) ;
#43110=ORIENTED_EDGE('',*,*,#29800,.F.) ;
#43111=ORIENTED_EDGE('',*,*,#29916,.F.) ;
#43112=ORIENTED_EDGE('',*,*,#29917,.F.) ;
#43113=ORIENTED_EDGE('',*,*,#29918,.F.) ;
#43114=ORIENTED_EDGE('',*,*,#29803,.F.) ;
#43115=ORIENTED_EDGE('',*,*,#29919,.F.) ;
#43116=ORIENTED_EDGE('',*,*,#29920,.F.) ;
#43117=ORIENTED_EDGE('',*,*,#29916,.T.) ;
#43118=ORIENTED_EDGE('',*,*,#29806,.F.) ;
#43119=ORIENTED_EDGE('',*,*,#29921,.F.) ;
#43120=ORIENTED_EDGE('',*,*,#29922,.F.) ;
#43121=ORIENTED_EDGE('',*,*,#29919,.T.) ;
#43122=ORIENTED_EDGE('',*,*,#29809,.F.) ;
#43123=ORIENTED_EDGE('',*,*,#29923,.T.) ;
#43124=ORIENTED_EDGE('',*,*,#29924,.F.) ;
#43125=ORIENTED_EDGE('',*,*,#29921,.T.) ;
#43126=ORIENTED_EDGE('',*,*,#29812,.F.) ;
#43127=ORIENTED_EDGE('',*,*,#29925,.F.) ;
#43128=ORIENTED_EDGE('',*,*,#29926,.F.) ;
#43129=ORIENTED_EDGE('',*,*,#29923,.F.) ;
#43130=ORIENTED_EDGE('',*,*,#29815,.F.) ;
#43131=ORIENTED_EDGE('',*,*,#29927,.F.) ;
#43132=ORIENTED_EDGE('',*,*,#29928,.F.) ;
#43133=ORIENTED_EDGE('',*,*,#29925,.T.) ;
#43134=ORIENTED_EDGE('',*,*,#29818,.F.) ;
#43135=ORIENTED_EDGE('',*,*,#29929,.F.) ;
#43136=ORIENTED_EDGE('',*,*,#29930,.F.) ;
#43137=ORIENTED_EDGE('',*,*,#29927,.T.) ;
#43138=ORIENTED_EDGE('',*,*,#29821,.F.) ;
#43139=ORIENTED_EDGE('',*,*,#29931,.T.) ;
#43140=ORIENTED_EDGE('',*,*,#29932,.F.) ;
#43141=ORIENTED_EDGE('',*,*,#29929,.T.) ;
#43142=ORIENTED_EDGE('',*,*,#29824,.F.) ;
#43143=ORIENTED_EDGE('',*,*,#29933,.F.) ;
#43144=ORIENTED_EDGE('',*,*,#29934,.F.) ;
#43145=ORIENTED_EDGE('',*,*,#29931,.F.) ;
#43146=ORIENTED_EDGE('',*,*,#29827,.F.) ;
#43147=ORIENTED_EDGE('',*,*,#29935,.F.) ;
#43148=ORIENTED_EDGE('',*,*,#29936,.F.) ;
#43149=ORIENTED_EDGE('',*,*,#29933,.T.) ;
#43150=ORIENTED_EDGE('',*,*,#29830,.F.) ;
#43151=ORIENTED_EDGE('',*,*,#29937,.F.) ;
#43152=ORIENTED_EDGE('',*,*,#29938,.F.) ;
#43153=ORIENTED_EDGE('',*,*,#29935,.T.) ;
#43154=ORIENTED_EDGE('',*,*,#29833,.F.) ;
#43155=ORIENTED_EDGE('',*,*,#29939,.T.) ;
#43156=ORIENTED_EDGE('',*,*,#29940,.F.) ;
#43157=ORIENTED_EDGE('',*,*,#29937,.T.) ;
#43158=ORIENTED_EDGE('',*,*,#29836,.F.) ;
#43159=ORIENTED_EDGE('',*,*,#29941,.F.) ;
#43160=ORIENTED_EDGE('',*,*,#29942,.F.) ;
#43161=ORIENTED_EDGE('',*,*,#29939,.F.) ;
#43162=ORIENTED_EDGE('',*,*,#29839,.F.) ;
#43163=ORIENTED_EDGE('',*,*,#29943,.F.) ;
#43164=ORIENTED_EDGE('',*,*,#29944,.F.) ;
#43165=ORIENTED_EDGE('',*,*,#29941,.T.) ;
#43166=ORIENTED_EDGE('',*,*,#29842,.F.) ;
#43167=ORIENTED_EDGE('',*,*,#29945,.F.) ;
#43168=ORIENTED_EDGE('',*,*,#29946,.F.) ;
#43169=ORIENTED_EDGE('',*,*,#29943,.T.) ;
#43170=ORIENTED_EDGE('',*,*,#29845,.F.) ;
#43171=ORIENTED_EDGE('',*,*,#29947,.T.) ;
#43172=ORIENTED_EDGE('',*,*,#29948,.F.) ;
#43173=ORIENTED_EDGE('',*,*,#29945,.T.) ;
#43174=ORIENTED_EDGE('',*,*,#29848,.F.) ;
#43175=ORIENTED_EDGE('',*,*,#29949,.F.) ;
#43176=ORIENTED_EDGE('',*,*,#29950,.F.) ;
#43177=ORIENTED_EDGE('',*,*,#29947,.F.) ;
#43178=ORIENTED_EDGE('',*,*,#29851,.F.) ;
#43179=ORIENTED_EDGE('',*,*,#29951,.F.) ;
#43180=ORIENTED_EDGE('',*,*,#29952,.F.) ;
#43181=ORIENTED_EDGE('',*,*,#29949,.T.) ;
#43182=ORIENTED_EDGE('',*,*,#29854,.F.) ;
#43183=ORIENTED_EDGE('',*,*,#29953,.F.) ;
#43184=ORIENTED_EDGE('',*,*,#29954,.F.) ;
#43185=ORIENTED_EDGE('',*,*,#29951,.T.) ;
#43186=ORIENTED_EDGE('',*,*,#29857,.F.) ;
#43187=ORIENTED_EDGE('',*,*,#29955,.T.) ;
#43188=ORIENTED_EDGE('',*,*,#29956,.F.) ;
#43189=ORIENTED_EDGE('',*,*,#29953,.T.) ;
#43190=ORIENTED_EDGE('',*,*,#29860,.F.) ;
#43191=ORIENTED_EDGE('',*,*,#29957,.F.) ;
#43192=ORIENTED_EDGE('',*,*,#29958,.F.) ;
#43193=ORIENTED_EDGE('',*,*,#29955,.F.) ;
#43194=ORIENTED_EDGE('',*,*,#29863,.F.) ;
#43195=ORIENTED_EDGE('',*,*,#29959,.F.) ;
#43196=ORIENTED_EDGE('',*,*,#29960,.F.) ;
#43197=ORIENTED_EDGE('',*,*,#29957,.T.) ;
#43198=ORIENTED_EDGE('',*,*,#29866,.F.) ;
#43199=ORIENTED_EDGE('',*,*,#29961,.F.) ;
#43200=ORIENTED_EDGE('',*,*,#29962,.F.) ;
#43201=ORIENTED_EDGE('',*,*,#29959,.T.) ;
#43202=ORIENTED_EDGE('',*,*,#29869,.F.) ;
#43203=ORIENTED_EDGE('',*,*,#29963,.T.) ;
#43204=ORIENTED_EDGE('',*,*,#29964,.F.) ;
#43205=ORIENTED_EDGE('',*,*,#29961,.T.) ;
#43206=ORIENTED_EDGE('',*,*,#29872,.F.) ;
#43207=ORIENTED_EDGE('',*,*,#29965,.F.) ;
#43208=ORIENTED_EDGE('',*,*,#29966,.F.) ;
#43209=ORIENTED_EDGE('',*,*,#29963,.F.) ;
#43210=ORIENTED_EDGE('',*,*,#29875,.F.) ;
#43211=ORIENTED_EDGE('',*,*,#29967,.F.) ;
#43212=ORIENTED_EDGE('',*,*,#29968,.F.) ;
#43213=ORIENTED_EDGE('',*,*,#29965,.T.) ;
#43214=ORIENTED_EDGE('',*,*,#29878,.F.) ;
#43215=ORIENTED_EDGE('',*,*,#29969,.F.) ;
#43216=ORIENTED_EDGE('',*,*,#29970,.F.) ;
#43217=ORIENTED_EDGE('',*,*,#29967,.T.) ;
#43218=ORIENTED_EDGE('',*,*,#29881,.F.) ;
#43219=ORIENTED_EDGE('',*,*,#29971,.T.) ;
#43220=ORIENTED_EDGE('',*,*,#29972,.F.) ;
#43221=ORIENTED_EDGE('',*,*,#29969,.T.) ;
#43222=ORIENTED_EDGE('',*,*,#29884,.F.) ;
#43223=ORIENTED_EDGE('',*,*,#29973,.F.) ;
#43224=ORIENTED_EDGE('',*,*,#29974,.F.) ;
#43225=ORIENTED_EDGE('',*,*,#29971,.F.) ;
#43226=ORIENTED_EDGE('',*,*,#29887,.F.) ;
#43227=ORIENTED_EDGE('',*,*,#29975,.F.) ;
#43228=ORIENTED_EDGE('',*,*,#29976,.F.) ;
#43229=ORIENTED_EDGE('',*,*,#29973,.T.) ;
#43230=ORIENTED_EDGE('',*,*,#29890,.F.) ;
#43231=ORIENTED_EDGE('',*,*,#29977,.F.) ;
#43232=ORIENTED_EDGE('',*,*,#29978,.F.) ;
#43233=ORIENTED_EDGE('',*,*,#29975,.T.) ;
#43234=ORIENTED_EDGE('',*,*,#29893,.F.) ;
#43235=ORIENTED_EDGE('',*,*,#29979,.T.) ;
#43236=ORIENTED_EDGE('',*,*,#29980,.F.) ;
#43237=ORIENTED_EDGE('',*,*,#29977,.T.) ;
#43238=ORIENTED_EDGE('',*,*,#29896,.F.) ;
#43239=ORIENTED_EDGE('',*,*,#29981,.F.) ;
#43240=ORIENTED_EDGE('',*,*,#29982,.F.) ;
#43241=ORIENTED_EDGE('',*,*,#29979,.F.) ;
#43242=ORIENTED_EDGE('',*,*,#29899,.F.) ;
#43243=ORIENTED_EDGE('',*,*,#29983,.F.) ;
#43244=ORIENTED_EDGE('',*,*,#29984,.F.) ;
#43245=ORIENTED_EDGE('',*,*,#29981,.T.) ;
#43246=ORIENTED_EDGE('',*,*,#29902,.F.) ;
#43247=ORIENTED_EDGE('',*,*,#29985,.F.) ;
#43248=ORIENTED_EDGE('',*,*,#29986,.F.) ;
#43249=ORIENTED_EDGE('',*,*,#29983,.T.) ;
#43250=ORIENTED_EDGE('',*,*,#29905,.F.) ;
#43251=ORIENTED_EDGE('',*,*,#29987,.T.) ;
#43252=ORIENTED_EDGE('',*,*,#29988,.F.) ;
#43253=ORIENTED_EDGE('',*,*,#29985,.T.) ;
#43254=ORIENTED_EDGE('',*,*,#29908,.F.) ;
#43255=ORIENTED_EDGE('',*,*,#29989,.F.) ;
#43256=ORIENTED_EDGE('',*,*,#29990,.F.) ;
#43257=ORIENTED_EDGE('',*,*,#29987,.F.) ;
#43258=ORIENTED_EDGE('',*,*,#29911,.F.) ;
#43259=ORIENTED_EDGE('',*,*,#29991,.F.) ;
#43260=ORIENTED_EDGE('',*,*,#29992,.F.) ;
#43261=ORIENTED_EDGE('',*,*,#29989,.T.) ;
#43262=ORIENTED_EDGE('',*,*,#29914,.F.) ;
#43263=ORIENTED_EDGE('',*,*,#29993,.F.) ;
#43264=ORIENTED_EDGE('',*,*,#29994,.F.) ;
#43265=ORIENTED_EDGE('',*,*,#29991,.T.) ;
#43266=ORIENTED_EDGE('',*,*,#29678,.F.) ;
#43267=ORIENTED_EDGE('',*,*,#29995,.T.) ;
#43268=ORIENTED_EDGE('',*,*,#29996,.F.) ;
#43269=ORIENTED_EDGE('',*,*,#29993,.T.) ;
#43270=ORIENTED_EDGE('',*,*,#29807,.F.) ;
#43271=ORIENTED_EDGE('',*,*,#29804,.F.) ;
#43272=ORIENTED_EDGE('',*,*,#29801,.F.) ;
#43273=ORIENTED_EDGE('',*,*,#29997,.F.) ;
#43274=ORIENTED_EDGE('',*,*,#29819,.F.) ;
#43275=ORIENTED_EDGE('',*,*,#29816,.F.) ;
#43276=ORIENTED_EDGE('',*,*,#29813,.F.) ;
#43277=ORIENTED_EDGE('',*,*,#29998,.F.) ;
#43278=ORIENTED_EDGE('',*,*,#29788,.F.) ;
#43279=ORIENTED_EDGE('',*,*,#29999,.F.) ;
#43280=ORIENTED_EDGE('',*,*,#29794,.F.) ;
#43281=ORIENTED_EDGE('',*,*,#29791,.F.) ;
#43282=ORIENTED_EDGE('',*,*,#29831,.F.) ;
#43283=ORIENTED_EDGE('',*,*,#29828,.F.) ;
#43284=ORIENTED_EDGE('',*,*,#29825,.F.) ;
#43285=ORIENTED_EDGE('',*,*,#30000,.F.) ;
#43286=ORIENTED_EDGE('',*,*,#29776,.F.) ;
#43287=ORIENTED_EDGE('',*,*,#30001,.F.) ;
#43288=ORIENTED_EDGE('',*,*,#29782,.F.) ;
#43289=ORIENTED_EDGE('',*,*,#29779,.F.) ;
#43290=ORIENTED_EDGE('',*,*,#29843,.F.) ;
#43291=ORIENTED_EDGE('',*,*,#29840,.F.) ;
#43292=ORIENTED_EDGE('',*,*,#29837,.F.) ;
#43293=ORIENTED_EDGE('',*,*,#30002,.F.) ;
#43294=ORIENTED_EDGE('',*,*,#29764,.F.) ;
#43295=ORIENTED_EDGE('',*,*,#30003,.F.) ;
#43296=ORIENTED_EDGE('',*,*,#29770,.F.) ;
#43297=ORIENTED_EDGE('',*,*,#29767,.F.) ;
#43298=ORIENTED_EDGE('',*,*,#29855,.F.) ;
#43299=ORIENTED_EDGE('',*,*,#29852,.F.) ;
#43300=ORIENTED_EDGE('',*,*,#29849,.F.) ;
#43301=ORIENTED_EDGE('',*,*,#30004,.F.) ;
#43302=ORIENTED_EDGE('',*,*,#29752,.F.) ;
#43303=ORIENTED_EDGE('',*,*,#30005,.F.) ;
#43304=ORIENTED_EDGE('',*,*,#29758,.F.) ;
#43305=ORIENTED_EDGE('',*,*,#29755,.F.) ;
#43306=ORIENTED_EDGE('',*,*,#29867,.F.) ;
#43307=ORIENTED_EDGE('',*,*,#29864,.F.) ;
#43308=ORIENTED_EDGE('',*,*,#29861,.F.) ;
#43309=ORIENTED_EDGE('',*,*,#30006,.F.) ;
#43310=ORIENTED_EDGE('',*,*,#29740,.F.) ;
#43311=ORIENTED_EDGE('',*,*,#30007,.F.) ;
#43312=ORIENTED_EDGE('',*,*,#29746,.F.) ;
#43313=ORIENTED_EDGE('',*,*,#29743,.F.) ;
#43314=ORIENTED_EDGE('',*,*,#29879,.F.) ;
#43315=ORIENTED_EDGE('',*,*,#29876,.F.) ;
#43316=ORIENTED_EDGE('',*,*,#29873,.F.) ;
#43317=ORIENTED_EDGE('',*,*,#30008,.F.) ;
#43318=ORIENTED_EDGE('',*,*,#29728,.F.) ;
#43319=ORIENTED_EDGE('',*,*,#30009,.F.) ;
#43320=ORIENTED_EDGE('',*,*,#29734,.F.) ;
#43321=ORIENTED_EDGE('',*,*,#29731,.F.) ;
#43322=ORIENTED_EDGE('',*,*,#29891,.F.) ;
#43323=ORIENTED_EDGE('',*,*,#29888,.F.) ;
#43324=ORIENTED_EDGE('',*,*,#29885,.F.) ;
#43325=ORIENTED_EDGE('',*,*,#30010,.F.) ;
#43326=ORIENTED_EDGE('',*,*,#29716,.F.) ;
#43327=ORIENTED_EDGE('',*,*,#30011,.F.) ;
#43328=ORIENTED_EDGE('',*,*,#29722,.F.) ;
#43329=ORIENTED_EDGE('',*,*,#29719,.F.) ;
#43330=ORIENTED_EDGE('',*,*,#29903,.F.) ;
#43331=ORIENTED_EDGE('',*,*,#29900,.F.) ;
#43332=ORIENTED_EDGE('',*,*,#29897,.F.) ;
#43333=ORIENTED_EDGE('',*,*,#30012,.F.) ;
#43334=ORIENTED_EDGE('',*,*,#29704,.F.) ;
#43335=ORIENTED_EDGE('',*,*,#30013,.F.) ;
#43336=ORIENTED_EDGE('',*,*,#29710,.F.) ;
#43337=ORIENTED_EDGE('',*,*,#29707,.F.) ;
#43338=ORIENTED_EDGE('',*,*,#29915,.F.) ;
#43339=ORIENTED_EDGE('',*,*,#29912,.F.) ;
#43340=ORIENTED_EDGE('',*,*,#29909,.F.) ;
#43341=ORIENTED_EDGE('',*,*,#30014,.F.) ;
#43342=ORIENTED_EDGE('',*,*,#29692,.F.) ;
#43343=ORIENTED_EDGE('',*,*,#30015,.F.) ;
#43344=ORIENTED_EDGE('',*,*,#30016,.F.) ;
#43345=ORIENTED_EDGE('',*,*,#29698,.F.) ;
#43346=ORIENTED_EDGE('',*,*,#29695,.F.) ;
#43347=ORIENTED_EDGE('',*,*,#29671,.F.) ;
#43348=ORIENTED_EDGE('',*,*,#29672,.F.) ;
#43349=ORIENTED_EDGE('',*,*,#30017,.T.) ;
#43350=ORIENTED_EDGE('',*,*,#30015,.T.) ;
#43351=ORIENTED_EDGE('',*,*,#29689,.T.) ;
#43352=ORIENTED_EDGE('',*,*,#30018,.T.) ;
#43353=ORIENTED_EDGE('',*,*,#29676,.T.) ;
#43354=ORIENTED_EDGE('',*,*,#30014,.T.) ;
#43355=ORIENTED_EDGE('',*,*,#29906,.T.) ;
#43356=ORIENTED_EDGE('',*,*,#30012,.T.) ;
#43357=ORIENTED_EDGE('',*,*,#29894,.T.) ;
#43358=ORIENTED_EDGE('',*,*,#30010,.T.) ;
#43359=ORIENTED_EDGE('',*,*,#29882,.T.) ;
#43360=ORIENTED_EDGE('',*,*,#30008,.T.) ;
#43361=ORIENTED_EDGE('',*,*,#29870,.T.) ;
#43362=ORIENTED_EDGE('',*,*,#30006,.T.) ;
#43363=ORIENTED_EDGE('',*,*,#29858,.T.) ;
#43364=ORIENTED_EDGE('',*,*,#30004,.T.) ;
#43365=ORIENTED_EDGE('',*,*,#29846,.T.) ;
#43366=ORIENTED_EDGE('',*,*,#30002,.T.) ;
#43367=ORIENTED_EDGE('',*,*,#29834,.T.) ;
#43368=ORIENTED_EDGE('',*,*,#30000,.T.) ;
#43369=ORIENTED_EDGE('',*,*,#29822,.T.) ;
#43370=ORIENTED_EDGE('',*,*,#29998,.T.) ;
#43371=ORIENTED_EDGE('',*,*,#29810,.T.) ;
#43372=ORIENTED_EDGE('',*,*,#29997,.T.) ;
#43373=ORIENTED_EDGE('',*,*,#29797,.T.) ;
#43374=ORIENTED_EDGE('',*,*,#29999,.T.) ;
#43375=ORIENTED_EDGE('',*,*,#29785,.T.) ;
#43376=ORIENTED_EDGE('',*,*,#30001,.T.) ;
#43377=ORIENTED_EDGE('',*,*,#29773,.T.) ;
#43378=ORIENTED_EDGE('',*,*,#30003,.T.) ;
#43379=ORIENTED_EDGE('',*,*,#29761,.T.) ;
#43380=ORIENTED_EDGE('',*,*,#30005,.T.) ;
#43381=ORIENTED_EDGE('',*,*,#29749,.T.) ;
#43382=ORIENTED_EDGE('',*,*,#30007,.T.) ;
#43383=ORIENTED_EDGE('',*,*,#29737,.T.) ;
#43384=ORIENTED_EDGE('',*,*,#30009,.T.) ;
#43385=ORIENTED_EDGE('',*,*,#29725,.T.) ;
#43386=ORIENTED_EDGE('',*,*,#30011,.T.) ;
#43387=ORIENTED_EDGE('',*,*,#29713,.T.) ;
#43388=ORIENTED_EDGE('',*,*,#30013,.T.) ;
#43389=ORIENTED_EDGE('',*,*,#29701,.T.) ;
#43390=ORIENTED_EDGE('',*,*,#30016,.T.) ;
#43391=ORIENTED_EDGE('',*,*,#30017,.F.) ;
#43392=ORIENTED_EDGE('',*,*,#29680,.F.) ;
#43393=ORIENTED_EDGE('',*,*,#30018,.F.) ;
#43394=ORIENTED_EDGE('',*,*,#29686,.F.) ;
#43395=ORIENTED_EDGE('',*,*,#29683,.F.) ;
#43396=ORIENTED_EDGE('',*,*,#29674,.F.) ;
#43397=ORIENTED_EDGE('',*,*,#29675,.F.) ;
#43398=ORIENTED_EDGE('',*,*,#30019,.T.) ;
#43399=ORIENTED_EDGE('',*,*,#30020,.T.) ;
#43400=ORIENTED_EDGE('',*,*,#30021,.F.) ;
#43401=ORIENTED_EDGE('',*,*,#30022,.T.) ;
#43402=ORIENTED_EDGE('',*,*,#30023,.F.) ;
#43403=ORIENTED_EDGE('',*,*,#30024,.T.) ;
#43404=ORIENTED_EDGE('',*,*,#30025,.F.) ;
#43405=ORIENTED_EDGE('',*,*,#30026,.T.) ;
#43406=ORIENTED_EDGE('',*,*,#30027,.F.) ;
#43407=ORIENTED_EDGE('',*,*,#30028,.T.) ;
#43408=ORIENTED_EDGE('',*,*,#30029,.F.) ;
#43409=ORIENTED_EDGE('',*,*,#30030,.T.) ;
#43410=ORIENTED_EDGE('',*,*,#30031,.F.) ;
#43411=ORIENTED_EDGE('',*,*,#30032,.T.) ;
#43412=ORIENTED_EDGE('',*,*,#30033,.F.) ;
#43413=ORIENTED_EDGE('',*,*,#30034,.T.) ;
#43414=ORIENTED_EDGE('',*,*,#30035,.F.) ;
#43415=ORIENTED_EDGE('',*,*,#30036,.T.) ;
#43416=ORIENTED_EDGE('',*,*,#30037,.F.) ;
#43417=ORIENTED_EDGE('',*,*,#30038,.T.) ;
#43418=ORIENTED_EDGE('',*,*,#30039,.F.) ;
#43419=ORIENTED_EDGE('',*,*,#30040,.T.) ;
#43420=ORIENTED_EDGE('',*,*,#30041,.F.) ;
#43421=ORIENTED_EDGE('',*,*,#30042,.T.) ;
#43422=ORIENTED_EDGE('',*,*,#30043,.F.) ;
#43423=ORIENTED_EDGE('',*,*,#30044,.T.) ;
#43424=ORIENTED_EDGE('',*,*,#30045,.F.) ;
#43425=ORIENTED_EDGE('',*,*,#30046,.T.) ;
#43426=ORIENTED_EDGE('',*,*,#30047,.F.) ;
#43427=ORIENTED_EDGE('',*,*,#30048,.T.) ;
#43428=ORIENTED_EDGE('',*,*,#30049,.F.) ;
#43429=ORIENTED_EDGE('',*,*,#30050,.T.) ;
#43430=ORIENTED_EDGE('',*,*,#30051,.F.) ;
#43431=ORIENTED_EDGE('',*,*,#30052,.T.) ;
#43432=ORIENTED_EDGE('',*,*,#30053,.F.) ;
#43433=ORIENTED_EDGE('',*,*,#30054,.T.) ;
#43434=ORIENTED_EDGE('',*,*,#30055,.F.) ;
#43435=ORIENTED_EDGE('',*,*,#30056,.T.) ;
#43436=ORIENTED_EDGE('',*,*,#30057,.F.) ;
#43437=ORIENTED_EDGE('',*,*,#30058,.T.) ;
#43438=ORIENTED_EDGE('',*,*,#30059,.F.) ;
#43439=ORIENTED_EDGE('',*,*,#30060,.T.) ;
#43440=ORIENTED_EDGE('',*,*,#30019,.F.) ;
#43441=ORIENTED_EDGE('',*,*,#30058,.F.) ;
#43442=ORIENTED_EDGE('',*,*,#30061,.F.) ;
#43443=ORIENTED_EDGE('',*,*,#30062,.F.) ;
#43444=ORIENTED_EDGE('',*,*,#30063,.F.) ;
#43445=ORIENTED_EDGE('',*,*,#30056,.F.) ;
#43446=ORIENTED_EDGE('',*,*,#30064,.F.) ;
#43447=ORIENTED_EDGE('',*,*,#30065,.F.) ;
#43448=ORIENTED_EDGE('',*,*,#30066,.F.) ;
#43449=ORIENTED_EDGE('',*,*,#30054,.F.) ;
#43450=ORIENTED_EDGE('',*,*,#30067,.F.) ;
#43451=ORIENTED_EDGE('',*,*,#30068,.F.) ;
#43452=ORIENTED_EDGE('',*,*,#30069,.F.) ;
#43453=ORIENTED_EDGE('',*,*,#30052,.F.) ;
#43454=ORIENTED_EDGE('',*,*,#30070,.F.) ;
#43455=ORIENTED_EDGE('',*,*,#30071,.F.) ;
#43456=ORIENTED_EDGE('',*,*,#30072,.F.) ;
#43457=ORIENTED_EDGE('',*,*,#30050,.F.) ;
#43458=ORIENTED_EDGE('',*,*,#30073,.F.) ;
#43459=ORIENTED_EDGE('',*,*,#30074,.F.) ;
#43460=ORIENTED_EDGE('',*,*,#30075,.F.) ;
#43461=ORIENTED_EDGE('',*,*,#30048,.F.) ;
#43462=ORIENTED_EDGE('',*,*,#30076,.F.) ;
#43463=ORIENTED_EDGE('',*,*,#30077,.F.) ;
#43464=ORIENTED_EDGE('',*,*,#30078,.F.) ;
#43465=ORIENTED_EDGE('',*,*,#30046,.F.) ;
#43466=ORIENTED_EDGE('',*,*,#30079,.F.) ;
#43467=ORIENTED_EDGE('',*,*,#30080,.F.) ;
#43468=ORIENTED_EDGE('',*,*,#30081,.F.) ;
#43469=ORIENTED_EDGE('',*,*,#30044,.F.) ;
#43470=ORIENTED_EDGE('',*,*,#30082,.F.) ;
#43471=ORIENTED_EDGE('',*,*,#30083,.F.) ;
#43472=ORIENTED_EDGE('',*,*,#30084,.F.) ;
#43473=ORIENTED_EDGE('',*,*,#30042,.F.) ;
#43474=ORIENTED_EDGE('',*,*,#30085,.F.) ;
#43475=ORIENTED_EDGE('',*,*,#30086,.F.) ;
#43476=ORIENTED_EDGE('',*,*,#30087,.F.) ;
#43477=ORIENTED_EDGE('',*,*,#30040,.F.) ;
#43478=ORIENTED_EDGE('',*,*,#30088,.F.) ;
#43479=ORIENTED_EDGE('',*,*,#30089,.F.) ;
#43480=ORIENTED_EDGE('',*,*,#30090,.F.) ;
#43481=ORIENTED_EDGE('',*,*,#30038,.F.) ;
#43482=ORIENTED_EDGE('',*,*,#30091,.F.) ;
#43483=ORIENTED_EDGE('',*,*,#30092,.F.) ;
#43484=ORIENTED_EDGE('',*,*,#30093,.F.) ;
#43485=ORIENTED_EDGE('',*,*,#30036,.F.) ;
#43486=ORIENTED_EDGE('',*,*,#30094,.F.) ;
#43487=ORIENTED_EDGE('',*,*,#30095,.F.) ;
#43488=ORIENTED_EDGE('',*,*,#30096,.F.) ;
#43489=ORIENTED_EDGE('',*,*,#30034,.F.) ;
#43490=ORIENTED_EDGE('',*,*,#30097,.F.) ;
#43491=ORIENTED_EDGE('',*,*,#30098,.F.) ;
#43492=ORIENTED_EDGE('',*,*,#30099,.F.) ;
#43493=ORIENTED_EDGE('',*,*,#30032,.F.) ;
#43494=ORIENTED_EDGE('',*,*,#30100,.F.) ;
#43495=ORIENTED_EDGE('',*,*,#30101,.F.) ;
#43496=ORIENTED_EDGE('',*,*,#30102,.F.) ;
#43497=ORIENTED_EDGE('',*,*,#30030,.F.) ;
#43498=ORIENTED_EDGE('',*,*,#30103,.F.) ;
#43499=ORIENTED_EDGE('',*,*,#30104,.F.) ;
#43500=ORIENTED_EDGE('',*,*,#30105,.F.) ;
#43501=ORIENTED_EDGE('',*,*,#30028,.F.) ;
#43502=ORIENTED_EDGE('',*,*,#30106,.F.) ;
#43503=ORIENTED_EDGE('',*,*,#30107,.F.) ;
#43504=ORIENTED_EDGE('',*,*,#30108,.F.) ;
#43505=ORIENTED_EDGE('',*,*,#30026,.F.) ;
#43506=ORIENTED_EDGE('',*,*,#30109,.F.) ;
#43507=ORIENTED_EDGE('',*,*,#30110,.F.) ;
#43508=ORIENTED_EDGE('',*,*,#30111,.F.) ;
#43509=ORIENTED_EDGE('',*,*,#30024,.F.) ;
#43510=ORIENTED_EDGE('',*,*,#30112,.F.) ;
#43511=ORIENTED_EDGE('',*,*,#30113,.F.) ;
#43512=ORIENTED_EDGE('',*,*,#30114,.F.) ;
#43513=ORIENTED_EDGE('',*,*,#30022,.F.) ;
#43514=ORIENTED_EDGE('',*,*,#30115,.F.) ;
#43515=ORIENTED_EDGE('',*,*,#30116,.F.) ;
#43516=ORIENTED_EDGE('',*,*,#30117,.F.) ;
#43517=ORIENTED_EDGE('',*,*,#30060,.F.) ;
#43518=ORIENTED_EDGE('',*,*,#30118,.F.) ;
#43519=ORIENTED_EDGE('',*,*,#30119,.F.) ;
#43520=ORIENTED_EDGE('',*,*,#30120,.F.) ;
#43521=ORIENTED_EDGE('',*,*,#30020,.F.) ;
#43522=ORIENTED_EDGE('',*,*,#30039,.T.) ;
#43523=ORIENTED_EDGE('',*,*,#30121,.T.) ;
#43524=ORIENTED_EDGE('',*,*,#30122,.T.) ;
#43525=ORIENTED_EDGE('',*,*,#30123,.F.) ;
#43526=ORIENTED_EDGE('',*,*,#30093,.T.) ;
#43527=ORIENTED_EDGE('',*,*,#30124,.T.) ;
#43528=ORIENTED_EDGE('',*,*,#30125,.T.) ;
#43529=ORIENTED_EDGE('',*,*,#30121,.F.) ;
#43530=ORIENTED_EDGE('',*,*,#30126,.T.) ;
#43531=ORIENTED_EDGE('',*,*,#30127,.T.) ;
#43532=ORIENTED_EDGE('',*,*,#30088,.T.) ;
#43533=ORIENTED_EDGE('',*,*,#30123,.T.) ;
#43534=ORIENTED_EDGE('',*,*,#30091,.T.) ;
#43535=ORIENTED_EDGE('',*,*,#30128,.T.) ;
#43536=ORIENTED_EDGE('',*,*,#30129,.T.) ;
#43537=ORIENTED_EDGE('',*,*,#30130,.T.) ;
#43538=ORIENTED_EDGE('',*,*,#30037,.T.) ;
#43539=ORIENTED_EDGE('',*,*,#30131,.T.) ;
#43540=ORIENTED_EDGE('',*,*,#29996,.T.) ;
#43541=ORIENTED_EDGE('',*,*,#30128,.F.) ;
#43542=ORIENTED_EDGE('',*,*,#30096,.T.) ;
#43543=ORIENTED_EDGE('',*,*,#30132,.T.) ;
#43544=ORIENTED_EDGE('',*,*,#29994,.T.) ;
#43545=ORIENTED_EDGE('',*,*,#30131,.F.) ;
#43546=ORIENTED_EDGE('',*,*,#30133,.T.) ;
#43547=ORIENTED_EDGE('',*,*,#30134,.T.) ;
#43548=ORIENTED_EDGE('',*,*,#30085,.T.) ;
#43549=ORIENTED_EDGE('',*,*,#30135,.T.) ;
#43550=ORIENTED_EDGE('',*,*,#30094,.T.) ;
#43551=ORIENTED_EDGE('',*,*,#30136,.T.) ;
#43552=ORIENTED_EDGE('',*,*,#29990,.T.) ;
#43553=ORIENTED_EDGE('',*,*,#30137,.T.) ;
#43554=ORIENTED_EDGE('',*,*,#30035,.T.) ;
#43555=ORIENTED_EDGE('',*,*,#30138,.T.) ;
#43556=ORIENTED_EDGE('',*,*,#29988,.T.) ;
#43557=ORIENTED_EDGE('',*,*,#30136,.F.) ;
#43558=ORIENTED_EDGE('',*,*,#30099,.T.) ;
#43559=ORIENTED_EDGE('',*,*,#30139,.T.) ;
#43560=ORIENTED_EDGE('',*,*,#29986,.T.) ;
#43561=ORIENTED_EDGE('',*,*,#30138,.F.) ;
#43562=ORIENTED_EDGE('',*,*,#30140,.T.) ;
#43563=ORIENTED_EDGE('',*,*,#30141,.T.) ;
#43564=ORIENTED_EDGE('',*,*,#30082,.T.) ;
#43565=ORIENTED_EDGE('',*,*,#30142,.T.) ;
#43566=ORIENTED_EDGE('',*,*,#30097,.T.) ;
#43567=ORIENTED_EDGE('',*,*,#30143,.T.) ;
#43568=ORIENTED_EDGE('',*,*,#29982,.T.) ;
#43569=ORIENTED_EDGE('',*,*,#30144,.T.) ;
#43570=ORIENTED_EDGE('',*,*,#30033,.T.) ;
#43571=ORIENTED_EDGE('',*,*,#30145,.T.) ;
#43572=ORIENTED_EDGE('',*,*,#29980,.T.) ;
#43573=ORIENTED_EDGE('',*,*,#30143,.F.) ;
#43574=ORIENTED_EDGE('',*,*,#30102,.T.) ;
#43575=ORIENTED_EDGE('',*,*,#30146,.T.) ;
#43576=ORIENTED_EDGE('',*,*,#29978,.T.) ;
#43577=ORIENTED_EDGE('',*,*,#30145,.F.) ;
#43578=ORIENTED_EDGE('',*,*,#30147,.T.) ;
#43579=ORIENTED_EDGE('',*,*,#30148,.T.) ;
#43580=ORIENTED_EDGE('',*,*,#30079,.T.) ;
#43581=ORIENTED_EDGE('',*,*,#30149,.T.) ;
#43582=ORIENTED_EDGE('',*,*,#30100,.T.) ;
#43583=ORIENTED_EDGE('',*,*,#30150,.T.) ;
#43584=ORIENTED_EDGE('',*,*,#29974,.T.) ;
#43585=ORIENTED_EDGE('',*,*,#30151,.T.) ;
#43586=ORIENTED_EDGE('',*,*,#30031,.T.) ;
#43587=ORIENTED_EDGE('',*,*,#30152,.T.) ;
#43588=ORIENTED_EDGE('',*,*,#29972,.T.) ;
#43589=ORIENTED_EDGE('',*,*,#30150,.F.) ;
#43590=ORIENTED_EDGE('',*,*,#30105,.T.) ;
#43591=ORIENTED_EDGE('',*,*,#30153,.T.) ;
#43592=ORIENTED_EDGE('',*,*,#29970,.T.) ;
#43593=ORIENTED_EDGE('',*,*,#30152,.F.) ;
#43594=ORIENTED_EDGE('',*,*,#30154,.T.) ;
#43595=ORIENTED_EDGE('',*,*,#30155,.T.) ;
#43596=ORIENTED_EDGE('',*,*,#30076,.T.) ;
#43597=ORIENTED_EDGE('',*,*,#30156,.T.) ;
#43598=ORIENTED_EDGE('',*,*,#30103,.T.) ;
#43599=ORIENTED_EDGE('',*,*,#30157,.T.) ;
#43600=ORIENTED_EDGE('',*,*,#29966,.T.) ;
#43601=ORIENTED_EDGE('',*,*,#30158,.T.) ;
#43602=ORIENTED_EDGE('',*,*,#30029,.T.) ;
#43603=ORIENTED_EDGE('',*,*,#30159,.T.) ;
#43604=ORIENTED_EDGE('',*,*,#29964,.T.) ;
#43605=ORIENTED_EDGE('',*,*,#30157,.F.) ;
#43606=ORIENTED_EDGE('',*,*,#30108,.T.) ;
#43607=ORIENTED_EDGE('',*,*,#30160,.T.) ;
#43608=ORIENTED_EDGE('',*,*,#29962,.T.) ;
#43609=ORIENTED_EDGE('',*,*,#30159,.F.) ;
#43610=ORIENTED_EDGE('',*,*,#30161,.T.) ;
#43611=ORIENTED_EDGE('',*,*,#30162,.T.) ;
#43612=ORIENTED_EDGE('',*,*,#30073,.T.) ;
#43613=ORIENTED_EDGE('',*,*,#30163,.T.) ;
#43614=ORIENTED_EDGE('',*,*,#30106,.T.) ;
#43615=ORIENTED_EDGE('',*,*,#30164,.T.) ;
#43616=ORIENTED_EDGE('',*,*,#29958,.T.) ;
#43617=ORIENTED_EDGE('',*,*,#30165,.T.) ;
#43618=ORIENTED_EDGE('',*,*,#30027,.T.) ;
#43619=ORIENTED_EDGE('',*,*,#30166,.T.) ;
#43620=ORIENTED_EDGE('',*,*,#29956,.T.) ;
#43621=ORIENTED_EDGE('',*,*,#30164,.F.) ;
#43622=ORIENTED_EDGE('',*,*,#30111,.T.) ;
#43623=ORIENTED_EDGE('',*,*,#30167,.T.) ;
#43624=ORIENTED_EDGE('',*,*,#29954,.T.) ;
#43625=ORIENTED_EDGE('',*,*,#30166,.F.) ;
#43626=ORIENTED_EDGE('',*,*,#30168,.T.) ;
#43627=ORIENTED_EDGE('',*,*,#30169,.T.) ;
#43628=ORIENTED_EDGE('',*,*,#30070,.T.) ;
#43629=ORIENTED_EDGE('',*,*,#30170,.T.) ;
#43630=ORIENTED_EDGE('',*,*,#30109,.T.) ;
#43631=ORIENTED_EDGE('',*,*,#30171,.T.) ;
#43632=ORIENTED_EDGE('',*,*,#29950,.T.) ;
#43633=ORIENTED_EDGE('',*,*,#30172,.T.) ;
#43634=ORIENTED_EDGE('',*,*,#30025,.T.) ;
#43635=ORIENTED_EDGE('',*,*,#30173,.T.) ;
#43636=ORIENTED_EDGE('',*,*,#29948,.T.) ;
#43637=ORIENTED_EDGE('',*,*,#30171,.F.) ;
#43638=ORIENTED_EDGE('',*,*,#30114,.T.) ;
#43639=ORIENTED_EDGE('',*,*,#30174,.T.) ;
#43640=ORIENTED_EDGE('',*,*,#29946,.T.) ;
#43641=ORIENTED_EDGE('',*,*,#30173,.F.) ;
#43642=ORIENTED_EDGE('',*,*,#30175,.T.) ;
#43643=ORIENTED_EDGE('',*,*,#30176,.T.) ;
#43644=ORIENTED_EDGE('',*,*,#30067,.T.) ;
#43645=ORIENTED_EDGE('',*,*,#30177,.T.) ;
#43646=ORIENTED_EDGE('',*,*,#30112,.T.) ;
#43647=ORIENTED_EDGE('',*,*,#30178,.T.) ;
#43648=ORIENTED_EDGE('',*,*,#29942,.T.) ;
#43649=ORIENTED_EDGE('',*,*,#30179,.T.) ;
#43650=ORIENTED_EDGE('',*,*,#30023,.T.) ;
#43651=ORIENTED_EDGE('',*,*,#30180,.T.) ;
#43652=ORIENTED_EDGE('',*,*,#29940,.T.) ;
#43653=ORIENTED_EDGE('',*,*,#30178,.F.) ;
#43654=ORIENTED_EDGE('',*,*,#30117,.T.) ;
#43655=ORIENTED_EDGE('',*,*,#30181,.T.) ;
#43656=ORIENTED_EDGE('',*,*,#29938,.T.) ;
#43657=ORIENTED_EDGE('',*,*,#30180,.F.) ;
#43658=ORIENTED_EDGE('',*,*,#30182,.T.) ;
#43659=ORIENTED_EDGE('',*,*,#30183,.T.) ;
#43660=ORIENTED_EDGE('',*,*,#30064,.T.) ;
#43661=ORIENTED_EDGE('',*,*,#30184,.T.) ;
#43662=ORIENTED_EDGE('',*,*,#30115,.T.) ;
#43663=ORIENTED_EDGE('',*,*,#30185,.T.) ;
#43664=ORIENTED_EDGE('',*,*,#29934,.T.) ;
#43665=ORIENTED_EDGE('',*,*,#30186,.T.) ;
#43666=ORIENTED_EDGE('',*,*,#30021,.T.) ;
#43667=ORIENTED_EDGE('',*,*,#30187,.T.) ;
#43668=ORIENTED_EDGE('',*,*,#29932,.T.) ;
#43669=ORIENTED_EDGE('',*,*,#30185,.F.) ;
#43670=ORIENTED_EDGE('',*,*,#30120,.T.) ;
#43671=ORIENTED_EDGE('',*,*,#30188,.T.) ;
#43672=ORIENTED_EDGE('',*,*,#29930,.T.) ;
#43673=ORIENTED_EDGE('',*,*,#30187,.F.) ;
#43674=ORIENTED_EDGE('',*,*,#29917,.T.) ;
#43675=ORIENTED_EDGE('',*,*,#30189,.T.) ;
#43676=ORIENTED_EDGE('',*,*,#30061,.T.) ;
#43677=ORIENTED_EDGE('',*,*,#30190,.T.) ;
#43678=ORIENTED_EDGE('',*,*,#30118,.T.) ;
#43679=ORIENTED_EDGE('',*,*,#30191,.T.) ;
#43680=ORIENTED_EDGE('',*,*,#29926,.T.) ;
#43681=ORIENTED_EDGE('',*,*,#30192,.T.) ;
#43682=ORIENTED_EDGE('',*,*,#30059,.T.) ;
#43683=ORIENTED_EDGE('',*,*,#30193,.T.) ;
#43684=ORIENTED_EDGE('',*,*,#29924,.T.) ;
#43685=ORIENTED_EDGE('',*,*,#30191,.F.) ;
#43686=ORIENTED_EDGE('',*,*,#29922,.T.) ;
#43687=ORIENTED_EDGE('',*,*,#30193,.F.) ;
#43688=ORIENTED_EDGE('',*,*,#30063,.T.) ;
#43689=ORIENTED_EDGE('',*,*,#30194,.T.) ;
#43690=ORIENTED_EDGE('',*,*,#29920,.T.) ;
#43691=ORIENTED_EDGE('',*,*,#30194,.F.) ;
#43692=ORIENTED_EDGE('',*,*,#30062,.T.) ;
#43693=ORIENTED_EDGE('',*,*,#30189,.F.) ;
#43694=ORIENTED_EDGE('',*,*,#30119,.T.) ;
#43695=ORIENTED_EDGE('',*,*,#30192,.F.) ;
#43696=ORIENTED_EDGE('',*,*,#29928,.T.) ;
#43697=ORIENTED_EDGE('',*,*,#30188,.F.) ;
#43698=ORIENTED_EDGE('',*,*,#30195,.T.) ;
#43699=ORIENTED_EDGE('',*,*,#30190,.F.) ;
#43700=ORIENTED_EDGE('',*,*,#30057,.T.) ;
#43701=ORIENTED_EDGE('',*,*,#30196,.T.) ;
#43702=ORIENTED_EDGE('',*,*,#30197,.T.) ;
#43703=ORIENTED_EDGE('',*,*,#30196,.F.) ;
#43704=ORIENTED_EDGE('',*,*,#30066,.T.) ;
#43705=ORIENTED_EDGE('',*,*,#30198,.T.) ;
#43706=ORIENTED_EDGE('',*,*,#30199,.T.) ;
#43707=ORIENTED_EDGE('',*,*,#30198,.F.) ;
#43708=ORIENTED_EDGE('',*,*,#30065,.T.) ;
#43709=ORIENTED_EDGE('',*,*,#30183,.F.) ;
#43710=ORIENTED_EDGE('',*,*,#30116,.T.) ;
#43711=ORIENTED_EDGE('',*,*,#30186,.F.) ;
#43712=ORIENTED_EDGE('',*,*,#29936,.T.) ;
#43713=ORIENTED_EDGE('',*,*,#30181,.F.) ;
#43714=ORIENTED_EDGE('',*,*,#30200,.T.) ;
#43715=ORIENTED_EDGE('',*,*,#30184,.F.) ;
#43716=ORIENTED_EDGE('',*,*,#30055,.T.) ;
#43717=ORIENTED_EDGE('',*,*,#30201,.T.) ;
#43718=ORIENTED_EDGE('',*,*,#30202,.T.) ;
#43719=ORIENTED_EDGE('',*,*,#30201,.F.) ;
#43720=ORIENTED_EDGE('',*,*,#30069,.T.) ;
#43721=ORIENTED_EDGE('',*,*,#30203,.T.) ;
#43722=ORIENTED_EDGE('',*,*,#30204,.T.) ;
#43723=ORIENTED_EDGE('',*,*,#30203,.F.) ;
#43724=ORIENTED_EDGE('',*,*,#30068,.T.) ;
#43725=ORIENTED_EDGE('',*,*,#30176,.F.) ;
#43726=ORIENTED_EDGE('',*,*,#30113,.T.) ;
#43727=ORIENTED_EDGE('',*,*,#30179,.F.) ;
#43728=ORIENTED_EDGE('',*,*,#29944,.T.) ;
#43729=ORIENTED_EDGE('',*,*,#30174,.F.) ;
#43730=ORIENTED_EDGE('',*,*,#30205,.T.) ;
#43731=ORIENTED_EDGE('',*,*,#30177,.F.) ;
#43732=ORIENTED_EDGE('',*,*,#30053,.T.) ;
#43733=ORIENTED_EDGE('',*,*,#30206,.T.) ;
#43734=ORIENTED_EDGE('',*,*,#30207,.T.) ;
#43735=ORIENTED_EDGE('',*,*,#30206,.F.) ;
#43736=ORIENTED_EDGE('',*,*,#30072,.T.) ;
#43737=ORIENTED_EDGE('',*,*,#30208,.T.) ;
#43738=ORIENTED_EDGE('',*,*,#30209,.T.) ;
#43739=ORIENTED_EDGE('',*,*,#30208,.F.) ;
#43740=ORIENTED_EDGE('',*,*,#30071,.T.) ;
#43741=ORIENTED_EDGE('',*,*,#30169,.F.) ;
#43742=ORIENTED_EDGE('',*,*,#30110,.T.) ;
#43743=ORIENTED_EDGE('',*,*,#30172,.F.) ;
#43744=ORIENTED_EDGE('',*,*,#29952,.T.) ;
#43745=ORIENTED_EDGE('',*,*,#30167,.F.) ;
#43746=ORIENTED_EDGE('',*,*,#30210,.T.) ;
#43747=ORIENTED_EDGE('',*,*,#30170,.F.) ;
#43748=ORIENTED_EDGE('',*,*,#30051,.T.) ;
#43749=ORIENTED_EDGE('',*,*,#30211,.T.) ;
#43750=ORIENTED_EDGE('',*,*,#30212,.T.) ;
#43751=ORIENTED_EDGE('',*,*,#30211,.F.) ;
#43752=ORIENTED_EDGE('',*,*,#30075,.T.) ;
#43753=ORIENTED_EDGE('',*,*,#30213,.T.) ;
#43754=ORIENTED_EDGE('',*,*,#30214,.T.) ;
#43755=ORIENTED_EDGE('',*,*,#30213,.F.) ;
#43756=ORIENTED_EDGE('',*,*,#30074,.T.) ;
#43757=ORIENTED_EDGE('',*,*,#30162,.F.) ;
#43758=ORIENTED_EDGE('',*,*,#30107,.T.) ;
#43759=ORIENTED_EDGE('',*,*,#30165,.F.) ;
#43760=ORIENTED_EDGE('',*,*,#29960,.T.) ;
#43761=ORIENTED_EDGE('',*,*,#30160,.F.) ;
#43762=ORIENTED_EDGE('',*,*,#30215,.T.) ;
#43763=ORIENTED_EDGE('',*,*,#30163,.F.) ;
#43764=ORIENTED_EDGE('',*,*,#30049,.T.) ;
#43765=ORIENTED_EDGE('',*,*,#30216,.T.) ;
#43766=ORIENTED_EDGE('',*,*,#30217,.T.) ;
#43767=ORIENTED_EDGE('',*,*,#30216,.F.) ;
#43768=ORIENTED_EDGE('',*,*,#30078,.T.) ;
#43769=ORIENTED_EDGE('',*,*,#30218,.T.) ;
#43770=ORIENTED_EDGE('',*,*,#30219,.T.) ;
#43771=ORIENTED_EDGE('',*,*,#30218,.F.) ;
#43772=ORIENTED_EDGE('',*,*,#30077,.T.) ;
#43773=ORIENTED_EDGE('',*,*,#30155,.F.) ;
#43774=ORIENTED_EDGE('',*,*,#30104,.T.) ;
#43775=ORIENTED_EDGE('',*,*,#30158,.F.) ;
#43776=ORIENTED_EDGE('',*,*,#29968,.T.) ;
#43777=ORIENTED_EDGE('',*,*,#30153,.F.) ;
#43778=ORIENTED_EDGE('',*,*,#30220,.T.) ;
#43779=ORIENTED_EDGE('',*,*,#30156,.F.) ;
#43780=ORIENTED_EDGE('',*,*,#30047,.T.) ;
#43781=ORIENTED_EDGE('',*,*,#30221,.T.) ;
#43782=ORIENTED_EDGE('',*,*,#30222,.T.) ;
#43783=ORIENTED_EDGE('',*,*,#30221,.F.) ;
#43784=ORIENTED_EDGE('',*,*,#30081,.T.) ;
#43785=ORIENTED_EDGE('',*,*,#30223,.T.) ;
#43786=ORIENTED_EDGE('',*,*,#30224,.T.) ;
#43787=ORIENTED_EDGE('',*,*,#30223,.F.) ;
#43788=ORIENTED_EDGE('',*,*,#30080,.T.) ;
#43789=ORIENTED_EDGE('',*,*,#30148,.F.) ;
#43790=ORIENTED_EDGE('',*,*,#30101,.T.) ;
#43791=ORIENTED_EDGE('',*,*,#30151,.F.) ;
#43792=ORIENTED_EDGE('',*,*,#29976,.T.) ;
#43793=ORIENTED_EDGE('',*,*,#30146,.F.) ;
#43794=ORIENTED_EDGE('',*,*,#30225,.T.) ;
#43795=ORIENTED_EDGE('',*,*,#30149,.F.) ;
#43796=ORIENTED_EDGE('',*,*,#30045,.T.) ;
#43797=ORIENTED_EDGE('',*,*,#30226,.T.) ;
#43798=ORIENTED_EDGE('',*,*,#30227,.T.) ;
#43799=ORIENTED_EDGE('',*,*,#30226,.F.) ;
#43800=ORIENTED_EDGE('',*,*,#30084,.T.) ;
#43801=ORIENTED_EDGE('',*,*,#30228,.T.) ;
#43802=ORIENTED_EDGE('',*,*,#30229,.T.) ;
#43803=ORIENTED_EDGE('',*,*,#30228,.F.) ;
#43804=ORIENTED_EDGE('',*,*,#30083,.T.) ;
#43805=ORIENTED_EDGE('',*,*,#30141,.F.) ;
#43806=ORIENTED_EDGE('',*,*,#30098,.T.) ;
#43807=ORIENTED_EDGE('',*,*,#30144,.F.) ;
#43808=ORIENTED_EDGE('',*,*,#29984,.T.) ;
#43809=ORIENTED_EDGE('',*,*,#30139,.F.) ;
#43810=ORIENTED_EDGE('',*,*,#30230,.T.) ;
#43811=ORIENTED_EDGE('',*,*,#30142,.F.) ;
#43812=ORIENTED_EDGE('',*,*,#30043,.T.) ;
#43813=ORIENTED_EDGE('',*,*,#30231,.T.) ;
#43814=ORIENTED_EDGE('',*,*,#30232,.T.) ;
#43815=ORIENTED_EDGE('',*,*,#30231,.F.) ;
#43816=ORIENTED_EDGE('',*,*,#30087,.T.) ;
#43817=ORIENTED_EDGE('',*,*,#30233,.T.) ;
#43818=ORIENTED_EDGE('',*,*,#30234,.T.) ;
#43819=ORIENTED_EDGE('',*,*,#30233,.F.) ;
#43820=ORIENTED_EDGE('',*,*,#30086,.T.) ;
#43821=ORIENTED_EDGE('',*,*,#30134,.F.) ;
#43822=ORIENTED_EDGE('',*,*,#30095,.T.) ;
#43823=ORIENTED_EDGE('',*,*,#30137,.F.) ;
#43824=ORIENTED_EDGE('',*,*,#29992,.T.) ;
#43825=ORIENTED_EDGE('',*,*,#30132,.F.) ;
#43826=ORIENTED_EDGE('',*,*,#30235,.T.) ;
#43827=ORIENTED_EDGE('',*,*,#30135,.F.) ;
#43828=ORIENTED_EDGE('',*,*,#30041,.T.) ;
#43829=ORIENTED_EDGE('',*,*,#30236,.T.) ;
#43830=ORIENTED_EDGE('',*,*,#30237,.T.) ;
#43831=ORIENTED_EDGE('',*,*,#30236,.F.) ;
#43832=ORIENTED_EDGE('',*,*,#30090,.T.) ;
#43833=ORIENTED_EDGE('',*,*,#30238,.T.) ;
#43834=ORIENTED_EDGE('',*,*,#30239,.T.) ;
#43835=ORIENTED_EDGE('',*,*,#30238,.F.) ;
#43836=ORIENTED_EDGE('',*,*,#30089,.T.) ;
#43837=ORIENTED_EDGE('',*,*,#30127,.F.) ;
#43838=ORIENTED_EDGE('',*,*,#30092,.T.) ;
#43839=ORIENTED_EDGE('',*,*,#30130,.F.) ;
#43840=ORIENTED_EDGE('',*,*,#30240,.T.) ;
#43841=ORIENTED_EDGE('',*,*,#30124,.F.) ;
#43842=ORIENTED_EDGE('',*,*,#29691,.F.) ;
#43843=ORIENTED_EDGE('',*,*,#30241,.T.) ;
#43844=ORIENTED_EDGE('',*,*,#30122,.F.) ;
#43845=ORIENTED_EDGE('',*,*,#30242,.T.) ;
#43846=ORIENTED_EDGE('',*,*,#29688,.F.) ;
#43847=ORIENTED_EDGE('',*,*,#30242,.F.) ;
#43848=ORIENTED_EDGE('',*,*,#30125,.F.) ;
#43849=ORIENTED_EDGE('',*,*,#30243,.T.) ;
#43850=ORIENTED_EDGE('',*,*,#29685,.F.) ;
#43851=ORIENTED_EDGE('',*,*,#30243,.F.) ;
#43852=ORIENTED_EDGE('',*,*,#30240,.F.) ;
#43853=ORIENTED_EDGE('',*,*,#30244,.T.) ;
#43854=ORIENTED_EDGE('',*,*,#29682,.F.) ;
#43855=ORIENTED_EDGE('',*,*,#30244,.F.) ;
#43856=ORIENTED_EDGE('',*,*,#30129,.F.) ;
#43857=ORIENTED_EDGE('',*,*,#29995,.F.) ;
#43858=ORIENTED_EDGE('',*,*,#29796,.F.) ;
#43859=ORIENTED_EDGE('',*,*,#30245,.F.) ;
#43860=ORIENTED_EDGE('',*,*,#30197,.F.) ;
#43861=ORIENTED_EDGE('',*,*,#30246,.T.) ;
#43862=ORIENTED_EDGE('',*,*,#29790,.F.) ;
#43863=ORIENTED_EDGE('',*,*,#30247,.F.) ;
#43864=ORIENTED_EDGE('',*,*,#30182,.F.) ;
#43865=ORIENTED_EDGE('',*,*,#30248,.F.) ;
#43866=ORIENTED_EDGE('',*,*,#29793,.F.) ;
#43867=ORIENTED_EDGE('',*,*,#30246,.F.) ;
#43868=ORIENTED_EDGE('',*,*,#30199,.F.) ;
#43869=ORIENTED_EDGE('',*,*,#30247,.T.) ;
#43870=ORIENTED_EDGE('',*,*,#29784,.F.) ;
#43871=ORIENTED_EDGE('',*,*,#30249,.F.) ;
#43872=ORIENTED_EDGE('',*,*,#30202,.F.) ;
#43873=ORIENTED_EDGE('',*,*,#30250,.T.) ;
#43874=ORIENTED_EDGE('',*,*,#29778,.F.) ;
#43875=ORIENTED_EDGE('',*,*,#30251,.F.) ;
#43876=ORIENTED_EDGE('',*,*,#30175,.F.) ;
#43877=ORIENTED_EDGE('',*,*,#30252,.F.) ;
#43878=ORIENTED_EDGE('',*,*,#29781,.F.) ;
#43879=ORIENTED_EDGE('',*,*,#30250,.F.) ;
#43880=ORIENTED_EDGE('',*,*,#30204,.F.) ;
#43881=ORIENTED_EDGE('',*,*,#30251,.T.) ;
#43882=ORIENTED_EDGE('',*,*,#29772,.F.) ;
#43883=ORIENTED_EDGE('',*,*,#30253,.F.) ;
#43884=ORIENTED_EDGE('',*,*,#30207,.F.) ;
#43885=ORIENTED_EDGE('',*,*,#30254,.T.) ;
#43886=ORIENTED_EDGE('',*,*,#29766,.F.) ;
#43887=ORIENTED_EDGE('',*,*,#30255,.F.) ;
#43888=ORIENTED_EDGE('',*,*,#30168,.F.) ;
#43889=ORIENTED_EDGE('',*,*,#30256,.F.) ;
#43890=ORIENTED_EDGE('',*,*,#29769,.F.) ;
#43891=ORIENTED_EDGE('',*,*,#30254,.F.) ;
#43892=ORIENTED_EDGE('',*,*,#30209,.F.) ;
#43893=ORIENTED_EDGE('',*,*,#30255,.T.) ;
#43894=ORIENTED_EDGE('',*,*,#29760,.F.) ;
#43895=ORIENTED_EDGE('',*,*,#30257,.F.) ;
#43896=ORIENTED_EDGE('',*,*,#30212,.F.) ;
#43897=ORIENTED_EDGE('',*,*,#30258,.T.) ;
#43898=ORIENTED_EDGE('',*,*,#29754,.F.) ;
#43899=ORIENTED_EDGE('',*,*,#30259,.F.) ;
#43900=ORIENTED_EDGE('',*,*,#30161,.F.) ;
#43901=ORIENTED_EDGE('',*,*,#30260,.F.) ;
#43902=ORIENTED_EDGE('',*,*,#29757,.F.) ;
#43903=ORIENTED_EDGE('',*,*,#30258,.F.) ;
#43904=ORIENTED_EDGE('',*,*,#30214,.F.) ;
#43905=ORIENTED_EDGE('',*,*,#30259,.T.) ;
#43906=ORIENTED_EDGE('',*,*,#29748,.F.) ;
#43907=ORIENTED_EDGE('',*,*,#30261,.F.) ;
#43908=ORIENTED_EDGE('',*,*,#30217,.F.) ;
#43909=ORIENTED_EDGE('',*,*,#30262,.T.) ;
#43910=ORIENTED_EDGE('',*,*,#29742,.F.) ;
#43911=ORIENTED_EDGE('',*,*,#30263,.F.) ;
#43912=ORIENTED_EDGE('',*,*,#30154,.F.) ;
#43913=ORIENTED_EDGE('',*,*,#30264,.F.) ;
#43914=ORIENTED_EDGE('',*,*,#29745,.F.) ;
#43915=ORIENTED_EDGE('',*,*,#30262,.F.) ;
#43916=ORIENTED_EDGE('',*,*,#30219,.F.) ;
#43917=ORIENTED_EDGE('',*,*,#30263,.T.) ;
#43918=ORIENTED_EDGE('',*,*,#29736,.F.) ;
#43919=ORIENTED_EDGE('',*,*,#30265,.F.) ;
#43920=ORIENTED_EDGE('',*,*,#30222,.F.) ;
#43921=ORIENTED_EDGE('',*,*,#30266,.T.) ;
#43922=ORIENTED_EDGE('',*,*,#29730,.F.) ;
#43923=ORIENTED_EDGE('',*,*,#30267,.F.) ;
#43924=ORIENTED_EDGE('',*,*,#30147,.F.) ;
#43925=ORIENTED_EDGE('',*,*,#30268,.F.) ;
#43926=ORIENTED_EDGE('',*,*,#29733,.F.) ;
#43927=ORIENTED_EDGE('',*,*,#30266,.F.) ;
#43928=ORIENTED_EDGE('',*,*,#30224,.F.) ;
#43929=ORIENTED_EDGE('',*,*,#30267,.T.) ;
#43930=ORIENTED_EDGE('',*,*,#29724,.F.) ;
#43931=ORIENTED_EDGE('',*,*,#30269,.F.) ;
#43932=ORIENTED_EDGE('',*,*,#30227,.F.) ;
#43933=ORIENTED_EDGE('',*,*,#30270,.T.) ;
#43934=ORIENTED_EDGE('',*,*,#29718,.F.) ;
#43935=ORIENTED_EDGE('',*,*,#30271,.F.) ;
#43936=ORIENTED_EDGE('',*,*,#30140,.F.) ;
#43937=ORIENTED_EDGE('',*,*,#30272,.F.) ;
#43938=ORIENTED_EDGE('',*,*,#29721,.F.) ;
#43939=ORIENTED_EDGE('',*,*,#30270,.F.) ;
#43940=ORIENTED_EDGE('',*,*,#30229,.F.) ;
#43941=ORIENTED_EDGE('',*,*,#30271,.T.) ;
#43942=ORIENTED_EDGE('',*,*,#29712,.F.) ;
#43943=ORIENTED_EDGE('',*,*,#30273,.F.) ;
#43944=ORIENTED_EDGE('',*,*,#30232,.F.) ;
#43945=ORIENTED_EDGE('',*,*,#30274,.T.) ;
#43946=ORIENTED_EDGE('',*,*,#29706,.F.) ;
#43947=ORIENTED_EDGE('',*,*,#30275,.F.) ;
#43948=ORIENTED_EDGE('',*,*,#30133,.F.) ;
#43949=ORIENTED_EDGE('',*,*,#30276,.F.) ;
#43950=ORIENTED_EDGE('',*,*,#29709,.F.) ;
#43951=ORIENTED_EDGE('',*,*,#30274,.F.) ;
#43952=ORIENTED_EDGE('',*,*,#30234,.F.) ;
#43953=ORIENTED_EDGE('',*,*,#30275,.T.) ;
#43954=ORIENTED_EDGE('',*,*,#29700,.F.) ;
#43955=ORIENTED_EDGE('',*,*,#30277,.F.) ;
#43956=ORIENTED_EDGE('',*,*,#30237,.F.) ;
#43957=ORIENTED_EDGE('',*,*,#30278,.T.) ;
#43958=ORIENTED_EDGE('',*,*,#29694,.F.) ;
#43959=ORIENTED_EDGE('',*,*,#30279,.F.) ;
#43960=ORIENTED_EDGE('',*,*,#30126,.F.) ;
#43961=ORIENTED_EDGE('',*,*,#30241,.F.) ;
#43962=ORIENTED_EDGE('',*,*,#29697,.F.) ;
#43963=ORIENTED_EDGE('',*,*,#30278,.F.) ;
#43964=ORIENTED_EDGE('',*,*,#30239,.F.) ;
#43965=ORIENTED_EDGE('',*,*,#30279,.T.) ;
#43966=ORIENTED_EDGE('',*,*,#29703,.F.) ;
#43967=ORIENTED_EDGE('',*,*,#30276,.T.) ;
#43968=ORIENTED_EDGE('',*,*,#30235,.F.) ;
#43969=ORIENTED_EDGE('',*,*,#30277,.T.) ;
#43970=ORIENTED_EDGE('',*,*,#29715,.F.) ;
#43971=ORIENTED_EDGE('',*,*,#30272,.T.) ;
#43972=ORIENTED_EDGE('',*,*,#30230,.F.) ;
#43973=ORIENTED_EDGE('',*,*,#30273,.T.) ;
#43974=ORIENTED_EDGE('',*,*,#29727,.F.) ;
#43975=ORIENTED_EDGE('',*,*,#30268,.T.) ;
#43976=ORIENTED_EDGE('',*,*,#30225,.F.) ;
#43977=ORIENTED_EDGE('',*,*,#30269,.T.) ;
#43978=ORIENTED_EDGE('',*,*,#29739,.F.) ;
#43979=ORIENTED_EDGE('',*,*,#30264,.T.) ;
#43980=ORIENTED_EDGE('',*,*,#30220,.F.) ;
#43981=ORIENTED_EDGE('',*,*,#30265,.T.) ;
#43982=ORIENTED_EDGE('',*,*,#29751,.F.) ;
#43983=ORIENTED_EDGE('',*,*,#30260,.T.) ;
#43984=ORIENTED_EDGE('',*,*,#30215,.F.) ;
#43985=ORIENTED_EDGE('',*,*,#30261,.T.) ;
#43986=ORIENTED_EDGE('',*,*,#29763,.F.) ;
#43987=ORIENTED_EDGE('',*,*,#30256,.T.) ;
#43988=ORIENTED_EDGE('',*,*,#30210,.F.) ;
#43989=ORIENTED_EDGE('',*,*,#30257,.T.) ;
#43990=ORIENTED_EDGE('',*,*,#29775,.F.) ;
#43991=ORIENTED_EDGE('',*,*,#30252,.T.) ;
#43992=ORIENTED_EDGE('',*,*,#30205,.F.) ;
#43993=ORIENTED_EDGE('',*,*,#30253,.T.) ;
#43994=ORIENTED_EDGE('',*,*,#29787,.F.) ;
#43995=ORIENTED_EDGE('',*,*,#30248,.T.) ;
#43996=ORIENTED_EDGE('',*,*,#30200,.F.) ;
#43997=ORIENTED_EDGE('',*,*,#30249,.T.) ;
#43998=ORIENTED_EDGE('',*,*,#29799,.F.) ;
#43999=ORIENTED_EDGE('',*,*,#29918,.T.) ;
#44000=ORIENTED_EDGE('',*,*,#30195,.F.) ;
#44001=ORIENTED_EDGE('',*,*,#30245,.T.) ;
#44002=ORIENTED_EDGE('',*,*,#29668,.F.) ;
#44003=ORIENTED_EDGE('',*,*,#30280,.T.) ;
#44004=ORIENTED_EDGE('',*,*,#29669,.F.) ;
#44005=ORIENTED_EDGE('',*,*,#30280,.F.) ;
#45797=TOROIDAL_SURFACE('',#54043,3.96824583655185,1.) ;
#45798=TOROIDAL_SURFACE('',#54048,4.,1.) ;
#45799=TOROIDAL_SURFACE('',#54057,4.95,0.15) ;
#45800=TOROIDAL_SURFACE('',#54061,0.350000000000003,0.15) ;
#45801=TOROIDAL_SURFACE('',#54065,4.95,0.15) ;
#45802=TOROIDAL_SURFACE('',#54069,0.350000000000003,0.15) ;
#45803=TOROIDAL_SURFACE('',#54073,4.95,0.15) ;
#45804=TOROIDAL_SURFACE('',#54077,0.350000000000003,0.15) ;
#45805=TOROIDAL_SURFACE('',#54081,4.95,0.15) ;
#45806=TOROIDAL_SURFACE('',#54085,0.350000000000003,0.15) ;
#45807=TOROIDAL_SURFACE('',#54089,4.95,0.15) ;
#45808=TOROIDAL_SURFACE('',#54093,0.350000000000003,0.15) ;
#45809=TOROIDAL_SURFACE('',#54097,4.95,0.15) ;
#45810=TOROIDAL_SURFACE('',#54101,0.350000000000003,0.15) ;
#45811=TOROIDAL_SURFACE('',#54105,4.95,0.15) ;
#45812=TOROIDAL_SURFACE('',#54109,0.350000000000003,0.15) ;
#45813=TOROIDAL_SURFACE('',#54113,4.95,0.15) ;
#45814=TOROIDAL_SURFACE('',#54117,0.350000000000003,0.15) ;
#45815=TOROIDAL_SURFACE('',#54121,4.95,0.15) ;
#45816=TOROIDAL_SURFACE('',#54125,0.350000000000003,0.15) ;
#45817=TOROIDAL_SURFACE('',#54129,4.95,0.15) ;
#45818=TOROIDAL_SURFACE('',#54133,0.350000000000003,0.15) ;
#45819=TOROIDAL_SURFACE('',#54137,4.95,0.15) ;
#45820=TOROIDAL_SURFACE('',#54141,0.350000000000003,0.15) ;
#45821=TOROIDAL_SURFACE('',#54145,4.95,0.15) ;
#45822=TOROIDAL_SURFACE('',#54149,0.350000000000003,0.15) ;
#45823=TOROIDAL_SURFACE('',#54153,4.95,0.15) ;
#45824=TOROIDAL_SURFACE('',#54157,0.350000000000003,0.15) ;
#45825=TOROIDAL_SURFACE('',#54161,4.95,0.15) ;
#45826=TOROIDAL_SURFACE('',#54165,0.350000000000003,0.15) ;
#45827=TOROIDAL_SURFACE('',#54169,4.95,0.15) ;
#45828=TOROIDAL_SURFACE('',#54173,0.350000000000003,0.15) ;
#45829=TOROIDAL_SURFACE('',#54177,4.95,0.15) ;
#45830=TOROIDAL_SURFACE('',#54181,0.350000000000003,0.15) ;
#45831=TOROIDAL_SURFACE('',#54185,4.95,0.15) ;
#45832=TOROIDAL_SURFACE('',#54189,0.350000000000003,0.15) ;
#45833=TOROIDAL_SURFACE('',#54193,4.95,0.15) ;
#45834=TOROIDAL_SURFACE('',#54197,0.350000000000003,0.15) ;
#45835=TOROIDAL_SURFACE('',#54201,4.95,0.15) ;
#45836=TOROIDAL_SURFACE('',#54205,0.350000000000003,0.15) ;
#45837=TOROIDAL_SURFACE('',#54209,4.95,0.15) ;
#45838=TOROIDAL_SURFACE('',#54213,0.350000000000003,0.15) ;
#45839=TOROIDAL_SURFACE('',#54316,4.95,0.15) ;
#45840=TOROIDAL_SURFACE('',#54320,4.95,0.15) ;
#45841=TOROIDAL_SURFACE('',#54403,4.95,0.15) ;
#45842=TOROIDAL_SURFACE('',#54408,4.95,0.15) ;
#45843=TOROIDAL_SURFACE('',#54412,4.95,0.15) ;
#45844=TOROIDAL_SURFACE('',#54416,4.95,0.15) ;
#45845=TOROIDAL_SURFACE('',#54420,4.95,0.15) ;
#45846=TOROIDAL_SURFACE('',#54424,4.95,0.15) ;
#45847=TOROIDAL_SURFACE('',#54428,4.95,0.15) ;
#45848=TOROIDAL_SURFACE('',#54432,4.95,0.15) ;
#45849=TOROIDAL_SURFACE('',#54436,4.95,0.15) ;
#45850=TOROIDAL_SURFACE('',#54440,4.95,0.15) ;
#45851=TOROIDAL_SURFACE('',#54444,4.95,0.15) ;
#45852=TOROIDAL_SURFACE('',#54446,0.350000000000003,0.15) ;
#45853=TOROIDAL_SURFACE('',#54447,0.350000000000003,0.15) ;
#45854=TOROIDAL_SURFACE('',#54448,4.95,0.15) ;
#45855=TOROIDAL_SURFACE('',#54451,0.350000000000003,0.15) ;
#45856=TOROIDAL_SURFACE('',#54453,0.350000000000003,0.15) ;
#45857=TOROIDAL_SURFACE('',#54454,4.95,0.15) ;
#45858=TOROIDAL_SURFACE('',#54457,0.350000000000003,0.15) ;
#45859=TOROIDAL_SURFACE('',#54459,0.350000000000003,0.15) ;
#45860=TOROIDAL_SURFACE('',#54460,4.95,0.15) ;
#45861=TOROIDAL_SURFACE('',#54463,0.350000000000003,0.15) ;
#45862=TOROIDAL_SURFACE('',#54465,0.350000000000003,0.15) ;
#45863=TOROIDAL_SURFACE('',#54466,4.95,0.15) ;
#45864=TOROIDAL_SURFACE('',#54469,0.350000000000003,0.15) ;
#45865=TOROIDAL_SURFACE('',#54471,0.350000000000003,0.15) ;
#45866=TOROIDAL_SURFACE('',#54472,4.95,0.15) ;
#45867=TOROIDAL_SURFACE('',#54475,0.350000000000003,0.15) ;
#45868=TOROIDAL_SURFACE('',#54477,0.350000000000003,0.15) ;
#45869=TOROIDAL_SURFACE('',#54478,4.95,0.15) ;
#45870=TOROIDAL_SURFACE('',#54481,0.350000000000003,0.15) ;
#45871=TOROIDAL_SURFACE('',#54483,0.350000000000003,0.15) ;
#45872=TOROIDAL_SURFACE('',#54484,4.95,0.15) ;
#45873=TOROIDAL_SURFACE('',#54487,0.350000000000003,0.15) ;
#45874=TOROIDAL_SURFACE('',#54489,0.350000000000003,0.15) ;
#45875=TOROIDAL_SURFACE('',#54490,4.95,0.15) ;
#45876=TOROIDAL_SURFACE('',#54493,0.350000000000003,0.15) ;
#45877=TOROIDAL_SURFACE('',#54495,0.350000000000003,0.15) ;
#45878=TOROIDAL_SURFACE('',#54496,4.95,0.15) ;
#45879=TOROIDAL_SURFACE('',#54499,0.350000000000003,0.15) ;
#45880=TOROIDAL_SURFACE('',#54501,0.350000000000003,0.15) ;
#48452=ADVANCED_FACE('',(#13234),#45797,.F.) ;
#48453=ADVANCED_FACE('',(#13235,#762),#2858,.F.) ;
#48454=ADVANCED_FACE('',(#13236),#45798,.F.) ;
#48455=ADVANCED_FACE('',(#13237,#763),#2859,.T.) ;
#48456=ADVANCED_FACE('',(#13238,#764),#2860,.T.) ;
#48457=ADVANCED_FACE('',(#13239,#765),#2861,.F.) ;
#48458=ADVANCED_FACE('',(#13240),#2111,.F.) ;
#48459=ADVANCED_FACE('',(#13241),#2112,.F.) ;
#48460=ADVANCED_FACE('',(#13242),#45799,.T.) ;
#48461=ADVANCED_FACE('',(#13243),#10492,.T.) ;
#48462=ADVANCED_FACE('',(#13244),#45800,.T.) ;
#48463=ADVANCED_FACE('',(#13245),#10493,.T.) ;
#48464=ADVANCED_FACE('',(#13246),#45801,.T.) ;
#48465=ADVANCED_FACE('',(#13247),#10494,.T.) ;
#48466=ADVANCED_FACE('',(#13248),#45802,.T.) ;
#48467=ADVANCED_FACE('',(#13249),#10495,.T.) ;
#48468=ADVANCED_FACE('',(#13250),#45803,.T.) ;
#48469=ADVANCED_FACE('',(#13251),#10496,.T.) ;
#48470=ADVANCED_FACE('',(#13252),#45804,.T.) ;
#48471=ADVANCED_FACE('',(#13253),#10497,.T.) ;
#48472=ADVANCED_FACE('',(#13254),#45805,.T.) ;
#48473=ADVANCED_FACE('',(#13255),#10498,.T.) ;
#48474=ADVANCED_FACE('',(#13256),#45806,.T.) ;
#48475=ADVANCED_FACE('',(#13257),#10499,.T.) ;
#48476=ADVANCED_FACE('',(#13258),#45807,.T.) ;
#48477=ADVANCED_FACE('',(#13259),#10500,.T.) ;
#48478=ADVANCED_FACE('',(#13260),#45808,.T.) ;
#48479=ADVANCED_FACE('',(#13261),#10501,.T.) ;
#48480=ADVANCED_FACE('',(#13262),#45809,.T.) ;
#48481=ADVANCED_FACE('',(#13263),#10502,.T.) ;
#48482=ADVANCED_FACE('',(#13264),#45810,.T.) ;
#48483=ADVANCED_FACE('',(#13265),#10503,.T.) ;
#48484=ADVANCED_FACE('',(#13266),#45811,.T.) ;
#48485=ADVANCED_FACE('',(#13267),#10504,.T.) ;
#48486=ADVANCED_FACE('',(#13268),#45812,.T.) ;
#48487=ADVANCED_FACE('',(#13269),#10505,.T.) ;
#48488=ADVANCED_FACE('',(#13270),#45813,.T.) ;
#48489=ADVANCED_FACE('',(#13271),#10506,.T.) ;
#48490=ADVANCED_FACE('',(#13272),#45814,.T.) ;
#48491=ADVANCED_FACE('',(#13273),#10507,.T.) ;
#48492=ADVANCED_FACE('',(#13274),#45815,.T.) ;
#48493=ADVANCED_FACE('',(#13275),#10508,.T.) ;
#48494=ADVANCED_FACE('',(#13276),#45816,.T.) ;
#48495=ADVANCED_FACE('',(#13277),#10509,.T.) ;
#48496=ADVANCED_FACE('',(#13278),#45817,.T.) ;
#48497=ADVANCED_FACE('',(#13279),#10510,.T.) ;
#48498=ADVANCED_FACE('',(#13280),#45818,.T.) ;
#48499=ADVANCED_FACE('',(#13281),#10511,.T.) ;
#48500=ADVANCED_FACE('',(#13282),#45819,.T.) ;
#48501=ADVANCED_FACE('',(#13283),#10512,.T.) ;
#48502=ADVANCED_FACE('',(#13284),#45820,.T.) ;
#48503=ADVANCED_FACE('',(#13285),#10513,.T.) ;
#48504=ADVANCED_FACE('',(#13286),#45821,.T.) ;
#48505=ADVANCED_FACE('',(#13287),#10514,.T.) ;
#48506=ADVANCED_FACE('',(#13288),#45822,.T.) ;
#48507=ADVANCED_FACE('',(#13289),#10515,.T.) ;
#48508=ADVANCED_FACE('',(#13290),#45823,.T.) ;
#48509=ADVANCED_FACE('',(#13291),#10516,.T.) ;
#48510=ADVANCED_FACE('',(#13292),#45824,.T.) ;
#48511=ADVANCED_FACE('',(#13293),#10517,.T.) ;
#48512=ADVANCED_FACE('',(#13294),#45825,.T.) ;
#48513=ADVANCED_FACE('',(#13295),#10518,.T.) ;
#48514=ADVANCED_FACE('',(#13296),#45826,.T.) ;
#48515=ADVANCED_FACE('',(#13297),#10519,.T.) ;
#48516=ADVANCED_FACE('',(#13298),#45827,.T.) ;
#48517=ADVANCED_FACE('',(#13299),#10520,.T.) ;
#48518=ADVANCED_FACE('',(#13300),#45828,.T.) ;
#48519=ADVANCED_FACE('',(#13301),#10521,.T.) ;
#48520=ADVANCED_FACE('',(#13302),#45829,.T.) ;
#48521=ADVANCED_FACE('',(#13303),#10522,.T.) ;
#48522=ADVANCED_FACE('',(#13304),#45830,.T.) ;
#48523=ADVANCED_FACE('',(#13305),#10523,.T.) ;
#48524=ADVANCED_FACE('',(#13306),#45831,.T.) ;
#48525=ADVANCED_FACE('',(#13307),#10524,.T.) ;
#48526=ADVANCED_FACE('',(#13308),#45832,.T.) ;
#48527=ADVANCED_FACE('',(#13309),#10525,.T.) ;
#48528=ADVANCED_FACE('',(#13310),#45833,.T.) ;
#48529=ADVANCED_FACE('',(#13311),#10526,.T.) ;
#48530=ADVANCED_FACE('',(#13312),#45834,.T.) ;
#48531=ADVANCED_FACE('',(#13313),#10527,.T.) ;
#48532=ADVANCED_FACE('',(#13314),#45835,.T.) ;
#48533=ADVANCED_FACE('',(#13315),#10528,.T.) ;
#48534=ADVANCED_FACE('',(#13316),#45836,.T.) ;
#48535=ADVANCED_FACE('',(#13317),#10529,.T.) ;
#48536=ADVANCED_FACE('',(#13318),#45837,.T.) ;
#48537=ADVANCED_FACE('',(#13319),#10530,.T.) ;
#48538=ADVANCED_FACE('',(#13320),#45838,.T.) ;
#48539=ADVANCED_FACE('',(#13321),#10531,.T.) ;
#48540=ADVANCED_FACE('',(#13322),#2862,.T.) ;
#48541=ADVANCED_FACE('',(#13323),#10532,.T.) ;
#48542=ADVANCED_FACE('',(#13324),#2863,.T.) ;
#48543=ADVANCED_FACE('',(#13325),#10533,.T.) ;
#48544=ADVANCED_FACE('',(#13326),#2864,.T.) ;
#48545=ADVANCED_FACE('',(#13327),#10534,.T.) ;
#48546=ADVANCED_FACE('',(#13328),#2865,.T.) ;
#48547=ADVANCED_FACE('',(#13329),#10535,.T.) ;
#48548=ADVANCED_FACE('',(#13330),#2866,.T.) ;
#48549=ADVANCED_FACE('',(#13331),#10536,.T.) ;
#48550=ADVANCED_FACE('',(#13332),#2867,.T.) ;
#48551=ADVANCED_FACE('',(#13333),#10537,.T.) ;
#48552=ADVANCED_FACE('',(#13334),#2868,.T.) ;
#48553=ADVANCED_FACE('',(#13335),#10538,.T.) ;
#48554=ADVANCED_FACE('',(#13336),#2869,.T.) ;
#48555=ADVANCED_FACE('',(#13337),#10539,.T.) ;
#48556=ADVANCED_FACE('',(#13338),#2870,.T.) ;
#48557=ADVANCED_FACE('',(#13339),#10540,.T.) ;
#48558=ADVANCED_FACE('',(#13340),#2871,.T.) ;
#48559=ADVANCED_FACE('',(#13341),#10541,.T.) ;
#48560=ADVANCED_FACE('',(#13342),#2872,.T.) ;
#48561=ADVANCED_FACE('',(#13343),#10542,.T.) ;
#48562=ADVANCED_FACE('',(#13344),#2873,.T.) ;
#48563=ADVANCED_FACE('',(#13345),#10543,.T.) ;
#48564=ADVANCED_FACE('',(#13346),#2874,.T.) ;
#48565=ADVANCED_FACE('',(#13347),#10544,.T.) ;
#48566=ADVANCED_FACE('',(#13348),#2875,.T.) ;
#48567=ADVANCED_FACE('',(#13349),#10545,.T.) ;
#48568=ADVANCED_FACE('',(#13350),#2876,.T.) ;
#48569=ADVANCED_FACE('',(#13351),#10546,.T.) ;
#48570=ADVANCED_FACE('',(#13352),#2877,.T.) ;
#48571=ADVANCED_FACE('',(#13353),#10547,.T.) ;
#48572=ADVANCED_FACE('',(#13354),#2878,.T.) ;
#48573=ADVANCED_FACE('',(#13355),#10548,.T.) ;
#48574=ADVANCED_FACE('',(#13356),#2879,.T.) ;
#48575=ADVANCED_FACE('',(#13357),#10549,.T.) ;
#48576=ADVANCED_FACE('',(#13358),#2880,.T.) ;
#48577=ADVANCED_FACE('',(#13359),#10550,.T.) ;
#48578=ADVANCED_FACE('',(#13360),#2881,.T.) ;
#48579=ADVANCED_FACE('',(#13361),#10551,.T.) ;
#48580=ADVANCED_FACE('',(#13362),#2882,.F.) ;
#48581=ADVANCED_FACE('',(#13363),#2883,.F.) ;
#48582=ADVANCED_FACE('',(#13364),#2884,.F.) ;
#48583=ADVANCED_FACE('',(#13365),#2885,.F.) ;
#48584=ADVANCED_FACE('',(#13366),#2886,.F.) ;
#48585=ADVANCED_FACE('',(#13367),#2887,.F.) ;
#48586=ADVANCED_FACE('',(#13368),#2888,.F.) ;
#48587=ADVANCED_FACE('',(#13369),#2889,.F.) ;
#48588=ADVANCED_FACE('',(#13370),#2890,.F.) ;
#48589=ADVANCED_FACE('',(#13371),#2891,.F.) ;
#48590=ADVANCED_FACE('',(#13372),#2892,.F.) ;
#48591=ADVANCED_FACE('',(#13373),#2893,.F.) ;
#48592=ADVANCED_FACE('',(#13374),#2894,.F.) ;
#48593=ADVANCED_FACE('',(#13375),#2895,.F.) ;
#48594=ADVANCED_FACE('',(#13376),#2896,.F.) ;
#48595=ADVANCED_FACE('',(#13377),#2897,.F.) ;
#48596=ADVANCED_FACE('',(#13378),#2898,.F.) ;
#48597=ADVANCED_FACE('',(#13379),#2899,.F.) ;
#48598=ADVANCED_FACE('',(#13380),#2900,.F.) ;
#48599=ADVANCED_FACE('',(#13381),#45839,.F.) ;
#48600=ADVANCED_FACE('',(#13382),#2901,.F.) ;
#48601=ADVANCED_FACE('',(#13383),#45840,.F.) ;
#48602=ADVANCED_FACE('',(#13384),#2902,.T.) ;
#48603=ADVANCED_FACE('',(#13385),#2903,.T.) ;
#48604=ADVANCED_FACE('',(#13386),#2904,.T.) ;
#48605=ADVANCED_FACE('',(#13387),#2905,.T.) ;
#48606=ADVANCED_FACE('',(#13388),#2906,.T.) ;
#48607=ADVANCED_FACE('',(#13389),#2907,.T.) ;
#48608=ADVANCED_FACE('',(#13390),#2908,.T.) ;
#48609=ADVANCED_FACE('',(#13391),#2909,.T.) ;
#48610=ADVANCED_FACE('',(#13392),#2910,.T.) ;
#48611=ADVANCED_FACE('',(#13393),#2911,.T.) ;
#48612=ADVANCED_FACE('',(#13394),#2912,.T.) ;
#48613=ADVANCED_FACE('',(#13395),#2913,.T.) ;
#48614=ADVANCED_FACE('',(#13396),#2914,.T.) ;
#48615=ADVANCED_FACE('',(#13397),#2915,.T.) ;
#48616=ADVANCED_FACE('',(#13398),#2916,.T.) ;
#48617=ADVANCED_FACE('',(#13399),#2917,.T.) ;
#48618=ADVANCED_FACE('',(#13400),#2918,.T.) ;
#48619=ADVANCED_FACE('',(#13401),#2919,.T.) ;
#48620=ADVANCED_FACE('',(#13402),#2920,.T.) ;
#48621=ADVANCED_FACE('',(#13403),#2921,.T.) ;
#48622=ADVANCED_FACE('',(#13404),#45841,.T.) ;
#48623=ADVANCED_FACE('',(#13405),#10552,.T.) ;
#48624=ADVANCED_FACE('',(#13406),#10553,.T.) ;
#48625=ADVANCED_FACE('',(#13407),#10554,.T.) ;
#48626=ADVANCED_FACE('',(#13408),#45842,.T.) ;
#48627=ADVANCED_FACE('',(#13409),#10555,.T.) ;
#48628=ADVANCED_FACE('',(#13410),#10556,.T.) ;
#48629=ADVANCED_FACE('',(#13411),#10557,.T.) ;
#48630=ADVANCED_FACE('',(#13412),#45843,.T.) ;
#48631=ADVANCED_FACE('',(#13413),#10558,.T.) ;
#48632=ADVANCED_FACE('',(#13414),#10559,.T.) ;
#48633=ADVANCED_FACE('',(#13415),#10560,.T.) ;
#48634=ADVANCED_FACE('',(#13416),#45844,.T.) ;
#48635=ADVANCED_FACE('',(#13417),#10561,.T.) ;
#48636=ADVANCED_FACE('',(#13418),#10562,.T.) ;
#48637=ADVANCED_FACE('',(#13419),#10563,.T.) ;
#48638=ADVANCED_FACE('',(#13420),#45845,.T.) ;
#48639=ADVANCED_FACE('',(#13421),#10564,.T.) ;
#48640=ADVANCED_FACE('',(#13422),#10565,.T.) ;
#48641=ADVANCED_FACE('',(#13423),#10566,.T.) ;
#48642=ADVANCED_FACE('',(#13424),#45846,.T.) ;
#48643=ADVANCED_FACE('',(#13425),#10567,.T.) ;
#48644=ADVANCED_FACE('',(#13426),#10568,.T.) ;
#48645=ADVANCED_FACE('',(#13427),#10569,.T.) ;
#48646=ADVANCED_FACE('',(#13428),#45847,.T.) ;
#48647=ADVANCED_FACE('',(#13429),#10570,.T.) ;
#48648=ADVANCED_FACE('',(#13430),#10571,.T.) ;
#48649=ADVANCED_FACE('',(#13431),#10572,.T.) ;
#48650=ADVANCED_FACE('',(#13432),#45848,.T.) ;
#48651=ADVANCED_FACE('',(#13433),#10573,.T.) ;
#48652=ADVANCED_FACE('',(#13434),#10574,.T.) ;
#48653=ADVANCED_FACE('',(#13435),#10575,.T.) ;
#48654=ADVANCED_FACE('',(#13436),#45849,.T.) ;
#48655=ADVANCED_FACE('',(#13437),#10576,.T.) ;
#48656=ADVANCED_FACE('',(#13438),#10577,.T.) ;
#48657=ADVANCED_FACE('',(#13439),#10578,.T.) ;
#48658=ADVANCED_FACE('',(#13440),#45850,.T.) ;
#48659=ADVANCED_FACE('',(#13441),#10579,.T.) ;
#48660=ADVANCED_FACE('',(#13442),#10580,.T.) ;
#48661=ADVANCED_FACE('',(#13443),#10581,.T.) ;
#48662=ADVANCED_FACE('',(#13444),#45851,.T.) ;
#48663=ADVANCED_FACE('',(#13445),#10582,.T.) ;
#48664=ADVANCED_FACE('',(#13446),#45852,.T.) ;
#48665=ADVANCED_FACE('',(#13447),#45853,.T.) ;
#48666=ADVANCED_FACE('',(#13448),#45854,.T.) ;
#48667=ADVANCED_FACE('',(#13449),#10583,.T.) ;
#48668=ADVANCED_FACE('',(#13450),#45855,.T.) ;
#48669=ADVANCED_FACE('',(#13451),#45856,.T.) ;
#48670=ADVANCED_FACE('',(#13452),#45857,.T.) ;
#48671=ADVANCED_FACE('',(#13453),#10584,.T.) ;
#48672=ADVANCED_FACE('',(#13454),#45858,.T.) ;
#48673=ADVANCED_FACE('',(#13455),#45859,.T.) ;
#48674=ADVANCED_FACE('',(#13456),#45860,.T.) ;
#48675=ADVANCED_FACE('',(#13457),#10585,.T.) ;
#48676=ADVANCED_FACE('',(#13458),#45861,.T.) ;
#48677=ADVANCED_FACE('',(#13459),#45862,.T.) ;
#48678=ADVANCED_FACE('',(#13460),#45863,.T.) ;
#48679=ADVANCED_FACE('',(#13461),#10586,.T.) ;
#48680=ADVANCED_FACE('',(#13462),#45864,.T.) ;
#48681=ADVANCED_FACE('',(#13463),#45865,.T.) ;
#48682=ADVANCED_FACE('',(#13464),#45866,.T.) ;
#48683=ADVANCED_FACE('',(#13465),#10587,.T.) ;
#48684=ADVANCED_FACE('',(#13466),#45867,.T.) ;
#48685=ADVANCED_FACE('',(#13467),#45868,.T.) ;
#48686=ADVANCED_FACE('',(#13468),#45869,.T.) ;
#48687=ADVANCED_FACE('',(#13469),#10588,.T.) ;
#48688=ADVANCED_FACE('',(#13470),#45870,.T.) ;
#48689=ADVANCED_FACE('',(#13471),#45871,.T.) ;
#48690=ADVANCED_FACE('',(#13472),#45872,.T.) ;
#48691=ADVANCED_FACE('',(#13473),#10589,.T.) ;
#48692=ADVANCED_FACE('',(#13474),#45873,.T.) ;
#48693=ADVANCED_FACE('',(#13475),#45874,.T.) ;
#48694=ADVANCED_FACE('',(#13476),#45875,.T.) ;
#48695=ADVANCED_FACE('',(#13477),#10590,.T.) ;
#48696=ADVANCED_FACE('',(#13478),#45876,.T.) ;
#48697=ADVANCED_FACE('',(#13479),#45877,.T.) ;
#48698=ADVANCED_FACE('',(#13480),#45878,.T.) ;
#48699=ADVANCED_FACE('',(#13481),#10591,.T.) ;
#48700=ADVANCED_FACE('',(#13482),#45879,.T.) ;
#48701=ADVANCED_FACE('',(#13483),#45880,.T.) ;
#48702=ADVANCED_FACE('',(#13484),#10592,.T.) ;
#48703=ADVANCED_FACE('',(#13485),#2922,.T.) ;
#48704=ADVANCED_FACE('',(#13486),#10593,.T.) ;
#48705=ADVANCED_FACE('',(#13487),#2923,.T.) ;
#48706=ADVANCED_FACE('',(#13488),#2924,.T.) ;
#48707=ADVANCED_FACE('',(#13489),#2925,.T.) ;
#48708=ADVANCED_FACE('',(#13490),#10594,.T.) ;
#48709=ADVANCED_FACE('',(#13491),#2926,.T.) ;
#48710=ADVANCED_FACE('',(#13492),#2927,.T.) ;
#48711=ADVANCED_FACE('',(#13493),#10595,.T.) ;
#48712=ADVANCED_FACE('',(#13494),#2928,.T.) ;
#48713=ADVANCED_FACE('',(#13495),#2929,.T.) ;
#48714=ADVANCED_FACE('',(#13496),#10596,.T.) ;
#48715=ADVANCED_FACE('',(#13497),#2930,.T.) ;
#48716=ADVANCED_FACE('',(#13498),#2931,.T.) ;
#48717=ADVANCED_FACE('',(#13499),#10597,.T.) ;
#48718=ADVANCED_FACE('',(#13500),#2932,.T.) ;
#48719=ADVANCED_FACE('',(#13501),#2933,.T.) ;
#48720=ADVANCED_FACE('',(#13502),#10598,.T.) ;
#48721=ADVANCED_FACE('',(#13503),#2934,.T.) ;
#48722=ADVANCED_FACE('',(#13504),#2935,.T.) ;
#48723=ADVANCED_FACE('',(#13505),#10599,.T.) ;
#48724=ADVANCED_FACE('',(#13506),#2936,.T.) ;
#48725=ADVANCED_FACE('',(#13507),#2937,.T.) ;
#48726=ADVANCED_FACE('',(#13508),#10600,.T.) ;
#48727=ADVANCED_FACE('',(#13509),#2938,.T.) ;
#48728=ADVANCED_FACE('',(#13510),#2939,.T.) ;
#48729=ADVANCED_FACE('',(#13511),#10601,.T.) ;
#48730=ADVANCED_FACE('',(#13512),#2940,.T.) ;
#48731=ADVANCED_FACE('',(#13513),#2941,.T.) ;
#48732=ADVANCED_FACE('',(#13514),#10602,.T.) ;
#48733=ADVANCED_FACE('',(#13515),#10603,.T.) ;
#48734=ADVANCED_FACE('',(#13516),#10604,.T.) ;
#48735=ADVANCED_FACE('',(#13517),#10605,.T.) ;
#48736=ADVANCED_FACE('',(#13518),#10606,.T.) ;
#48737=ADVANCED_FACE('',(#13519),#10607,.T.) ;
#48738=ADVANCED_FACE('',(#13520),#10608,.T.) ;
#48739=ADVANCED_FACE('',(#13521),#10609,.T.) ;
#48740=ADVANCED_FACE('',(#13522),#10610,.T.) ;
#48741=ADVANCED_FACE('',(#13523),#10611,.T.) ;
#48742=ADVANCED_FACE('',(#13524),#10612,.F.) ;
#49075=CLOSED_SHELL('',(#48452,#48453,#48454,#48455,#48456,#48457,#48458,
#48459,#48460,#48461,#48462,#48463,#48464,#48465,#48466,#48467,#48468,#48469,
#48470,#48471,#48472,#48473,#48474,#48475,#48476,#48477,#48478,#48479,#48480,
#48481,#48482,#48483,#48484,#48485,#48486,#48487,#48488,#48489,#48490,#48491,
#48492,#48493,#48494,#48495,#48496,#48497,#48498,#48499,#48500,#48501,#48502,
#48503,#48504,#48505,#48506,#48507,#48508,#48509,#48510,#48511,#48512,#48513,
#48514,#48515,#48516,#48517,#48518,#48519,#48520,#48521,#48522,#48523,#48524,
#48525,#48526,#48527,#48528,#48529,#48530,#48531,#48532,#48533,#48534,#48535,
#48536,#48537,#48538,#48539,#48540,#48541,#48542,#48543,#48544,#48545,#48546,
#48547,#48548,#48549,#48550,#48551,#48552,#48553,#48554,#48555,#48556,#48557,
#48558,#48559,#48560,#48561,#48562,#48563,#48564,#48565,#48566,#48567,#48568,
#48569,#48570,#48571,#48572,#48573,#48574,#48575,#48576,#48577,#48578,#48579,
#48580,#48581,#48582,#48583,#48584,#48585,#48586,#48587,#48588,#48589,#48590,
#48591,#48592,#48593,#48594,#48595,#48596,#48597,#48598,#48599,#48600,#48601,
#48602,#48603,#48604,#48605,#48606,#48607,#48608,#48609,#48610,#48611,#48612,
#48613,#48614,#48615,#48616,#48617,#48618,#48619,#48620,#48621,#48622,#48623,
#48624,#48625,#48626,#48627,#48628,#48629,#48630,#48631,#48632,#48633,#48634,
#48635,#48636,#48637,#48638,#48639,#48640,#48641,#48642,#48643,#48644,#48645,
#48646,#48647,#48648,#48649,#48650,#48651,#48652,#48653,#48654,#48655,#48656,
#48657,#48658,#48659,#48660,#48661,#48662,#48663,#48664,#48665,#48666,#48667,
#48668,#48669,#48670,#48671,#48672,#48673,#48674,#48675,#48676,#48677,#48678,
#48679,#48680,#48681,#48682,#48683,#48684,#48685,#48686,#48687,#48688,#48689,
#48690,#48691,#48692,#48693,#48694,#48695,#48696,#48697,#48698,#48699,#48700,
#48701,#48702,#48703,#48704,#48705,#48706,#48707,#48708,#48709,#48710,#48711,
#48712,#48713,#48714,#48715,#48716,#48717,#48718,#48719,#48720,#48721,#48722,
#48723,#48724,#48725,#48726,#48727,#48728,#48729,#48730,#48731,#48732,#48733,
#48734,#48735,#48736,#48737,#48738,#48739,#48740,#48741,#48742)) ;
#54042=AXIS2_PLACEMENT_3D('',#101745,#67283,#67284) ;
#54043=AXIS2_PLACEMENT_3D('',#101746,#67285,#67286) ;
#54044=AXIS2_PLACEMENT_3D('',#101748,#67287,#67288) ;
#54045=AXIS2_PLACEMENT_3D('',#101750,#67289,#67290) ;
#54046=AXIS2_PLACEMENT_3D('',#101751,#67291,#67292) ;
#54047=AXIS2_PLACEMENT_3D('',#101752,#67293,#67294) ;
#54048=AXIS2_PLACEMENT_3D('',#101770,#67295,#67296) ;
#54049=AXIS2_PLACEMENT_3D('',#101772,#67297,#67298) ;
#54050=AXIS2_PLACEMENT_3D('',#101774,#67299,#67300) ;
#54051=AXIS2_PLACEMENT_3D('',#101775,#67301,#67302) ;
#54052=AXIS2_PLACEMENT_3D('',#101776,#67303,#67304) ;
#54053=AXIS2_PLACEMENT_3D('',#101794,#67305,#67306) ;
#54054=AXIS2_PLACEMENT_3D('',#101796,#67307,#67308) ;
#54055=AXIS2_PLACEMENT_3D('',#101797,#67309,#67310) ;
#54056=AXIS2_PLACEMENT_3D('',#101799,#67311,#67312) ;
#54057=AXIS2_PLACEMENT_3D('',#102014,#67313,#67314) ;
#54058=AXIS2_PLACEMENT_3D('',#102017,#67315,#67316) ;
#54059=AXIS2_PLACEMENT_3D('',#102034,#67317,#67318) ;
#54060=AXIS2_PLACEMENT_3D('',#102049,#67319,#67320) ;
#54061=AXIS2_PLACEMENT_3D('',#102070,#67323,#67324) ;
#54062=AXIS2_PLACEMENT_3D('',#102072,#67325,#67326) ;
#54063=AXIS2_PLACEMENT_3D('',#102090,#67327,#67328) ;
#54064=AXIS2_PLACEMENT_3D('',#102091,#67329,#67330) ;
#54065=AXIS2_PLACEMENT_3D('',#102110,#67333,#67334) ;
#54066=AXIS2_PLACEMENT_3D('',#102112,#67335,#67336) ;
#54067=AXIS2_PLACEMENT_3D('',#102128,#67337,#67338) ;
#54068=AXIS2_PLACEMENT_3D('',#102129,#67339,#67340) ;
#54069=AXIS2_PLACEMENT_3D('',#102150,#67343,#67344) ;
#54070=AXIS2_PLACEMENT_3D('',#102152,#67345,#67346) ;
#54071=AXIS2_PLACEMENT_3D('',#102170,#67347,#67348) ;
#54072=AXIS2_PLACEMENT_3D('',#102171,#67349,#67350) ;
#54073=AXIS2_PLACEMENT_3D('',#102190,#67353,#67354) ;
#54074=AXIS2_PLACEMENT_3D('',#102192,#67355,#67356) ;
#54075=AXIS2_PLACEMENT_3D('',#102208,#67357,#67358) ;
#54076=AXIS2_PLACEMENT_3D('',#102209,#67359,#67360) ;
#54077=AXIS2_PLACEMENT_3D('',#102230,#67363,#67364) ;
#54078=AXIS2_PLACEMENT_3D('',#102232,#67365,#67366) ;
#54079=AXIS2_PLACEMENT_3D('',#102250,#67367,#67368) ;
#54080=AXIS2_PLACEMENT_3D('',#102251,#67369,#67370) ;
#54081=AXIS2_PLACEMENT_3D('',#102270,#67373,#67374) ;
#54082=AXIS2_PLACEMENT_3D('',#102272,#67375,#67376) ;
#54083=AXIS2_PLACEMENT_3D('',#102288,#67377,#67378) ;
#54084=AXIS2_PLACEMENT_3D('',#102289,#67379,#67380) ;
#54085=AXIS2_PLACEMENT_3D('',#102310,#67383,#67384) ;
#54086=AXIS2_PLACEMENT_3D('',#102312,#67385,#67386) ;
#54087=AXIS2_PLACEMENT_3D('',#102330,#67387,#67388) ;
#54088=AXIS2_PLACEMENT_3D('',#102331,#67389,#67390) ;
#54089=AXIS2_PLACEMENT_3D('',#102350,#67393,#67394) ;
#54090=AXIS2_PLACEMENT_3D('',#102352,#67395,#67396) ;
#54091=AXIS2_PLACEMENT_3D('',#102368,#67397,#67398) ;
#54092=AXIS2_PLACEMENT_3D('',#102369,#67399,#67400) ;
#54093=AXIS2_PLACEMENT_3D('',#102390,#67403,#67404) ;
#54094=AXIS2_PLACEMENT_3D('',#102392,#67405,#67406) ;
#54095=AXIS2_PLACEMENT_3D('',#102410,#67407,#67408) ;
#54096=AXIS2_PLACEMENT_3D('',#102411,#67409,#67410) ;
#54097=AXIS2_PLACEMENT_3D('',#102430,#67413,#67414) ;
#54098=AXIS2_PLACEMENT_3D('',#102432,#67415,#67416) ;
#54099=AXIS2_PLACEMENT_3D('',#102448,#67417,#67418) ;
#54100=AXIS2_PLACEMENT_3D('',#102449,#67419,#67420) ;
#54101=AXIS2_PLACEMENT_3D('',#102470,#67423,#67424) ;
#54102=AXIS2_PLACEMENT_3D('',#102472,#67425,#67426) ;
#54103=AXIS2_PLACEMENT_3D('',#102490,#67427,#67428) ;
#54104=AXIS2_PLACEMENT_3D('',#102491,#67429,#67430) ;
#54105=AXIS2_PLACEMENT_3D('',#102510,#67433,#67434) ;
#54106=AXIS2_PLACEMENT_3D('',#102512,#67435,#67436) ;
#54107=AXIS2_PLACEMENT_3D('',#102528,#67437,#67438) ;
#54108=AXIS2_PLACEMENT_3D('',#102529,#67439,#67440) ;
#54109=AXIS2_PLACEMENT_3D('',#102550,#67443,#67444) ;
#54110=AXIS2_PLACEMENT_3D('',#102552,#67445,#67446) ;
#54111=AXIS2_PLACEMENT_3D('',#102570,#67447,#67448) ;
#54112=AXIS2_PLACEMENT_3D('',#102571,#67449,#67450) ;
#54113=AXIS2_PLACEMENT_3D('',#102590,#67453,#67454) ;
#54114=AXIS2_PLACEMENT_3D('',#102592,#67455,#67456) ;
#54115=AXIS2_PLACEMENT_3D('',#102608,#67457,#67458) ;
#54116=AXIS2_PLACEMENT_3D('',#102609,#67459,#67460) ;
#54117=AXIS2_PLACEMENT_3D('',#102630,#67463,#67464) ;
#54118=AXIS2_PLACEMENT_3D('',#102632,#67465,#67466) ;
#54119=AXIS2_PLACEMENT_3D('',#102650,#67467,#67468) ;
#54120=AXIS2_PLACEMENT_3D('',#102651,#67469,#67470) ;
#54121=AXIS2_PLACEMENT_3D('',#102670,#67473,#67474) ;
#54122=AXIS2_PLACEMENT_3D('',#102672,#67475,#67476) ;
#54123=AXIS2_PLACEMENT_3D('',#102688,#67477,#67478) ;
#54124=AXIS2_PLACEMENT_3D('',#102689,#67479,#67480) ;
#54125=AXIS2_PLACEMENT_3D('',#102710,#67483,#67484) ;
#54126=AXIS2_PLACEMENT_3D('',#102712,#67485,#67486) ;
#54127=AXIS2_PLACEMENT_3D('',#102730,#67487,#67488) ;
#54128=AXIS2_PLACEMENT_3D('',#102731,#67489,#67490) ;
#54129=AXIS2_PLACEMENT_3D('',#102750,#67493,#67494) ;
#54130=AXIS2_PLACEMENT_3D('',#102752,#67495,#67496) ;
#54131=AXIS2_PLACEMENT_3D('',#102768,#67497,#67498) ;
#54132=AXIS2_PLACEMENT_3D('',#102769,#67499,#67500) ;
#54133=AXIS2_PLACEMENT_3D('',#102790,#67503,#67504) ;
#54134=AXIS2_PLACEMENT_3D('',#102792,#67505,#67506) ;
#54135=AXIS2_PLACEMENT_3D('',#102810,#67507,#67508) ;
#54136=AXIS2_PLACEMENT_3D('',#102811,#67509,#67510) ;
#54137=AXIS2_PLACEMENT_3D('',#102830,#67513,#67514) ;
#54138=AXIS2_PLACEMENT_3D('',#102832,#67515,#67516) ;
#54139=AXIS2_PLACEMENT_3D('',#102848,#67517,#67518) ;
#54140=AXIS2_PLACEMENT_3D('',#102849,#67519,#67520) ;
#54141=AXIS2_PLACEMENT_3D('',#102870,#67523,#67524) ;
#54142=AXIS2_PLACEMENT_3D('',#102872,#67525,#67526) ;
#54143=AXIS2_PLACEMENT_3D('',#102874,#67527,#67528) ;
#54144=AXIS2_PLACEMENT_3D('',#102891,#67529,#67530) ;
#54145=AXIS2_PLACEMENT_3D('',#102910,#67533,#67534) ;
#54146=AXIS2_PLACEMENT_3D('',#102912,#67535,#67536) ;
#54147=AXIS2_PLACEMENT_3D('',#102914,#67537,#67538) ;
#54148=AXIS2_PLACEMENT_3D('',#102929,#67539,#67540) ;
#54149=AXIS2_PLACEMENT_3D('',#102950,#67543,#67544) ;
#54150=AXIS2_PLACEMENT_3D('',#102952,#67545,#67546) ;
#54151=AXIS2_PLACEMENT_3D('',#102954,#67547,#67548) ;
#54152=AXIS2_PLACEMENT_3D('',#102971,#67549,#67550) ;
#54153=AXIS2_PLACEMENT_3D('',#102990,#67553,#67554) ;
#54154=AXIS2_PLACEMENT_3D('',#102992,#67555,#67556) ;
#54155=AXIS2_PLACEMENT_3D('',#102994,#67557,#67558) ;
#54156=AXIS2_PLACEMENT_3D('',#103009,#67559,#67560) ;
#54157=AXIS2_PLACEMENT_3D('',#103030,#67563,#67564) ;
#54158=AXIS2_PLACEMENT_3D('',#103032,#67565,#67566) ;
#54159=AXIS2_PLACEMENT_3D('',#103034,#67567,#67568) ;
#54160=AXIS2_PLACEMENT_3D('',#103051,#67569,#67570) ;
#54161=AXIS2_PLACEMENT_3D('',#103070,#67573,#67574) ;
#54162=AXIS2_PLACEMENT_3D('',#103072,#67575,#67576) ;
#54163=AXIS2_PLACEMENT_3D('',#103074,#67577,#67578) ;
#54164=AXIS2_PLACEMENT_3D('',#103089,#67579,#67580) ;
#54165=AXIS2_PLACEMENT_3D('',#103110,#67583,#67584) ;
#54166=AXIS2_PLACEMENT_3D('',#103112,#67585,#67586) ;
#54167=AXIS2_PLACEMENT_3D('',#103114,#67587,#67588) ;
#54168=AXIS2_PLACEMENT_3D('',#103131,#67589,#67590) ;
#54169=AXIS2_PLACEMENT_3D('',#103150,#67593,#67594) ;
#54170=AXIS2_PLACEMENT_3D('',#103152,#67595,#67596) ;
#54171=AXIS2_PLACEMENT_3D('',#103154,#67597,#67598) ;
#54172=AXIS2_PLACEMENT_3D('',#103169,#67599,#67600) ;
#54173=AXIS2_PLACEMENT_3D('',#103190,#67603,#67604) ;
#54174=AXIS2_PLACEMENT_3D('',#103192,#67605,#67606) ;
#54175=AXIS2_PLACEMENT_3D('',#103194,#67607,#67608) ;
#54176=AXIS2_PLACEMENT_3D('',#103211,#67609,#67610) ;
#54177=AXIS2_PLACEMENT_3D('',#103230,#67613,#67614) ;
#54178=AXIS2_PLACEMENT_3D('',#103232,#67615,#67616) ;
#54179=AXIS2_PLACEMENT_3D('',#103234,#67617,#67618) ;
#54180=AXIS2_PLACEMENT_3D('',#103249,#67619,#67620) ;
#54181=AXIS2_PLACEMENT_3D('',#103270,#67623,#67624) ;
#54182=AXIS2_PLACEMENT_3D('',#103272,#67625,#67626) ;
#54183=AXIS2_PLACEMENT_3D('',#103274,#67627,#67628) ;
#54184=AXIS2_PLACEMENT_3D('',#103291,#67629,#67630) ;
#54185=AXIS2_PLACEMENT_3D('',#103310,#67633,#67634) ;
#54186=AXIS2_PLACEMENT_3D('',#103312,#67635,#67636) ;
#54187=AXIS2_PLACEMENT_3D('',#103314,#67637,#67638) ;
#54188=AXIS2_PLACEMENT_3D('',#103329,#67639,#67640) ;
#54189=AXIS2_PLACEMENT_3D('',#103350,#67643,#67644) ;
#54190=AXIS2_PLACEMENT_3D('',#103352,#67645,#67646) ;
#54191=AXIS2_PLACEMENT_3D('',#103354,#67647,#67648) ;
#54192=AXIS2_PLACEMENT_3D('',#103371,#67649,#67650) ;
#54193=AXIS2_PLACEMENT_3D('',#103390,#67653,#67654) ;
#54194=AXIS2_PLACEMENT_3D('',#103392,#67655,#67656) ;
#54195=AXIS2_PLACEMENT_3D('',#103394,#67657,#67658) ;
#54196=AXIS2_PLACEMENT_3D('',#103409,#67659,#67660) ;
#54197=AXIS2_PLACEMENT_3D('',#103430,#67663,#67664) ;
#54198=AXIS2_PLACEMENT_3D('',#103432,#67665,#67666) ;
#54199=AXIS2_PLACEMENT_3D('',#103434,#67667,#67668) ;
#54200=AXIS2_PLACEMENT_3D('',#103451,#67669,#67670) ;
#54201=AXIS2_PLACEMENT_3D('',#103470,#67673,#67674) ;
#54202=AXIS2_PLACEMENT_3D('',#103472,#67675,#67676) ;
#54203=AXIS2_PLACEMENT_3D('',#103474,#67677,#67678) ;
#54204=AXIS2_PLACEMENT_3D('',#103489,#67679,#67680) ;
#54205=AXIS2_PLACEMENT_3D('',#103510,#67683,#67684) ;
#54206=AXIS2_PLACEMENT_3D('',#103512,#67685,#67686) ;
#54207=AXIS2_PLACEMENT_3D('',#103514,#67687,#67688) ;
#54208=AXIS2_PLACEMENT_3D('',#103531,#67689,#67690) ;
#54209=AXIS2_PLACEMENT_3D('',#103550,#67693,#67694) ;
#54210=AXIS2_PLACEMENT_3D('',#103552,#67695,#67696) ;
#54211=AXIS2_PLACEMENT_3D('',#103554,#67697,#67698) ;
#54212=AXIS2_PLACEMENT_3D('',#103569,#67699,#67700) ;
#54213=AXIS2_PLACEMENT_3D('',#103590,#67703,#67704) ;
#54214=AXIS2_PLACEMENT_3D('',#103592,#67705,#67706) ;
#54215=AXIS2_PLACEMENT_3D('',#103594,#67707,#67708) ;
#54216=AXIS2_PLACEMENT_3D('',#103611,#67709,#67710) ;
#54217=AXIS2_PLACEMENT_3D('',#103614,#67713,#67714) ;
#54218=AXIS2_PLACEMENT_3D('',#103620,#67718,#67719) ;
#54219=AXIS2_PLACEMENT_3D('',#103623,#67721,#67722) ;
#54220=AXIS2_PLACEMENT_3D('',#103624,#67723,#67724) ;
#54221=AXIS2_PLACEMENT_3D('',#103628,#67727,#67728) ;
#54222=AXIS2_PLACEMENT_3D('',#103631,#67730,#67731) ;
#54223=AXIS2_PLACEMENT_3D('',#103632,#67732,#67733) ;
#54224=AXIS2_PLACEMENT_3D('',#103636,#67736,#67737) ;
#54225=AXIS2_PLACEMENT_3D('',#103639,#67739,#67740) ;
#54226=AXIS2_PLACEMENT_3D('',#103640,#67741,#67742) ;
#54227=AXIS2_PLACEMENT_3D('',#103644,#67745,#67746) ;
#54228=AXIS2_PLACEMENT_3D('',#103647,#67748,#67749) ;
#54229=AXIS2_PLACEMENT_3D('',#103648,#67750,#67751) ;
#54230=AXIS2_PLACEMENT_3D('',#103652,#67754,#67755) ;
#54231=AXIS2_PLACEMENT_3D('',#103655,#67757,#67758) ;
#54232=AXIS2_PLACEMENT_3D('',#103656,#67759,#67760) ;
#54233=AXIS2_PLACEMENT_3D('',#103660,#67763,#67764) ;
#54234=AXIS2_PLACEMENT_3D('',#103663,#67766,#67767) ;
#54235=AXIS2_PLACEMENT_3D('',#103664,#67768,#67769) ;
#54236=AXIS2_PLACEMENT_3D('',#103668,#67772,#67773) ;
#54237=AXIS2_PLACEMENT_3D('',#103671,#67775,#67776) ;
#54238=AXIS2_PLACEMENT_3D('',#103672,#67777,#67778) ;
#54239=AXIS2_PLACEMENT_3D('',#103676,#67781,#67782) ;
#54240=AXIS2_PLACEMENT_3D('',#103679,#67784,#67785) ;
#54241=AXIS2_PLACEMENT_3D('',#103680,#67786,#67787) ;
#54242=AXIS2_PLACEMENT_3D('',#103684,#67790,#67791) ;
#54243=AXIS2_PLACEMENT_3D('',#103687,#67793,#67794) ;
#54244=AXIS2_PLACEMENT_3D('',#103688,#67795,#67796) ;
#54245=AXIS2_PLACEMENT_3D('',#103692,#67799,#67800) ;
#54246=AXIS2_PLACEMENT_3D('',#103695,#67802,#67803) ;
#54247=AXIS2_PLACEMENT_3D('',#103696,#67804,#67805) ;
#54248=AXIS2_PLACEMENT_3D('',#103700,#67808,#67809) ;
#54249=AXIS2_PLACEMENT_3D('',#103703,#67811,#67812) ;
#54250=AXIS2_PLACEMENT_3D('',#103704,#67813,#67814) ;
#54251=AXIS2_PLACEMENT_3D('',#103708,#67817,#67818) ;
#54252=AXIS2_PLACEMENT_3D('',#103711,#67820,#67821) ;
#54253=AXIS2_PLACEMENT_3D('',#103712,#67822,#67823) ;
#54254=AXIS2_PLACEMENT_3D('',#103716,#67826,#67827) ;
#54255=AXIS2_PLACEMENT_3D('',#103719,#67829,#67830) ;
#54256=AXIS2_PLACEMENT_3D('',#103720,#67831,#67832) ;
#54257=AXIS2_PLACEMENT_3D('',#103724,#67835,#67836) ;
#54258=AXIS2_PLACEMENT_3D('',#103727,#67838,#67839) ;
#54259=AXIS2_PLACEMENT_3D('',#103728,#67840,#67841) ;
#54260=AXIS2_PLACEMENT_3D('',#103732,#67844,#67845) ;
#54261=AXIS2_PLACEMENT_3D('',#103735,#67847,#67848) ;
#54262=AXIS2_PLACEMENT_3D('',#103736,#67849,#67850) ;
#54263=AXIS2_PLACEMENT_3D('',#103740,#67853,#67854) ;
#54264=AXIS2_PLACEMENT_3D('',#103743,#67856,#67857) ;
#54265=AXIS2_PLACEMENT_3D('',#103744,#67858,#67859) ;
#54266=AXIS2_PLACEMENT_3D('',#103748,#67862,#67863) ;
#54267=AXIS2_PLACEMENT_3D('',#103751,#67865,#67866) ;
#54268=AXIS2_PLACEMENT_3D('',#103752,#67867,#67868) ;
#54269=AXIS2_PLACEMENT_3D('',#103756,#67871,#67872) ;
#54270=AXIS2_PLACEMENT_3D('',#103759,#67874,#67875) ;
#54271=AXIS2_PLACEMENT_3D('',#103760,#67876,#67877) ;
#54272=AXIS2_PLACEMENT_3D('',#103764,#67880,#67881) ;
#54273=AXIS2_PLACEMENT_3D('',#103767,#67883,#67884) ;
#54274=AXIS2_PLACEMENT_3D('',#103768,#67885,#67886) ;
#54275=AXIS2_PLACEMENT_3D('',#103772,#67889,#67890) ;
#54276=AXIS2_PLACEMENT_3D('',#103775,#67892,#67893) ;
#54277=AXIS2_PLACEMENT_3D('',#103776,#67894,#67895) ;
#54278=AXIS2_PLACEMENT_3D('',#103777,#67896,#67897) ;
#54279=AXIS2_PLACEMENT_3D('',#103778,#67898,#67899) ;
#54280=AXIS2_PLACEMENT_3D('',#103779,#67900,#67901) ;
#54281=AXIS2_PLACEMENT_3D('',#103780,#67902,#67903) ;
#54282=AXIS2_PLACEMENT_3D('',#103781,#67904,#67905) ;
#54283=AXIS2_PLACEMENT_3D('',#103782,#67906,#67907) ;
#54284=AXIS2_PLACEMENT_3D('',#103783,#67908,#67909) ;
#54285=AXIS2_PLACEMENT_3D('',#103784,#67910,#67911) ;
#54286=AXIS2_PLACEMENT_3D('',#103785,#67912,#67913) ;
#54287=AXIS2_PLACEMENT_3D('',#103786,#67914,#67915) ;
#54288=AXIS2_PLACEMENT_3D('',#103787,#67916,#67917) ;
#54289=AXIS2_PLACEMENT_3D('',#103788,#67918,#67919) ;
#54290=AXIS2_PLACEMENT_3D('',#103789,#67920,#67921) ;
#54291=AXIS2_PLACEMENT_3D('',#103790,#67922,#67923) ;
#54292=AXIS2_PLACEMENT_3D('',#103791,#67924,#67925) ;
#54293=AXIS2_PLACEMENT_3D('',#103792,#67926,#67927) ;
#54294=AXIS2_PLACEMENT_3D('',#103793,#67928,#67929) ;
#54295=AXIS2_PLACEMENT_3D('',#103794,#67930,#67931) ;
#54296=AXIS2_PLACEMENT_3D('',#103795,#67932,#67933) ;
#54297=AXIS2_PLACEMENT_3D('',#103796,#67934,#67935) ;
#54298=AXIS2_PLACEMENT_3D('',#103797,#67936,#67937) ;
#54299=AXIS2_PLACEMENT_3D('',#103798,#67938,#67939) ;
#54300=AXIS2_PLACEMENT_3D('',#103799,#67940,#67941) ;
#54301=AXIS2_PLACEMENT_3D('',#103800,#67942,#67943) ;
#54302=AXIS2_PLACEMENT_3D('',#103801,#67944,#67945) ;
#54303=AXIS2_PLACEMENT_3D('',#103802,#67946,#67947) ;
#54304=AXIS2_PLACEMENT_3D('',#103803,#67948,#67949) ;
#54305=AXIS2_PLACEMENT_3D('',#103804,#67950,#67951) ;
#54306=AXIS2_PLACEMENT_3D('',#103805,#67952,#67953) ;
#54307=AXIS2_PLACEMENT_3D('',#103806,#67954,#67955) ;
#54308=AXIS2_PLACEMENT_3D('',#103807,#67956,#67957) ;
#54309=AXIS2_PLACEMENT_3D('',#103808,#67958,#67959) ;
#54310=AXIS2_PLACEMENT_3D('',#103809,#67960,#67961) ;
#54311=AXIS2_PLACEMENT_3D('',#103810,#67962,#67963) ;
#54312=AXIS2_PLACEMENT_3D('',#103811,#67964,#67965) ;
#54313=AXIS2_PLACEMENT_3D('',#103812,#67966,#67967) ;
#54314=AXIS2_PLACEMENT_3D('',#103814,#67968,#67969) ;
#54315=AXIS2_PLACEMENT_3D('',#103815,#67970,#67971) ;
#54316=AXIS2_PLACEMENT_3D('',#103816,#67972,#67973) ;
#54317=AXIS2_PLACEMENT_3D('',#103817,#67974,#67975) ;
#54318=AXIS2_PLACEMENT_3D('',#103818,#67976,#67977) ;
#54319=AXIS2_PLACEMENT_3D('',#103819,#67978,#67979) ;
#54320=AXIS2_PLACEMENT_3D('',#103820,#67980,#67981) ;
#54321=AXIS2_PLACEMENT_3D('',#103822,#67982,#67983) ;
#54322=AXIS2_PLACEMENT_3D('',#103824,#67984,#67985) ;
#54323=AXIS2_PLACEMENT_3D('',#103826,#67986,#67987) ;
#54324=AXIS2_PLACEMENT_3D('',#103828,#67988,#67989) ;
#54325=AXIS2_PLACEMENT_3D('',#103830,#67990,#67991) ;
#54326=AXIS2_PLACEMENT_3D('',#103832,#67992,#67993) ;
#54327=AXIS2_PLACEMENT_3D('',#103834,#67994,#67995) ;
#54328=AXIS2_PLACEMENT_3D('',#103836,#67996,#67997) ;
#54329=AXIS2_PLACEMENT_3D('',#103838,#67998,#67999) ;
#54330=AXIS2_PLACEMENT_3D('',#103840,#68000,#68001) ;
#54331=AXIS2_PLACEMENT_3D('',#103842,#68002,#68003) ;
#54332=AXIS2_PLACEMENT_3D('',#103844,#68004,#68005) ;
#54333=AXIS2_PLACEMENT_3D('',#103846,#68006,#68007) ;
#54334=AXIS2_PLACEMENT_3D('',#103848,#68008,#68009) ;
#54335=AXIS2_PLACEMENT_3D('',#103850,#68010,#68011) ;
#54336=AXIS2_PLACEMENT_3D('',#103852,#68012,#68013) ;
#54337=AXIS2_PLACEMENT_3D('',#103854,#68014,#68015) ;
#54338=AXIS2_PLACEMENT_3D('',#103856,#68016,#68017) ;
#54339=AXIS2_PLACEMENT_3D('',#103858,#68018,#68019) ;
#54340=AXIS2_PLACEMENT_3D('',#103860,#68020,#68021) ;
#54341=AXIS2_PLACEMENT_3D('',#103862,#68022,#68023) ;
#54342=AXIS2_PLACEMENT_3D('',#103864,#68024,#68025) ;
#54343=AXIS2_PLACEMENT_3D('',#103866,#68026,#68027) ;
#54344=AXIS2_PLACEMENT_3D('',#103868,#68028,#68029) ;
#54345=AXIS2_PLACEMENT_3D('',#103870,#68030,#68031) ;
#54346=AXIS2_PLACEMENT_3D('',#103872,#68032,#68033) ;
#54347=AXIS2_PLACEMENT_3D('',#103874,#68034,#68035) ;
#54348=AXIS2_PLACEMENT_3D('',#103876,#68036,#68037) ;
#54349=AXIS2_PLACEMENT_3D('',#103878,#68038,#68039) ;
#54350=AXIS2_PLACEMENT_3D('',#103880,#68040,#68041) ;
#54351=AXIS2_PLACEMENT_3D('',#103882,#68042,#68043) ;
#54352=AXIS2_PLACEMENT_3D('',#103884,#68044,#68045) ;
#54353=AXIS2_PLACEMENT_3D('',#103886,#68046,#68047) ;
#54354=AXIS2_PLACEMENT_3D('',#103888,#68048,#68049) ;
#54355=AXIS2_PLACEMENT_3D('',#103890,#68050,#68051) ;
#54356=AXIS2_PLACEMENT_3D('',#103892,#68052,#68053) ;
#54357=AXIS2_PLACEMENT_3D('',#103894,#68054,#68055) ;
#54358=AXIS2_PLACEMENT_3D('',#103896,#68056,#68057) ;
#54359=AXIS2_PLACEMENT_3D('',#103898,#68058,#68059) ;
#54360=AXIS2_PLACEMENT_3D('',#103900,#68060,#68061) ;
#54361=AXIS2_PLACEMENT_3D('',#103902,#68062,#68063) ;
#54362=AXIS2_PLACEMENT_3D('',#103903,#68064,#68065) ;
#54363=AXIS2_PLACEMENT_3D('',#103904,#68066,#68067) ;
#54364=AXIS2_PLACEMENT_3D('',#103908,#68069,#68070) ;
#54365=AXIS2_PLACEMENT_3D('',#103910,#68072,#68073) ;
#54366=AXIS2_PLACEMENT_3D('',#103914,#68075,#68076) ;
#54367=AXIS2_PLACEMENT_3D('',#103916,#68078,#68079) ;
#54368=AXIS2_PLACEMENT_3D('',#103920,#68081,#68082) ;
#54369=AXIS2_PLACEMENT_3D('',#103922,#68084,#68085) ;
#54370=AXIS2_PLACEMENT_3D('',#103926,#68087,#68088) ;
#54371=AXIS2_PLACEMENT_3D('',#103928,#68090,#68091) ;
#54372=AXIS2_PLACEMENT_3D('',#103932,#68093,#68094) ;
#54373=AXIS2_PLACEMENT_3D('',#103934,#68096,#68097) ;
#54374=AXIS2_PLACEMENT_3D('',#103938,#68099,#68100) ;
#54375=AXIS2_PLACEMENT_3D('',#103940,#68102,#68103) ;
#54376=AXIS2_PLACEMENT_3D('',#103944,#68105,#68106) ;
#54377=AXIS2_PLACEMENT_3D('',#103946,#68108,#68109) ;
#54378=AXIS2_PLACEMENT_3D('',#103950,#68111,#68112) ;
#54379=AXIS2_PLACEMENT_3D('',#103952,#68114,#68115) ;
#54380=AXIS2_PLACEMENT_3D('',#103956,#68117,#68118) ;
#54381=AXIS2_PLACEMENT_3D('',#103958,#68120,#68121) ;
#54382=AXIS2_PLACEMENT_3D('',#103962,#68123,#68124) ;
#54383=AXIS2_PLACEMENT_3D('',#103964,#68126,#68127) ;
#54384=AXIS2_PLACEMENT_3D('',#103968,#68129,#68130) ;
#54385=AXIS2_PLACEMENT_3D('',#103970,#68132,#68133) ;
#54386=AXIS2_PLACEMENT_3D('',#103974,#68135,#68136) ;
#54387=AXIS2_PLACEMENT_3D('',#103976,#68138,#68139) ;
#54388=AXIS2_PLACEMENT_3D('',#103980,#68141,#68142) ;
#54389=AXIS2_PLACEMENT_3D('',#103982,#68144,#68145) ;
#54390=AXIS2_PLACEMENT_3D('',#103986,#68147,#68148) ;
#54391=AXIS2_PLACEMENT_3D('',#103988,#68150,#68151) ;
#54392=AXIS2_PLACEMENT_3D('',#103992,#68153,#68154) ;
#54393=AXIS2_PLACEMENT_3D('',#103994,#68156,#68157) ;
#54394=AXIS2_PLACEMENT_3D('',#103998,#68159,#68160) ;
#54395=AXIS2_PLACEMENT_3D('',#104000,#68162,#68163) ;
#54396=AXIS2_PLACEMENT_3D('',#104004,#68165,#68166) ;
#54397=AXIS2_PLACEMENT_3D('',#104006,#68168,#68169) ;
#54398=AXIS2_PLACEMENT_3D('',#104010,#68171,#68172) ;
#54399=AXIS2_PLACEMENT_3D('',#104012,#68174,#68175) ;
#54400=AXIS2_PLACEMENT_3D('',#104016,#68177,#68178) ;
#54401=AXIS2_PLACEMENT_3D('',#104018,#68180,#68181) ;
#54402=AXIS2_PLACEMENT_3D('',#104022,#68183,#68184) ;
#54403=AXIS2_PLACEMENT_3D('',#104024,#68186,#68187) ;
#54404=AXIS2_PLACEMENT_3D('',#104041,#68188,#68189) ;
#54405=AXIS2_PLACEMENT_3D('',#104056,#68190,#68191) ;
#54406=AXIS2_PLACEMENT_3D('',#104075,#68193,#68194) ;
#54407=AXIS2_PLACEMENT_3D('',#104094,#68196,#68197) ;
#54408=AXIS2_PLACEMENT_3D('',#104127,#68199,#68200) ;
#54409=AXIS2_PLACEMENT_3D('',#104142,#68201,#68202) ;
#54410=AXIS2_PLACEMENT_3D('',#104159,#68203,#68204) ;
#54411=AXIS2_PLACEMENT_3D('',#104193,#68206,#68207) ;
#54412=AXIS2_PLACEMENT_3D('',#104224,#68208,#68209) ;
#54413=AXIS2_PLACEMENT_3D('',#104239,#68210,#68211) ;
#54414=AXIS2_PLACEMENT_3D('',#104256,#68212,#68213) ;
#54415=AXIS2_PLACEMENT_3D('',#104290,#68215,#68216) ;
#54416=AXIS2_PLACEMENT_3D('',#104321,#68217,#68218) ;
#54417=AXIS2_PLACEMENT_3D('',#104336,#68219,#68220) ;
#54418=AXIS2_PLACEMENT_3D('',#104353,#68221,#68222) ;
#54419=AXIS2_PLACEMENT_3D('',#104387,#68224,#68225) ;
#54420=AXIS2_PLACEMENT_3D('',#104418,#68226,#68227) ;
#54421=AXIS2_PLACEMENT_3D('',#104433,#68228,#68229) ;
#54422=AXIS2_PLACEMENT_3D('',#104450,#68230,#68231) ;
#54423=AXIS2_PLACEMENT_3D('',#104484,#68233,#68234) ;
#54424=AXIS2_PLACEMENT_3D('',#104515,#68235,#68236) ;
#54425=AXIS2_PLACEMENT_3D('',#104530,#68237,#68238) ;
#54426=AXIS2_PLACEMENT_3D('',#104547,#68239,#68240) ;
#54427=AXIS2_PLACEMENT_3D('',#104581,#68242,#68243) ;
#54428=AXIS2_PLACEMENT_3D('',#104612,#68244,#68245) ;
#54429=AXIS2_PLACEMENT_3D('',#104627,#68246,#68247) ;
#54430=AXIS2_PLACEMENT_3D('',#104644,#68248,#68249) ;
#54431=AXIS2_PLACEMENT_3D('',#104678,#68251,#68252) ;
#54432=AXIS2_PLACEMENT_3D('',#104709,#68253,#68254) ;
#54433=AXIS2_PLACEMENT_3D('',#104724,#68255,#68256) ;
#54434=AXIS2_PLACEMENT_3D('',#104741,#68257,#68258) ;
#54435=AXIS2_PLACEMENT_3D('',#104775,#68260,#68261) ;
#54436=AXIS2_PLACEMENT_3D('',#104806,#68262,#68263) ;
#54437=AXIS2_PLACEMENT_3D('',#104821,#68264,#68265) ;
#54438=AXIS2_PLACEMENT_3D('',#104838,#68266,#68267) ;
#54439=AXIS2_PLACEMENT_3D('',#104872,#68269,#68270) ;
#54440=AXIS2_PLACEMENT_3D('',#104903,#68271,#68272) ;
#54441=AXIS2_PLACEMENT_3D('',#104918,#68273,#68274) ;
#54442=AXIS2_PLACEMENT_3D('',#104935,#68275,#68276) ;
#54443=AXIS2_PLACEMENT_3D('',#104966,#68277,#68278) ;
#54444=AXIS2_PLACEMENT_3D('',#104997,#68279,#68280) ;
#54445=AXIS2_PLACEMENT_3D('',#105012,#68281,#68282) ;
#54446=AXIS2_PLACEMENT_3D('',#105029,#68283,#68284) ;
#54447=AXIS2_PLACEMENT_3D('',#105030,#68285,#68286) ;
#54448=AXIS2_PLACEMENT_3D('',#105031,#68287,#68288) ;
#54449=AXIS2_PLACEMENT_3D('',#105033,#68289,#68290) ;
#54450=AXIS2_PLACEMENT_3D('',#105048,#68291,#68292) ;
#54451=AXIS2_PLACEMENT_3D('',#105067,#68294,#68295) ;
#54452=AXIS2_PLACEMENT_3D('',#105068,#68296,#68297) ;
#54453=AXIS2_PLACEMENT_3D('',#105069,#68298,#68299) ;
#54454=AXIS2_PLACEMENT_3D('',#105070,#68300,#68301) ;
#54455=AXIS2_PLACEMENT_3D('',#105072,#68302,#68303) ;
#54456=AXIS2_PLACEMENT_3D('',#105087,#68304,#68305) ;
#54457=AXIS2_PLACEMENT_3D('',#105106,#68307,#68308) ;
#54458=AXIS2_PLACEMENT_3D('',#105107,#68309,#68310) ;
#54459=AXIS2_PLACEMENT_3D('',#105108,#68311,#68312) ;
#54460=AXIS2_PLACEMENT_3D('',#105109,#68313,#68314) ;
#54461=AXIS2_PLACEMENT_3D('',#105111,#68315,#68316) ;
#54462=AXIS2_PLACEMENT_3D('',#105126,#68317,#68318) ;
#54463=AXIS2_PLACEMENT_3D('',#105145,#68320,#68321) ;
#54464=AXIS2_PLACEMENT_3D('',#105146,#68322,#68323) ;
#54465=AXIS2_PLACEMENT_3D('',#105147,#68324,#68325) ;
#54466=AXIS2_PLACEMENT_3D('',#105148,#68326,#68327) ;
#54467=AXIS2_PLACEMENT_3D('',#105150,#68328,#68329) ;
#54468=AXIS2_PLACEMENT_3D('',#105165,#68330,#68331) ;
#54469=AXIS2_PLACEMENT_3D('',#105184,#68333,#68334) ;
#54470=AXIS2_PLACEMENT_3D('',#105185,#68335,#68336) ;
#54471=AXIS2_PLACEMENT_3D('',#105186,#68337,#68338) ;
#54472=AXIS2_PLACEMENT_3D('',#105187,#68339,#68340) ;
#54473=AXIS2_PLACEMENT_3D('',#105189,#68341,#68342) ;
#54474=AXIS2_PLACEMENT_3D('',#105204,#68343,#68344) ;
#54475=AXIS2_PLACEMENT_3D('',#105223,#68346,#68347) ;
#54476=AXIS2_PLACEMENT_3D('',#105224,#68348,#68349) ;
#54477=AXIS2_PLACEMENT_3D('',#105225,#68350,#68351) ;
#54478=AXIS2_PLACEMENT_3D('',#105226,#68352,#68353) ;
#54479=AXIS2_PLACEMENT_3D('',#105228,#68354,#68355) ;
#54480=AXIS2_PLACEMENT_3D('',#105243,#68356,#68357) ;
#54481=AXIS2_PLACEMENT_3D('',#105262,#68359,#68360) ;
#54482=AXIS2_PLACEMENT_3D('',#105263,#68361,#68362) ;
#54483=AXIS2_PLACEMENT_3D('',#105264,#68363,#68364) ;
#54484=AXIS2_PLACEMENT_3D('',#105265,#68365,#68366) ;
#54485=AXIS2_PLACEMENT_3D('',#105267,#68367,#68368) ;
#54486=AXIS2_PLACEMENT_3D('',#105282,#68369,#68370) ;
#54487=AXIS2_PLACEMENT_3D('',#105301,#68372,#68373) ;
#54488=AXIS2_PLACEMENT_3D('',#105302,#68374,#68375) ;
#54489=AXIS2_PLACEMENT_3D('',#105303,#68376,#68377) ;
#54490=AXIS2_PLACEMENT_3D('',#105304,#68378,#68379) ;
#54491=AXIS2_PLACEMENT_3D('',#105306,#68380,#68381) ;
#54492=AXIS2_PLACEMENT_3D('',#105321,#68382,#68383) ;
#54493=AXIS2_PLACEMENT_3D('',#105340,#68385,#68386) ;
#54494=AXIS2_PLACEMENT_3D('',#105341,#68387,#68388) ;
#54495=AXIS2_PLACEMENT_3D('',#105342,#68389,#68390) ;
#54496=AXIS2_PLACEMENT_3D('',#105343,#68391,#68392) ;
#54497=AXIS2_PLACEMENT_3D('',#105345,#68393,#68394) ;
#54498=AXIS2_PLACEMENT_3D('',#105360,#68395,#68396) ;
#54499=AXIS2_PLACEMENT_3D('',#105379,#68398,#68399) ;
#54500=AXIS2_PLACEMENT_3D('',#105380,#68400,#68401) ;
#54501=AXIS2_PLACEMENT_3D('',#105381,#68402,#68403) ;
#54502=AXIS2_PLACEMENT_3D('',#105382,#68404,#68405) ;
#54503=AXIS2_PLACEMENT_3D('',#105383,#68406,#68407) ;
#54504=AXIS2_PLACEMENT_3D('',#105386,#68410,#68411) ;
#54505=AXIS2_PLACEMENT_3D('',#105388,#68413,#68414) ;
#54506=AXIS2_PLACEMENT_3D('',#105390,#68416,#68417) ;
#54507=AXIS2_PLACEMENT_3D('',#105391,#68418,#68419) ;
#54508=AXIS2_PLACEMENT_3D('',#105394,#68422,#68423) ;
#54509=AXIS2_PLACEMENT_3D('',#105397,#68426,#68427) ;
#54510=AXIS2_PLACEMENT_3D('',#105398,#68428,#68429) ;
#54511=AXIS2_PLACEMENT_3D('',#105401,#68432,#68433) ;
#54512=AXIS2_PLACEMENT_3D('',#105404,#68436,#68437) ;
#54513=AXIS2_PLACEMENT_3D('',#105405,#68438,#68439) ;
#54514=AXIS2_PLACEMENT_3D('',#105408,#68442,#68443) ;
#54515=AXIS2_PLACEMENT_3D('',#105411,#68446,#68447) ;
#54516=AXIS2_PLACEMENT_3D('',#105412,#68448,#68449) ;
#54517=AXIS2_PLACEMENT_3D('',#105415,#68452,#68453) ;
#54518=AXIS2_PLACEMENT_3D('',#105418,#68456,#68457) ;
#54519=AXIS2_PLACEMENT_3D('',#105419,#68458,#68459) ;
#54520=AXIS2_PLACEMENT_3D('',#105422,#68462,#68463) ;
#54521=AXIS2_PLACEMENT_3D('',#105425,#68466,#68467) ;
#54522=AXIS2_PLACEMENT_3D('',#105426,#68468,#68469) ;
#54523=AXIS2_PLACEMENT_3D('',#105429,#68472,#68473) ;
#54524=AXIS2_PLACEMENT_3D('',#105432,#68476,#68477) ;
#54525=AXIS2_PLACEMENT_3D('',#105433,#68478,#68479) ;
#54526=AXIS2_PLACEMENT_3D('',#105436,#68482,#68483) ;
#54527=AXIS2_PLACEMENT_3D('',#105439,#68486,#68487) ;
#54528=AXIS2_PLACEMENT_3D('',#105440,#68488,#68489) ;
#54529=AXIS2_PLACEMENT_3D('',#105443,#68492,#68493) ;
#54530=AXIS2_PLACEMENT_3D('',#105446,#68496,#68497) ;
#54531=AXIS2_PLACEMENT_3D('',#105447,#68498,#68499) ;
#54532=AXIS2_PLACEMENT_3D('',#105450,#68502,#68503) ;
#54533=AXIS2_PLACEMENT_3D('',#105452,#68505,#68506) ;
#54534=AXIS2_PLACEMENT_3D('',#105453,#68507,#68508) ;
#54535=AXIS2_PLACEMENT_3D('',#105454,#68509,#68510) ;
#54536=AXIS2_PLACEMENT_3D('',#105455,#68511,#68512) ;
#54537=AXIS2_PLACEMENT_3D('',#105456,#68513,#68514) ;
#54538=AXIS2_PLACEMENT_3D('',#105457,#68515,#68516) ;
#54539=AXIS2_PLACEMENT_3D('',#105458,#68517,#68518) ;
#54540=AXIS2_PLACEMENT_3D('',#105459,#68519,#68520) ;
#54541=AXIS2_PLACEMENT_3D('',#105460,#68521,#68522) ;
#54542=AXIS2_PLACEMENT_3D('',#105461,#68523,#68524) ;
#54543=AXIS2_PLACEMENT_3D('',#105462,#68525,#68526) ;
#67283=DIRECTION('axis',(0.,0.,1.)) ;
#67284=DIRECTION('refdir',(1.,0.,0.)) ;
#67285=DIRECTION('center_axis',(0.,-1.,0.)) ;
#67286=DIRECTION('ref_axis',(1.,0.,0.)) ;
#67287=DIRECTION('center_axis',(0.,-1.,0.)) ;
#67288=DIRECTION('ref_axis',(-1.,0.,0.)) ;
#67289=DIRECTION('center_axis',(0.,0.,1.)) ;
#67290=DIRECTION('ref_axis',(-1.,0.,0.)) ;
#67291=DIRECTION('center_axis',(0.,-1.,0.)) ;
#67292=DIRECTION('ref_axis',(1.,0.,0.)) ;
#67293=DIRECTION('center_axis',(0.,1.,0.)) ;
#67294=DIRECTION('ref_axis',(-1.,0.,0.)) ;
#67295=DIRECTION('center_axis',(0.,-1.,0.)) ;
#67296=DIRECTION('ref_axis',(0.,0.,-1.)) ;
#67297=DIRECTION('center_axis',(0.,1.,0.)) ;
#67298=DIRECTION('ref_axis',(-1.,0.,0.)) ;
#67299=DIRECTION('center_axis',(1.,0.,0.)) ;
#67300=DIRECTION('ref_axis',(0.,0.,1.)) ;
#67301=DIRECTION('center_axis',(0.,1.,0.)) ;
#67302=DIRECTION('ref_axis',(-1.,0.,0.)) ;
#67303=DIRECTION('center_axis',(0.,1.,0.)) ;
#67304=DIRECTION('ref_axis',(-1.,0.,0.)) ;
#67305=DIRECTION('center_axis',(0.,1.,0.)) ;
#67306=DIRECTION('ref_axis',(-1.,0.,0.)) ;
#67307=DIRECTION('center_axis',(0.,-1.,0.)) ;
#67308=DIRECTION('ref_axis',(-1.,0.,0.)) ;
#67309=DIRECTION('center_axis',(0.,1.,0.)) ;
#67310=DIRECTION('ref_axis',(-1.,0.,0.)) ;
#67311=DIRECTION('center_axis',(0.,1.,0.)) ;
#67312=DIRECTION('ref_axis',(-1.,0.,0.)) ;
#67313=DIRECTION('center_axis',(0.,-1.,0.)) ;
#67314=DIRECTION('ref_axis',(0.,0.,-1.)) ;
#67315=DIRECTION('center_axis',(0.,-1.,0.)) ;
#67316=DIRECTION('ref_axis',(-0.406305370818768,0.,0.913737350469939)) ;
#67317=DIRECTION('center_axis',(0.,-1.,0.)) ;
#67318=DIRECTION('ref_axis',(-0.453990499739547,0.,0.891006524188368)) ;
#67319=DIRECTION('center_axis',(0.309016994374948,0.,-0.951056516295154)) ;
#67320=DIRECTION('ref_axis',(-0.672498511963948,-0.707106781186557,-0.218508012224408)) ;
#67321=DIRECTION('',(-0.309016994374947,0.,0.951056516295154)) ;
#67322=DIRECTION('',(0.309016994374948,0.,-0.951056516295154)) ;
#67323=DIRECTION('center_axis',(0.,-1.,0.)) ;
#67324=DIRECTION('ref_axis',(-0.309016994374914,0.,0.951056516295165)) ;
#67325=DIRECTION('center_axis',(0.,1.,0.)) ;
#67326=DIRECTION('ref_axis',(-0.309016994374945,0.,0.951056516295154)) ;
#67327=DIRECTION('center_axis',(0.,-1.,0.)) ;
#67328=DIRECTION('ref_axis',(-0.309016994374945,0.,0.951056516295154)) ;
#67329=DIRECTION('center_axis',(-0.309016994374948,0.,0.951056516295154)) ;
#67330=DIRECTION('ref_axis',(0.672498511963948,-0.707106781186557,0.218508012224408)) ;
#67331=DIRECTION('',(0.309016994374948,0.,-0.951056516295154)) ;
#67332=DIRECTION('',(-0.309016994374948,0.,0.951056516295154)) ;
#67333=DIRECTION('center_axis',(0.,-1.,0.)) ;
#67334=DIRECTION('ref_axis',(0.,0.,-1.)) ;
#67335=DIRECTION('center_axis',(0.,-1.,0.)) ;
#67336=DIRECTION('ref_axis',(-0.406305370818768,0.,0.913737350469939)) ;
#67337=DIRECTION('center_axis',(0.,-1.,0.)) ;
#67338=DIRECTION('ref_axis',(-0.156434465040232,0.,0.987688340595138)) ;
#67339=DIRECTION('center_axis',(1.11022302462516E-16,0.,-1.)) ;
#67340=DIRECTION('ref_axis',(-0.707106781186527,-0.707106781186568,-7.85046229341867E-17)) ;
#67341=DIRECTION('',(-1.11022302462516E-16,0.,1.)) ;
#67342=DIRECTION('',(1.11022302462516E-16,0.,-1.)) ;
#67343=DIRECTION('center_axis',(0.,-1.,0.)) ;
#67344=DIRECTION('ref_axis',(-9.9475983006414E-14,0.,1.)) ;
#67345=DIRECTION('center_axis',(0.,1.,0.)) ;
#67346=DIRECTION('ref_axis',(0.,0.,1.)) ;
#67347=DIRECTION('center_axis',(0.,-1.,0.)) ;
#67348=DIRECTION('ref_axis',(0.,0.,1.)) ;
#67349=DIRECTION('center_axis',(-1.11022302462516E-16,0.,1.)) ;
#67350=DIRECTION('ref_axis',(0.707106781186506,-0.707106781186589,7.85046229341844E-17)) ;
#67351=DIRECTION('',(1.11022302462516E-16,0.,-1.)) ;
#67352=DIRECTION('',(-1.11022302462516E-16,0.,1.)) ;
#67353=DIRECTION('center_axis',(0.,-1.,0.)) ;
#67354=DIRECTION('ref_axis',(0.,0.,-1.)) ;
#67355=DIRECTION('center_axis',(0.,-1.,0.)) ;
#67356=DIRECTION('ref_axis',(-0.406305370818768,0.,0.913737350469939)) ;
#67357=DIRECTION('center_axis',(0.,-1.,0.)) ;
#67358=DIRECTION('ref_axis',(0.156434465040233,0.,0.987688340595137)) ;
#67359=DIRECTION('center_axis',(-0.309016994374947,0.,-0.951056516295154)) ;
#67360=DIRECTION('ref_axis',(-0.672498511963948,-0.707106781186557,0.218508012224407)) ;
#67361=DIRECTION('',(0.309016994374947,0.,0.951056516295154)) ;
#67362=DIRECTION('',(-0.309016994374947,0.,-0.951056516295154)) ;
#67363=DIRECTION('center_axis',(0.,-1.,0.)) ;
#67364=DIRECTION('ref_axis',(0.309016994374783,0.,0.951056516295207)) ;
#67365=DIRECTION('center_axis',(0.,1.,0.)) ;
#67366=DIRECTION('ref_axis',(0.309016994374945,0.,0.951056516295154)) ;
#67367=DIRECTION('center_axis',(0.,-1.,0.)) ;
#67368=DIRECTION('ref_axis',(0.309016994374945,0.,0.951056516295154)) ;
#67369=DIRECTION('center_axis',(0.309016994374947,0.,0.951056516295154)) ;
#67370=DIRECTION('ref_axis',(0.672498511963948,-0.707106781186557,-0.218508012224407)) ;
#67371=DIRECTION('',(-0.309016994374947,0.,-0.951056516295154)) ;
#67372=DIRECTION('',(0.309016994374947,0.,0.951056516295154)) ;
#67373=DIRECTION('center_axis',(0.,-1.,0.)) ;
#67374=DIRECTION('ref_axis',(0.,0.,-1.)) ;
#67375=DIRECTION('center_axis',(0.,-1.,0.)) ;
#67376=DIRECTION('ref_axis',(-0.406305370818768,0.,0.913737350469939)) ;
#67377=DIRECTION('center_axis',(0.,-1.,0.)) ;
#67378=DIRECTION('ref_axis',(0.453990499739549,0.,0.891006524188367)) ;
#67379=DIRECTION('center_axis',(-0.587785252292473,0.,-0.809016994374948)) ;
#67380=DIRECTION('ref_axis',(-0.572061402817695,-0.707106781186534,0.415626937777461)) ;
#67381=DIRECTION('',(0.587785252292473,0.,0.809016994374948)) ;
#67382=DIRECTION('',(-0.587785252292473,0.,-0.809016994374947)) ;
#67383=DIRECTION('center_axis',(0.,-1.,0.)) ;
#67384=DIRECTION('ref_axis',(0.587785252292717,0.,0.80901699437477)) ;
#67385=DIRECTION('center_axis',(0.,1.,0.)) ;
#67386=DIRECTION('ref_axis',(0.587785252292468,0.,0.809016994374951)) ;
#67387=DIRECTION('center_axis',(0.,-1.,0.)) ;
#67388=DIRECTION('ref_axis',(0.587785252292468,0.,0.809016994374951)) ;
#67389=DIRECTION('center_axis',(0.587785252292473,0.,0.809016994374948)) ;
#67390=DIRECTION('ref_axis',(0.572061402817668,-0.707106781186568,-0.415626937777441)) ;
#67391=DIRECTION('',(-0.587785252292473,0.,-0.809016994374947)) ;
#67392=DIRECTION('',(0.587785252292473,0.,0.809016994374947)) ;
#67393=DIRECTION('center_axis',(0.,-1.,0.)) ;
#67394=DIRECTION('ref_axis',(0.,0.,-1.)) ;
#67395=DIRECTION('center_axis',(0.,-1.,0.)) ;
#67396=DIRECTION('ref_axis',(-0.406305370818768,0.,0.913737350469939)) ;
#67397=DIRECTION('center_axis',(0.,-1.,0.)) ;
#67398=DIRECTION('ref_axis',(0.70710678118655,0.,0.707106781186545)) ;
#67399=DIRECTION('center_axis',(-0.809016994374947,0.,-0.587785252292473)) ;
#67400=DIRECTION('ref_axis',(-0.415626937777452,-0.707106781186551,0.572061402817681)) ;
#67401=DIRECTION('',(0.809016994374947,0.,0.587785252292473)) ;
#67402=DIRECTION('',(-0.809016994374947,0.,-0.587785252292473)) ;
#67403=DIRECTION('center_axis',(0.,-1.,0.)) ;
#67404=DIRECTION('ref_axis',(0.809016994375165,0.,0.587785252292174)) ;
#67405=DIRECTION('center_axis',(0.,1.,0.)) ;
#67406=DIRECTION('ref_axis',(0.809016994374947,0.,0.587785252292474)) ;
#67407=DIRECTION('center_axis',(0.,-1.,0.)) ;
#67408=DIRECTION('ref_axis',(0.809016994374947,0.,0.587785252292474)) ;
#67409=DIRECTION('center_axis',(0.809016994374947,0.,0.587785252292473)) ;
#67410=DIRECTION('ref_axis',(0.415626937777427,-0.707106781186592,-0.572061402817648)) ;
#67411=DIRECTION('',(-0.809016994374947,0.,-0.587785252292473)) ;
#67412=DIRECTION('',(0.809016994374947,0.,0.587785252292473)) ;
#67413=DIRECTION('center_axis',(0.,-1.,0.)) ;
#67414=DIRECTION('ref_axis',(0.,0.,-1.)) ;
#67415=DIRECTION('center_axis',(0.,-1.,0.)) ;
#67416=DIRECTION('ref_axis',(-0.406305370818768,0.,0.913737350469939)) ;
#67417=DIRECTION('center_axis',(0.,-1.,0.)) ;
#67418=DIRECTION('ref_axis',(0.891006524188368,0.,0.453990499739546)) ;
#67419=DIRECTION('center_axis',(-0.951056516295154,0.,-0.309016994374948)) ;
#67420=DIRECTION('ref_axis',(-0.2185080122244,-0.707106781186583,0.672498511963923)) ;
#67421=DIRECTION('',(0.951056516295153,0.,0.309016994374948)) ;
#67422=DIRECTION('',(-0.951056516295153,0.,-0.309016994374948)) ;
#67423=DIRECTION('center_axis',(0.,-1.,0.)) ;
#67424=DIRECTION('ref_axis',(0.95105651629519,0.,0.309016994374834)) ;
#67425=DIRECTION('center_axis',(0.,1.,0.)) ;
#67426=DIRECTION('ref_axis',(0.951056516295153,0.,0.309016994374948)) ;
#67427=DIRECTION('center_axis',(0.,-1.,0.)) ;
#67428=DIRECTION('ref_axis',(0.951056516295153,0.,0.309016994374948)) ;
#67429=DIRECTION('center_axis',(0.951056516295154,0.,0.309016994374948)) ;
#67430=DIRECTION('ref_axis',(0.218508012224406,-0.707106781186563,-0.672498511963942)) ;
#67431=DIRECTION('',(-0.951056516295153,0.,-0.309016994374948)) ;
#67432=DIRECTION('',(0.951056516295153,0.,0.309016994374948)) ;
#67433=DIRECTION('center_axis',(0.,-1.,0.)) ;
#67434=DIRECTION('ref_axis',(0.,0.,-1.)) ;
#67435=DIRECTION('center_axis',(0.,-1.,0.)) ;
#67436=DIRECTION('ref_axis',(-0.406305370818768,0.,0.913737350469939)) ;
#67437=DIRECTION('center_axis',(0.,-1.,0.)) ;
#67438=DIRECTION('ref_axis',(0.987688340595138,0.,0.15643446504023)) ;
#67439=DIRECTION('center_axis',(-1.,0.,-2.22044604925031E-16)) ;
#67440=DIRECTION('ref_axis',(-1.57009245868373E-16,-0.707106781186568,0.707106781186527)) ;
#67441=DIRECTION('',(1.,0.,2.22044604925031E-16)) ;
#67442=DIRECTION('',(-1.,0.,-2.22044604925031E-16)) ;
#67443=DIRECTION('center_axis',(0.,-1.,0.)) ;
#67444=DIRECTION('ref_axis',(1.,0.,-1.49213974509621E-13)) ;
#67445=DIRECTION('center_axis',(0.,1.,0.)) ;
#67446=DIRECTION('ref_axis',(1.,0.,0.)) ;
#67447=DIRECTION('center_axis',(0.,-1.,0.)) ;
#67448=DIRECTION('ref_axis',(1.,0.,0.)) ;
#67449=DIRECTION('center_axis',(1.,0.,2.22044604925031E-16)) ;
#67450=DIRECTION('ref_axis',(1.57009245868373E-16,-0.707106781186568,-0.707106781186527)) ;
#67451=DIRECTION('',(-1.,0.,-2.22044604925031E-16)) ;
#67452=DIRECTION('',(1.,0.,2.22044604925031E-16)) ;
#67453=DIRECTION('center_axis',(0.,-1.,0.)) ;
#67454=DIRECTION('ref_axis',(0.,0.,-1.)) ;
#67455=DIRECTION('center_axis',(0.,-1.,0.)) ;
#67456=DIRECTION('ref_axis',(-0.406305370818768,0.,0.913737350469939)) ;
#67457=DIRECTION('center_axis',(0.,-1.,0.)) ;
#67458=DIRECTION('ref_axis',(0.987688340595138,0.,-0.156434465040229)) ;
#67459=DIRECTION('center_axis',(-0.951056516295154,0.,0.309016994374947)) ;
#67460=DIRECTION('ref_axis',(0.218508012224405,-0.707106781186563,0.672498511963943)) ;
#67461=DIRECTION('',(0.951056516295154,0.,-0.309016994374947)) ;
#67462=DIRECTION('',(-0.951056516295154,0.,0.309016994374947)) ;
#67463=DIRECTION('center_axis',(0.,-1.,0.)) ;
#67464=DIRECTION('ref_axis',(0.,0.,-1.)) ;
#67465=DIRECTION('center_axis',(0.,1.,0.)) ;
#67466=DIRECTION('ref_axis',(0.951056516295153,0.,-0.309016994374948)) ;
#67467=DIRECTION('center_axis',(0.,-1.,0.)) ;
#67468=DIRECTION('ref_axis',(0.951056516295153,0.,-0.309016994374948)) ;
#67469=DIRECTION('center_axis',(0.951056516295154,0.,-0.309016994374947)) ;
#67470=DIRECTION('ref_axis',(-0.218508012224405,-0.707106781186563,-0.672498511963943)) ;
#67471=DIRECTION('',(-0.951056516295154,0.,0.309016994374947)) ;
#67472=DIRECTION('',(0.951056516295154,0.,-0.309016994374947)) ;
#67473=DIRECTION('center_axis',(0.,-1.,0.)) ;
#67474=DIRECTION('ref_axis',(0.,0.,-1.)) ;
#67475=DIRECTION('center_axis',(0.,-1.,0.)) ;
#67476=DIRECTION('ref_axis',(-0.406305370818768,0.,0.913737350469939)) ;
#67477=DIRECTION('center_axis',(0.,-1.,0.)) ;
#67478=DIRECTION('ref_axis',(0.891006524188368,0.,-0.453990499739547)) ;
#67479=DIRECTION('center_axis',(-0.809016994374948,0.,0.587785252292473)) ;
#67480=DIRECTION('ref_axis',(0.415626937777451,-0.707106781186551,0.572061402817682)) ;
#67481=DIRECTION('',(0.809016994374948,0.,-0.587785252292473)) ;
#67482=DIRECTION('',(-0.809016994374948,0.,0.587785252292473)) ;
#67483=DIRECTION('center_axis',(0.,-1.,0.)) ;
#67484=DIRECTION('ref_axis',(0.,0.,-1.)) ;
#67485=DIRECTION('center_axis',(0.,1.,0.)) ;
#67486=DIRECTION('ref_axis',(0.809016994374947,0.,-0.587785252292474)) ;
#67487=DIRECTION('center_axis',(0.,-1.,0.)) ;
#67488=DIRECTION('ref_axis',(0.809016994374947,0.,-0.587785252292474)) ;
#67489=DIRECTION('center_axis',(0.809016994374948,0.,-0.587785252292473)) ;
#67490=DIRECTION('ref_axis',(-0.415626937777437,-0.707106781186575,-0.572061402817662)) ;
#67491=DIRECTION('',(-0.809016994374948,0.,0.587785252292473)) ;
#67492=DIRECTION('',(0.809016994374948,0.,-0.587785252292473)) ;
#67493=DIRECTION('center_axis',(0.,-1.,0.)) ;
#67494=DIRECTION('ref_axis',(0.,0.,-1.)) ;
#67495=DIRECTION('center_axis',(0.,-1.,0.)) ;
#67496=DIRECTION('ref_axis',(-0.406305370818768,0.,0.913737350469939)) ;
#67497=DIRECTION('center_axis',(0.,-1.,0.)) ;
#67498=DIRECTION('ref_axis',(0.707106781186547,0.,-0.707106781186547)) ;
#67499=DIRECTION('center_axis',(-0.587785252292473,0.,0.809016994374947)) ;
#67500=DIRECTION('ref_axis',(0.572061402817686,-0.707106781186546,0.415626937777454)) ;
#67501=DIRECTION('',(0.587785252292473,0.,-0.809016994374947)) ;
#67502=DIRECTION('',(-0.587785252292473,0.,0.809016994374947)) ;
#67503=DIRECTION('center_axis',(0.,-1.,0.)) ;
#67504=DIRECTION('ref_axis',(0.,0.,-1.)) ;
#67505=DIRECTION('center_axis',(0.,1.,0.)) ;
#67506=DIRECTION('ref_axis',(0.587785252292468,0.,-0.809016994374951)) ;
#67507=DIRECTION('center_axis',(0.,-1.,0.)) ;
#67508=DIRECTION('ref_axis',(0.587785252292468,0.,-0.809016994374951)) ;
#67509=DIRECTION('center_axis',(0.587785252292473,0.,-0.809016994374947)) ;
#67510=DIRECTION('ref_axis',(-0.572061402817695,-0.707106781186534,-0.415626937777461)) ;
#67511=DIRECTION('',(-0.587785252292473,0.,0.809016994374947)) ;
#67512=DIRECTION('',(0.587785252292473,0.,-0.809016994374947)) ;
#67513=DIRECTION('center_axis',(0.,-1.,0.)) ;
#67514=DIRECTION('ref_axis',(0.,0.,-1.)) ;
#67515=DIRECTION('center_axis',(0.,-1.,0.)) ;
#67516=DIRECTION('ref_axis',(-0.406305370818768,0.,0.913737350469939)) ;
#67517=DIRECTION('center_axis',(0.,-1.,0.)) ;
#67518=DIRECTION('ref_axis',(0.453990499739547,0.,-0.891006524188368)) ;
#67519=DIRECTION('center_axis',(-0.309016994374948,0.,0.951056516295154)) ;
#67520=DIRECTION('ref_axis',(0.672498511963948,-0.707106781186557,0.218508012224408)) ;
#67521=DIRECTION('',(-0.309016994374948,0.,0.951056516295153)) ;
#67522=DIRECTION('',(0.309016994374948,0.,-0.951056516295153)) ;
#67523=DIRECTION('center_axis',(0.,-1.,0.)) ;
#67524=DIRECTION('ref_axis',(0.,0.,-1.)) ;
#67525=DIRECTION('center_axis',(0.,-1.,0.)) ;
#67526=DIRECTION('ref_axis',(0.309016994374945,0.,-0.951056516295154)) ;
#67527=DIRECTION('center_axis',(0.,1.,0.)) ;
#67528=DIRECTION('ref_axis',(0.309016994374945,0.,-0.951056516295154)) ;
#67529=DIRECTION('center_axis',(0.309016994374948,0.,-0.951056516295154)) ;
#67530=DIRECTION('ref_axis',(-0.672498511963948,-0.707106781186557,-0.218508012224408)) ;
#67531=DIRECTION('',(0.309016994374948,0.,-0.951056516295153)) ;
#67532=DIRECTION('',(-0.309016994374948,0.,0.951056516295153)) ;
#67533=DIRECTION('center_axis',(0.,-1.,0.)) ;
#67534=DIRECTION('ref_axis',(0.,0.,-1.)) ;
#67535=DIRECTION('center_axis',(0.,-1.,0.)) ;
#67536=DIRECTION('ref_axis',(0.156434465040232,0.,-0.987688340595138)) ;
#67537=DIRECTION('center_axis',(0.,-1.,0.)) ;
#67538=DIRECTION('ref_axis',(-0.406305370818768,0.,0.913737350469939)) ;
#67539=DIRECTION('center_axis',(0.,0.,1.)) ;
#67540=DIRECTION('ref_axis',(0.707106781186506,-0.707106781186589,0.)) ;
#67541=DIRECTION('',(0.,0.,1.)) ;
#67542=DIRECTION('',(0.,0.,-1.)) ;
#67543=DIRECTION('center_axis',(0.,-1.,0.)) ;
#67544=DIRECTION('ref_axis',(0.,0.,-1.)) ;
#67545=DIRECTION('center_axis',(0.,-1.,0.)) ;
#67546=DIRECTION('ref_axis',(0.,0.,-1.)) ;
#67547=DIRECTION('center_axis',(0.,1.,0.)) ;
#67548=DIRECTION('ref_axis',(0.,0.,-1.)) ;
#67549=DIRECTION('center_axis',(0.,0.,-1.)) ;
#67550=DIRECTION('ref_axis',(-0.707106781186527,-0.707106781186568,0.)) ;
#67551=DIRECTION('',(0.,0.,-1.)) ;
#67552=DIRECTION('',(0.,0.,1.)) ;
#67553=DIRECTION('center_axis',(0.,-1.,0.)) ;
#67554=DIRECTION('ref_axis',(0.,0.,-1.)) ;
#67555=DIRECTION('center_axis',(0.,-1.,0.)) ;
#67556=DIRECTION('ref_axis',(-0.156434465040231,0.,-0.987688340595138)) ;
#67557=DIRECTION('center_axis',(0.,-1.,0.)) ;
#67558=DIRECTION('ref_axis',(-0.406305370818768,0.,0.913737350469939)) ;
#67559=DIRECTION('center_axis',(0.309016994374947,0.,0.951056516295154)) ;
#67560=DIRECTION('ref_axis',(0.672498511963948,-0.707106781186557,-0.218508012224407)) ;
#67561=DIRECTION('',(0.309016994374947,0.,0.951056516295154)) ;
#67562=DIRECTION('',(-0.309016994374947,0.,-0.951056516295154)) ;
#67563=DIRECTION('center_axis',(0.,-1.,0.)) ;
#67564=DIRECTION('ref_axis',(0.,0.,-1.)) ;
#67565=DIRECTION('center_axis',(0.,-1.,0.)) ;
#67566=DIRECTION('ref_axis',(-0.309016994374945,0.,-0.951056516295154)) ;
#67567=DIRECTION('center_axis',(0.,1.,0.)) ;
#67568=DIRECTION('ref_axis',(-0.309016994374945,0.,-0.951056516295154)) ;
#67569=DIRECTION('center_axis',(-0.309016994374947,0.,-0.951056516295154)) ;
#67570=DIRECTION('ref_axis',(-0.672498511963948,-0.707106781186557,0.218508012224407)) ;
#67571=DIRECTION('',(-0.309016994374947,0.,-0.951056516295154)) ;
#67572=DIRECTION('',(0.309016994374947,0.,0.951056516295154)) ;
#67573=DIRECTION('center_axis',(0.,-1.,0.)) ;
#67574=DIRECTION('ref_axis',(0.,0.,-1.)) ;
#67575=DIRECTION('center_axis',(0.,-1.,0.)) ;
#67576=DIRECTION('ref_axis',(-0.453990499739546,0.,-0.891006524188368)) ;
#67577=DIRECTION('center_axis',(0.,-1.,0.)) ;
#67578=DIRECTION('ref_axis',(-0.406305370818768,0.,0.913737350469939)) ;
#67579=DIRECTION('center_axis',(0.587785252292473,0.,0.809016994374948)) ;
#67580=DIRECTION('ref_axis',(0.572061402817682,-0.707106781186551,-0.415626937777451)) ;
#67581=DIRECTION('',(0.587785252292473,0.,0.809016994374947)) ;
#67582=DIRECTION('',(-0.587785252292473,0.,-0.809016994374947)) ;
#67583=DIRECTION('center_axis',(0.,-1.,0.)) ;
#67584=DIRECTION('ref_axis',(0.,0.,-1.)) ;
#67585=DIRECTION('center_axis',(0.,-1.,0.)) ;
#67586=DIRECTION('ref_axis',(-0.587785252292474,0.,-0.809016994374947)) ;
#67587=DIRECTION('center_axis',(0.,1.,0.)) ;
#67588=DIRECTION('ref_axis',(-0.587785252292474,0.,-0.809016994374947)) ;
#67589=DIRECTION('center_axis',(-0.587785252292473,0.,-0.809016994374948)) ;
#67590=DIRECTION('ref_axis',(-0.572061402817672,-0.707106781186563,0.415626937777444)) ;
#67591=DIRECTION('',(-0.587785252292473,0.,-0.809016994374947)) ;
#67592=DIRECTION('',(0.587785252292473,0.,0.809016994374947)) ;
#67593=DIRECTION('center_axis',(0.,-1.,0.)) ;
#67594=DIRECTION('ref_axis',(0.,0.,-1.)) ;
#67595=DIRECTION('center_axis',(0.,-1.,0.)) ;
#67596=DIRECTION('ref_axis',(-0.707106781186547,0.,-0.707106781186548)) ;
#67597=DIRECTION('center_axis',(0.,-1.,0.)) ;
#67598=DIRECTION('ref_axis',(-0.406305370818768,0.,0.913737350469939)) ;
#67599=DIRECTION('center_axis',(0.809016994374947,0.,0.587785252292473)) ;
#67600=DIRECTION('ref_axis',(0.415626937777442,-0.707106781186568,-0.572061402817668)) ;
#67601=DIRECTION('',(0.809016994374947,0.,0.587785252292473)) ;
#67602=DIRECTION('',(-0.809016994374947,0.,-0.587785252292473)) ;
#67603=DIRECTION('center_axis',(0.,-1.,0.)) ;
#67604=DIRECTION('ref_axis',(0.,0.,-1.)) ;
#67605=DIRECTION('center_axis',(0.,-1.,0.)) ;
#67606=DIRECTION('ref_axis',(-0.809016994374947,0.,-0.587785252292474)) ;
#67607=DIRECTION('center_axis',(0.,1.,0.)) ;
#67608=DIRECTION('ref_axis',(-0.809016994374947,0.,-0.587785252292474)) ;
#67609=DIRECTION('center_axis',(-0.809016994374947,0.,-0.587785252292473)) ;
#67610=DIRECTION('ref_axis',(-0.415626937777444,-0.707106781186563,0.572061402817672)) ;
#67611=DIRECTION('',(-0.809016994374947,0.,-0.587785252292473)) ;
#67612=DIRECTION('',(0.809016994374947,0.,0.587785252292473)) ;
#67613=DIRECTION('center_axis',(0.,-1.,0.)) ;
#67614=DIRECTION('ref_axis',(0.,0.,-1.)) ;
#67615=DIRECTION('center_axis',(0.,-1.,0.)) ;
#67616=DIRECTION('ref_axis',(-0.891006524188368,0.,-0.453990499739547)) ;
#67617=DIRECTION('center_axis',(0.,-1.,0.)) ;
#67618=DIRECTION('ref_axis',(-0.406305370818768,0.,0.913737350469939)) ;
#67619=DIRECTION('center_axis',(0.951056516295154,0.,0.309016994374948)) ;
#67620=DIRECTION('ref_axis',(0.218508012224408,-0.707106781186557,-0.672498511963948)) ;
#67621=DIRECTION('',(0.951056516295154,0.,0.309016994374948)) ;
#67622=DIRECTION('',(-0.951056516295154,0.,-0.309016994374948)) ;
#67623=DIRECTION('center_axis',(0.,-1.,0.)) ;
#67624=DIRECTION('ref_axis',(0.,0.,-1.)) ;
#67625=DIRECTION('center_axis',(0.,-1.,0.)) ;
#67626=DIRECTION('ref_axis',(-0.951056516295154,0.,-0.309016994374945)) ;
#67627=DIRECTION('center_axis',(0.,1.,0.)) ;
#67628=DIRECTION('ref_axis',(-0.951056516295154,0.,-0.309016994374945)) ;
#67629=DIRECTION('center_axis',(-0.951056516295154,0.,-0.309016994374948)) ;
#67630=DIRECTION('ref_axis',(-0.218508012224408,-0.707106781186557,0.672498511963948)) ;
#67631=DIRECTION('',(-0.951056516295154,0.,-0.309016994374948)) ;
#67632=DIRECTION('',(0.951056516295154,0.,0.309016994374948)) ;
#67633=DIRECTION('center_axis',(0.,-1.,0.)) ;
#67634=DIRECTION('ref_axis',(0.,0.,-1.)) ;
#67635=DIRECTION('center_axis',(0.,-1.,0.)) ;
#67636=DIRECTION('ref_axis',(-0.987688340595138,0.,-0.156434465040231)) ;
#67637=DIRECTION('center_axis',(0.,-1.,0.)) ;
#67638=DIRECTION('ref_axis',(-0.406305370818768,0.,0.913737350469939)) ;
#67639=DIRECTION('center_axis',(1.,0.,5.55111512312578E-17)) ;
#67640=DIRECTION('ref_axis',(3.92523114670932E-17,-0.707106781186568,-0.707106781186527)) ;
#67641=DIRECTION('',(1.,0.,5.55111512312578E-17)) ;
#67642=DIRECTION('',(-1.,0.,-5.55111512312578E-17)) ;
#67643=DIRECTION('center_axis',(0.,-1.,0.)) ;
#67644=DIRECTION('ref_axis',(-1.,0.,4.90274487674469E-13)) ;
#67645=DIRECTION('center_axis',(0.,-1.,0.)) ;
#67646=DIRECTION('ref_axis',(-1.,0.,0.)) ;
#67647=DIRECTION('center_axis',(0.,1.,0.)) ;
#67648=DIRECTION('ref_axis',(-1.,0.,0.)) ;
#67649=DIRECTION('center_axis',(-1.,0.,-5.55111512312578E-17)) ;
#67650=DIRECTION('ref_axis',(-3.92523114670932E-17,-0.707106781186568,0.707106781186527)) ;
#67651=DIRECTION('',(-1.,0.,-5.55111512312578E-17)) ;
#67652=DIRECTION('',(1.,0.,5.55111512312578E-17)) ;
#67653=DIRECTION('center_axis',(0.,-1.,0.)) ;
#67654=DIRECTION('ref_axis',(0.,0.,-1.)) ;
#67655=DIRECTION('center_axis',(0.,-1.,0.)) ;
#67656=DIRECTION('ref_axis',(-0.987688340595138,0.,0.156434465040229)) ;
#67657=DIRECTION('center_axis',(0.,-1.,0.)) ;
#67658=DIRECTION('ref_axis',(-0.406305370818768,0.,0.913737350469939)) ;
#67659=DIRECTION('center_axis',(0.951056516295154,0.,-0.309016994374947)) ;
#67660=DIRECTION('ref_axis',(-0.218508012224407,-0.707106781186557,-0.672498511963948)) ;
#67661=DIRECTION('',(0.951056516295154,0.,-0.309016994374947)) ;
#67662=DIRECTION('',(-0.951056516295154,0.,0.309016994374947)) ;
#67663=DIRECTION('center_axis',(0.,-1.,0.)) ;
#67664=DIRECTION('ref_axis',(-0.951056516295038,0.,0.309016994375305)) ;
#67665=DIRECTION('center_axis',(0.,-1.,0.)) ;
#67666=DIRECTION('ref_axis',(-0.951056516295154,0.,0.309016994374945)) ;
#67667=DIRECTION('center_axis',(0.,1.,0.)) ;
#67668=DIRECTION('ref_axis',(-0.951056516295154,0.,0.309016994374945)) ;
#67669=DIRECTION('center_axis',(-0.951056516295154,0.,0.309016994374947)) ;
#67670=DIRECTION('ref_axis',(0.218508012224407,-0.707106781186557,0.672498511963948)) ;
#67671=DIRECTION('',(-0.951056516295154,0.,0.309016994374947)) ;
#67672=DIRECTION('',(0.951056516295154,0.,-0.309016994374947)) ;
#67673=DIRECTION('center_axis',(0.,-1.,0.)) ;
#67674=DIRECTION('ref_axis',(0.,0.,-1.)) ;
#67675=DIRECTION('center_axis',(0.,-1.,0.)) ;
#67676=DIRECTION('ref_axis',(-0.891006524188369,0.,0.453990499739545)) ;
#67677=DIRECTION('center_axis',(0.,-1.,0.)) ;
#67678=DIRECTION('ref_axis',(-0.406305370818768,0.,0.913737350469939)) ;
#67679=DIRECTION('center_axis',(0.809016994374948,0.,-0.587785252292473)) ;
#67680=DIRECTION('ref_axis',(-0.415626937777444,-0.707106781186563,-0.572061402817672)) ;
#67681=DIRECTION('',(0.809016994374947,0.,-0.587785252292473)) ;
#67682=DIRECTION('',(-0.809016994374947,0.,0.587785252292473)) ;
#67683=DIRECTION('center_axis',(0.,-1.,0.)) ;
#67684=DIRECTION('ref_axis',(-0.809016994374941,0.,0.587785252292482)) ;
#67685=DIRECTION('center_axis',(0.,-1.,0.)) ;
#67686=DIRECTION('ref_axis',(-0.809016994374947,0.,0.587785252292474)) ;
#67687=DIRECTION('center_axis',(0.,1.,0.)) ;
#67688=DIRECTION('ref_axis',(-0.809016994374947,0.,0.587785252292474)) ;
#67689=DIRECTION('center_axis',(-0.809016994374948,0.,0.587785252292473)) ;
#67690=DIRECTION('ref_axis',(0.415626937777444,-0.707106781186563,0.572061402817672)) ;
#67691=DIRECTION('',(-0.809016994374947,0.,0.587785252292473)) ;
#67692=DIRECTION('',(0.809016994374947,0.,-0.587785252292473)) ;
#67693=DIRECTION('center_axis',(0.,-1.,0.)) ;
#67694=DIRECTION('ref_axis',(0.,0.,-1.)) ;
#67695=DIRECTION('center_axis',(0.,-1.,0.)) ;
#67696=DIRECTION('ref_axis',(-0.707106781186548,0.,0.707106781186547)) ;
#67697=DIRECTION('center_axis',(0.,-1.,0.)) ;
#67698=DIRECTION('ref_axis',(-0.406305370818768,0.,0.913737350469939)) ;
#67699=DIRECTION('center_axis',(0.587785252292473,0.,-0.809016994374947)) ;
#67700=DIRECTION('ref_axis',(-0.572061402817681,-0.707106781186551,-0.415626937777452)) ;
#67701=DIRECTION('',(0.587785252292473,0.,-0.809016994374947)) ;
#67702=DIRECTION('',(-0.587785252292473,0.,0.809016994374947)) ;
#67703=DIRECTION('center_axis',(0.,-1.,0.)) ;
#67704=DIRECTION('ref_axis',(-0.587785252292018,0.,0.809016994375278)) ;
#67705=DIRECTION('center_axis',(0.,-1.,0.)) ;
#67706=DIRECTION('ref_axis',(-0.587785252292474,0.,0.809016994374947)) ;
#67707=DIRECTION('center_axis',(0.,1.,0.)) ;
#67708=DIRECTION('ref_axis',(-0.587785252292474,0.,0.809016994374947)) ;
#67709=DIRECTION('center_axis',(-0.587785252292473,0.,0.809016994374947)) ;
#67710=DIRECTION('ref_axis',(0.572061402817672,-0.707106781186563,0.415626937777444)) ;
#67711=DIRECTION('',(-0.587785252292473,0.,0.809016994374947)) ;
#67712=DIRECTION('',(0.587785252292473,0.,-0.809016994374947)) ;
#67713=DIRECTION('center_axis',(0.951056516295154,0.,0.309016994374948)) ;
#67714=DIRECTION('ref_axis',(-0.309016994374948,0.,0.951056516295153)) ;
#67715=DIRECTION('',(0.,-1.,0.)) ;
#67716=DIRECTION('',(0.309016994374948,0.,-0.951056516295153)) ;
#67717=DIRECTION('',(0.,1.,0.)) ;
#67718=DIRECTION('center_axis',(0.,-1.,0.)) ;
#67719=DIRECTION('ref_axis',(0.309016994374938,0.,-0.951056516295157)) ;
#67720=DIRECTION('',(0.,-1.,0.)) ;
#67721=DIRECTION('center_axis',(0.,1.,0.)) ;
#67722=DIRECTION('ref_axis',(0.309016994374945,0.,-0.951056516295154)) ;
#67723=DIRECTION('center_axis',(-0.951056516295154,0.,-0.309016994374948)) ;
#67724=DIRECTION('ref_axis',(0.309016994374948,0.,-0.951056516295153)) ;
#67725=DIRECTION('',(0.,-1.,0.)) ;
#67726=DIRECTION('',(-0.309016994374948,0.,0.951056516295153)) ;
#67727=DIRECTION('center_axis',(0.,-1.,0.)) ;
#67728=DIRECTION('ref_axis',(-1.,0.,0.)) ;
#67729=DIRECTION('',(0.,1.,0.)) ;
#67730=DIRECTION('center_axis',(0.,1.,0.)) ;
#67731=DIRECTION('ref_axis',(0.156434465040232,0.,-0.987688340595138)) ;
#67732=DIRECTION('center_axis',(1.,0.,0.)) ;
#67733=DIRECTION('ref_axis',(0.,0.,1.)) ;
#67734=DIRECTION('',(0.,-1.,0.)) ;
#67735=DIRECTION('',(0.,0.,-1.)) ;
#67736=DIRECTION('center_axis',(0.,-1.,0.)) ;
#67737=DIRECTION('ref_axis',(-4.50212443845799E-15,0.,-1.)) ;
#67738=DIRECTION('',(0.,-1.,0.)) ;
#67739=DIRECTION('center_axis',(0.,1.,0.)) ;
#67740=DIRECTION('ref_axis',(0.,0.,-1.)) ;
#67741=DIRECTION('center_axis',(-1.,0.,0.)) ;
#67742=DIRECTION('ref_axis',(0.,0.,-1.)) ;
#67743=DIRECTION('',(0.,-1.,0.)) ;
#67744=DIRECTION('',(0.,0.,1.)) ;
#67745=DIRECTION('center_axis',(0.,-1.,0.)) ;
#67746=DIRECTION('ref_axis',(-1.,0.,0.)) ;
#67747=DIRECTION('',(0.,1.,0.)) ;
#67748=DIRECTION('center_axis',(0.,1.,0.)) ;
#67749=DIRECTION('ref_axis',(-0.15643446504023,0.,-0.987688340595138)) ;
#67750=DIRECTION('center_axis',(0.951056516295154,0.,-0.309016994374947)) ;
#67751=DIRECTION('ref_axis',(0.309016994374947,0.,0.951056516295154)) ;
#67752=DIRECTION('',(0.,-1.,0.)) ;
#67753=DIRECTION('',(-0.309016994374947,0.,-0.951056516295154)) ;
#67754=DIRECTION('center_axis',(0.,-1.,0.)) ;
#67755=DIRECTION('ref_axis',(-0.309016994374953,0.,-0.951056516295152)) ;
#67756=DIRECTION('',(0.,-1.,0.)) ;
#67757=DIRECTION('center_axis',(0.,1.,0.)) ;
#67758=DIRECTION('ref_axis',(-0.309016994374945,0.,-0.951056516295154)) ;
#67759=DIRECTION('center_axis',(-0.951056516295154,0.,0.309016994374947)) ;
#67760=DIRECTION('ref_axis',(-0.309016994374947,0.,-0.951056516295154)) ;
#67761=DIRECTION('',(0.,-1.,0.)) ;
#67762=DIRECTION('',(0.309016994374947,0.,0.951056516295154)) ;
#67763=DIRECTION('center_axis',(0.,-1.,0.)) ;
#67764=DIRECTION('ref_axis',(-1.,0.,0.)) ;
#67765=DIRECTION('',(0.,1.,0.)) ;
#67766=DIRECTION('center_axis',(0.,1.,0.)) ;
#67767=DIRECTION('ref_axis',(-0.453990499739546,0.,-0.891006524188368)) ;
#67768=DIRECTION('center_axis',(0.809016994374948,0.,-0.587785252292473)) ;
#67769=DIRECTION('ref_axis',(0.587785252292473,0.,0.809016994374948)) ;
#67770=DIRECTION('',(0.,-1.,0.)) ;
#67771=DIRECTION('',(-0.587785252292473,0.,-0.809016994374947)) ;
#67772=DIRECTION('center_axis',(0.,-1.,0.)) ;
#67773=DIRECTION('ref_axis',(-0.587785252292477,0.,-0.809016994374945)) ;
#67774=DIRECTION('',(0.,-1.,0.)) ;
#67775=DIRECTION('center_axis',(0.,1.,0.)) ;
#67776=DIRECTION('ref_axis',(-0.587785252292474,0.,-0.809016994374947)) ;
#67777=DIRECTION('center_axis',(-0.809016994374948,0.,0.587785252292473)) ;
#67778=DIRECTION('ref_axis',(-0.587785252292473,0.,-0.809016994374948)) ;
#67779=DIRECTION('',(0.,-1.,0.)) ;
#67780=DIRECTION('',(0.587785252292473,0.,0.809016994374947)) ;
#67781=DIRECTION('center_axis',(0.,-1.,0.)) ;
#67782=DIRECTION('ref_axis',(-1.,0.,0.)) ;
#67783=DIRECTION('',(0.,1.,0.)) ;
#67784=DIRECTION('center_axis',(0.,1.,0.)) ;
#67785=DIRECTION('ref_axis',(-0.707106781186547,0.,-0.707106781186548)) ;
#67786=DIRECTION('center_axis',(0.587785252292473,0.,-0.809016994374947)) ;
#67787=DIRECTION('ref_axis',(0.809016994374947,0.,0.587785252292473)) ;
#67788=DIRECTION('',(0.,-1.,0.)) ;
#67789=DIRECTION('',(-0.809016994374947,0.,-0.587785252292473)) ;
#67790=DIRECTION('center_axis',(0.,-1.,0.)) ;
#67791=DIRECTION('ref_axis',(-0.809016994374942,0.,-0.587785252292481)) ;
#67792=DIRECTION('',(0.,-1.,0.)) ;
#67793=DIRECTION('center_axis',(0.,1.,0.)) ;
#67794=DIRECTION('ref_axis',(-0.809016994374947,0.,-0.587785252292474)) ;
#67795=DIRECTION('center_axis',(-0.587785252292473,0.,0.809016994374947)) ;
#67796=DIRECTION('ref_axis',(-0.809016994374947,0.,-0.587785252292473)) ;
#67797=DIRECTION('',(0.,-1.,0.)) ;
#67798=DIRECTION('',(0.809016994374947,0.,0.587785252292473)) ;
#67799=DIRECTION('center_axis',(0.,-1.,0.)) ;
#67800=DIRECTION('ref_axis',(-1.,0.,0.)) ;
#67801=DIRECTION('',(0.,1.,0.)) ;
#67802=DIRECTION('center_axis',(0.,1.,0.)) ;
#67803=DIRECTION('ref_axis',(-0.891006524188368,0.,-0.453990499739547)) ;
#67804=DIRECTION('center_axis',(0.309016994374948,0.,-0.951056516295154)) ;
#67805=DIRECTION('ref_axis',(0.951056516295154,0.,0.309016994374948)) ;
#67806=DIRECTION('',(0.,-1.,0.)) ;
#67807=DIRECTION('',(-0.951056516295154,0.,-0.309016994374948)) ;
#67808=DIRECTION('center_axis',(0.,-1.,0.)) ;
#67809=DIRECTION('ref_axis',(-0.951056516295152,0.,-0.309016994374953)) ;
#67810=DIRECTION('',(0.,-1.,0.)) ;
#67811=DIRECTION('center_axis',(0.,1.,0.)) ;
#67812=DIRECTION('ref_axis',(-0.951056516295154,0.,-0.309016994374945)) ;
#67813=DIRECTION('center_axis',(-0.309016994374948,0.,0.951056516295154)) ;
#67814=DIRECTION('ref_axis',(-0.951056516295154,0.,-0.309016994374948)) ;
#67815=DIRECTION('',(0.,-1.,0.)) ;
#67816=DIRECTION('',(0.951056516295154,0.,0.309016994374948)) ;
#67817=DIRECTION('center_axis',(0.,-1.,0.)) ;
#67818=DIRECTION('ref_axis',(-1.,0.,0.)) ;
#67819=DIRECTION('',(0.,1.,0.)) ;
#67820=DIRECTION('center_axis',(0.,1.,0.)) ;
#67821=DIRECTION('ref_axis',(-0.987688340595138,0.,-0.156434465040231)) ;
#67822=DIRECTION('center_axis',(5.55111512312578E-17,0.,-1.)) ;
#67823=DIRECTION('ref_axis',(1.,0.,5.55111512312578E-17)) ;
#67824=DIRECTION('',(0.,-1.,0.)) ;
#67825=DIRECTION('',(-1.,0.,-5.55111512312578E-17)) ;
#67826=DIRECTION('center_axis',(0.,-1.,0.)) ;
#67827=DIRECTION('ref_axis',(-1.,0.,9.31771680776961E-15)) ;
#67828=DIRECTION('',(0.,-1.,0.)) ;
#67829=DIRECTION('center_axis',(0.,1.,0.)) ;
#67830=DIRECTION('ref_axis',(-1.,0.,0.)) ;
#67831=DIRECTION('center_axis',(-5.55111512312578E-17,0.,1.)) ;
#67832=DIRECTION('ref_axis',(-1.,0.,-5.55111512312578E-17)) ;
#67833=DIRECTION('',(0.,-1.,0.)) ;
#67834=DIRECTION('',(1.,0.,5.55111512312578E-17)) ;
#67835=DIRECTION('center_axis',(0.,-1.,0.)) ;
#67836=DIRECTION('ref_axis',(-1.,0.,0.)) ;
#67837=DIRECTION('',(0.,1.,0.)) ;
#67838=DIRECTION('center_axis',(0.,1.,0.)) ;
#67839=DIRECTION('ref_axis',(-0.987688340595138,0.,0.156434465040229)) ;
#67840=DIRECTION('center_axis',(-0.309016994374947,0.,-0.951056516295154)) ;
#67841=DIRECTION('ref_axis',(0.951056516295154,0.,-0.309016994374947)) ;
#67842=DIRECTION('',(0.,-1.,0.)) ;
#67843=DIRECTION('',(-0.951056516295154,0.,0.309016994374947)) ;
#67844=DIRECTION('center_axis',(0.,-1.,0.)) ;
#67845=DIRECTION('ref_axis',(-0.951056516295152,0.,0.309016994374954)) ;
#67846=DIRECTION('',(0.,-1.,0.)) ;
#67847=DIRECTION('center_axis',(0.,1.,0.)) ;
#67848=DIRECTION('ref_axis',(-0.951056516295154,0.,0.309016994374945)) ;
#67849=DIRECTION('center_axis',(0.309016994374947,0.,0.951056516295154)) ;
#67850=DIRECTION('ref_axis',(-0.951056516295154,0.,0.309016994374947)) ;
#67851=DIRECTION('',(0.,-1.,0.)) ;
#67852=DIRECTION('',(0.951056516295154,0.,-0.309016994374947)) ;
#67853=DIRECTION('center_axis',(0.,-1.,0.)) ;
#67854=DIRECTION('ref_axis',(-1.,0.,0.)) ;
#67855=DIRECTION('',(0.,1.,0.)) ;
#67856=DIRECTION('center_axis',(0.,1.,0.)) ;
#67857=DIRECTION('ref_axis',(-0.891006524188369,0.,0.453990499739545)) ;
#67858=DIRECTION('center_axis',(-0.587785252292473,0.,-0.809016994374948)) ;
#67859=DIRECTION('ref_axis',(0.809016994374948,0.,-0.587785252292473)) ;
#67860=DIRECTION('',(0.,-1.,0.)) ;
#67861=DIRECTION('',(-0.809016994374947,0.,0.587785252292473)) ;
#67862=DIRECTION('center_axis',(0.,-1.,0.)) ;
#67863=DIRECTION('ref_axis',(-0.809016994374949,0.,0.587785252292471)) ;
#67864=DIRECTION('',(0.,-1.,0.)) ;
#67865=DIRECTION('center_axis',(0.,1.,0.)) ;
#67866=DIRECTION('ref_axis',(-0.809016994374947,0.,0.587785252292474)) ;
#67867=DIRECTION('center_axis',(0.587785252292473,0.,0.809016994374948)) ;
#67868=DIRECTION('ref_axis',(-0.809016994374948,0.,0.587785252292473)) ;
#67869=DIRECTION('',(0.,-1.,0.)) ;
#67870=DIRECTION('',(0.809016994374947,0.,-0.587785252292473)) ;
#67871=DIRECTION('center_axis',(0.,-1.,0.)) ;
#67872=DIRECTION('ref_axis',(-1.,0.,0.)) ;
#67873=DIRECTION('',(0.,1.,0.)) ;
#67874=DIRECTION('center_axis',(0.,1.,0.)) ;
#67875=DIRECTION('ref_axis',(-0.707106781186548,0.,0.707106781186547)) ;
#67876=DIRECTION('center_axis',(-0.809016994374947,0.,-0.587785252292473)) ;
#67877=DIRECTION('ref_axis',(0.587785252292473,0.,-0.809016994374947)) ;
#67878=DIRECTION('',(0.,-1.,0.)) ;
#67879=DIRECTION('',(-0.587785252292473,0.,0.809016994374947)) ;
#67880=DIRECTION('center_axis',(0.,-1.,0.)) ;
#67881=DIRECTION('ref_axis',(-0.587785252292476,0.,0.809016994374946)) ;
#67882=DIRECTION('',(0.,-1.,0.)) ;
#67883=DIRECTION('center_axis',(0.,1.,0.)) ;
#67884=DIRECTION('ref_axis',(-0.587785252292474,0.,0.809016994374947)) ;
#67885=DIRECTION('center_axis',(0.809016994374947,0.,0.587785252292473)) ;
#67886=DIRECTION('ref_axis',(-0.587785252292473,0.,0.809016994374947)) ;
#67887=DIRECTION('',(0.,-1.,0.)) ;
#67888=DIRECTION('',(0.587785252292473,0.,-0.809016994374947)) ;
#67889=DIRECTION('center_axis',(0.,-1.,0.)) ;
#67890=DIRECTION('ref_axis',(-1.,0.,0.)) ;
#67891=DIRECTION('',(0.,1.,0.)) ;
#67892=DIRECTION('center_axis',(0.,1.,0.)) ;
#67893=DIRECTION('ref_axis',(-0.453990499739546,0.,0.891006524188368)) ;
#67894=DIRECTION('center_axis',(0.,1.,0.)) ;
#67895=DIRECTION('ref_axis',(-1.,0.,0.)) ;
#67896=DIRECTION('center_axis',(0.,-1.,0.)) ;
#67897=DIRECTION('ref_axis',(-0.406305370818768,0.,0.913737350469939)) ;
#67898=DIRECTION('center_axis',(0.,1.,0.)) ;
#67899=DIRECTION('ref_axis',(-1.,0.,0.)) ;
#67900=DIRECTION('center_axis',(0.,-1.,0.)) ;
#67901=DIRECTION('ref_axis',(-0.406305370818768,0.,0.913737350469939)) ;
#67902=DIRECTION('center_axis',(0.,1.,0.)) ;
#67903=DIRECTION('ref_axis',(-1.,0.,0.)) ;
#67904=DIRECTION('center_axis',(0.,-1.,0.)) ;
#67905=DIRECTION('ref_axis',(-0.406305370818768,0.,0.913737350469939)) ;
#67906=DIRECTION('center_axis',(0.,1.,0.)) ;
#67907=DIRECTION('ref_axis',(-1.,0.,0.)) ;
#67908=DIRECTION('center_axis',(0.,-1.,0.)) ;
#67909=DIRECTION('ref_axis',(-0.406305370818768,0.,0.913737350469939)) ;
#67910=DIRECTION('center_axis',(0.,1.,0.)) ;
#67911=DIRECTION('ref_axis',(-1.,0.,0.)) ;
#67912=DIRECTION('center_axis',(0.,-1.,0.)) ;
#67913=DIRECTION('ref_axis',(-0.406305370818768,0.,0.913737350469939)) ;
#67914=DIRECTION('center_axis',(0.,1.,0.)) ;
#67915=DIRECTION('ref_axis',(-1.,0.,0.)) ;
#67916=DIRECTION('center_axis',(0.,-1.,0.)) ;
#67917=DIRECTION('ref_axis',(-0.406305370818768,0.,0.913737350469939)) ;
#67918=DIRECTION('center_axis',(0.,1.,0.)) ;
#67919=DIRECTION('ref_axis',(-1.,0.,0.)) ;
#67920=DIRECTION('center_axis',(0.,-1.,0.)) ;
#67921=DIRECTION('ref_axis',(-0.406305370818768,0.,0.913737350469939)) ;
#67922=DIRECTION('center_axis',(0.,1.,0.)) ;
#67923=DIRECTION('ref_axis',(-1.,0.,0.)) ;
#67924=DIRECTION('center_axis',(0.,-1.,0.)) ;
#67925=DIRECTION('ref_axis',(-0.406305370818768,0.,0.913737350469939)) ;
#67926=DIRECTION('center_axis',(0.,1.,0.)) ;
#67927=DIRECTION('ref_axis',(-1.,0.,0.)) ;
#67928=DIRECTION('center_axis',(0.,-1.,0.)) ;
#67929=DIRECTION('ref_axis',(-0.406305370818768,0.,0.913737350469939)) ;
#67930=DIRECTION('center_axis',(0.,1.,0.)) ;
#67931=DIRECTION('ref_axis',(-1.,0.,0.)) ;
#67932=DIRECTION('center_axis',(0.,-1.,0.)) ;
#67933=DIRECTION('ref_axis',(-0.406305370818768,0.,0.913737350469939)) ;
#67934=DIRECTION('center_axis',(0.,1.,0.)) ;
#67935=DIRECTION('ref_axis',(-1.,0.,0.)) ;
#67936=DIRECTION('center_axis',(0.,-1.,0.)) ;
#67937=DIRECTION('ref_axis',(-0.406305370818768,0.,0.913737350469939)) ;
#67938=DIRECTION('center_axis',(0.,1.,0.)) ;
#67939=DIRECTION('ref_axis',(-1.,0.,0.)) ;
#67940=DIRECTION('center_axis',(0.,-1.,0.)) ;
#67941=DIRECTION('ref_axis',(-0.406305370818768,0.,0.913737350469939)) ;
#67942=DIRECTION('center_axis',(0.,1.,0.)) ;
#67943=DIRECTION('ref_axis',(-1.,0.,0.)) ;
#67944=DIRECTION('center_axis',(0.,-1.,0.)) ;
#67945=DIRECTION('ref_axis',(-0.406305370818768,0.,0.913737350469939)) ;
#67946=DIRECTION('center_axis',(0.,1.,0.)) ;
#67947=DIRECTION('ref_axis',(-1.,0.,0.)) ;
#67948=DIRECTION('center_axis',(0.,-1.,0.)) ;
#67949=DIRECTION('ref_axis',(-0.406305370818768,0.,0.913737350469939)) ;
#67950=DIRECTION('center_axis',(0.,1.,0.)) ;
#67951=DIRECTION('ref_axis',(-1.,0.,0.)) ;
#67952=DIRECTION('center_axis',(0.,-1.,0.)) ;
#67953=DIRECTION('ref_axis',(-0.406305370818768,0.,0.913737350469939)) ;
#67954=DIRECTION('center_axis',(0.,1.,0.)) ;
#67955=DIRECTION('ref_axis',(-1.,0.,0.)) ;
#67956=DIRECTION('center_axis',(0.,-1.,0.)) ;
#67957=DIRECTION('ref_axis',(-0.406305370818768,0.,0.913737350469939)) ;
#67958=DIRECTION('center_axis',(0.,1.,0.)) ;
#67959=DIRECTION('ref_axis',(-1.,0.,0.)) ;
#67960=DIRECTION('center_axis',(0.,-1.,0.)) ;
#67961=DIRECTION('ref_axis',(-0.406305370818768,0.,0.913737350469939)) ;
#67962=DIRECTION('center_axis',(0.,1.,0.)) ;
#67963=DIRECTION('ref_axis',(-1.,0.,0.)) ;
#67964=DIRECTION('center_axis',(0.,-1.,0.)) ;
#67965=DIRECTION('ref_axis',(-0.406305370818768,0.,0.913737350469939)) ;
#67966=DIRECTION('center_axis',(0.,1.,0.)) ;
#67967=DIRECTION('ref_axis',(-1.,0.,0.)) ;
#67968=DIRECTION('center_axis',(0.,-1.,0.)) ;
#67969=DIRECTION('ref_axis',(-0.406305370818768,0.,0.913737350469939)) ;
#67970=DIRECTION('center_axis',(0.,-1.,0.)) ;
#67971=DIRECTION('ref_axis',(-0.406305370818768,0.,0.913737350469939)) ;
#67972=DIRECTION('center_axis',(0.,-1.,0.)) ;
#67973=DIRECTION('ref_axis',(0.,0.,-1.)) ;
#67974=DIRECTION('center_axis',(1.,0.,0.)) ;
#67975=DIRECTION('ref_axis',(0.,0.,1.)) ;
#67976=DIRECTION('center_axis',(0.,-1.,0.)) ;
#67977=DIRECTION('ref_axis',(-0.406305370818768,0.,0.913737350469939)) ;
#67978=DIRECTION('center_axis',(0.,1.,0.)) ;
#67979=DIRECTION('ref_axis',(-1.,0.,0.)) ;
#67980=DIRECTION('center_axis',(0.,1.,0.)) ;
#67981=DIRECTION('ref_axis',(0.,0.,1.)) ;
#67982=DIRECTION('center_axis',(1.,0.,0.)) ;
#67983=DIRECTION('ref_axis',(0.,0.,-1.)) ;
#67984=DIRECTION('center_axis',(0.,1.,0.)) ;
#67985=DIRECTION('ref_axis',(-0.208373389176835,0.,0.978049349819813)) ;
#67986=DIRECTION('center_axis',(0.,-1.,0.)) ;
#67987=DIRECTION('ref_axis',(-0.15643446504023,0.,-0.987688340595138)) ;
#67988=DIRECTION('center_axis',(0.,1.,0.)) ;
#67989=DIRECTION('ref_axis',(-0.208373389176835,0.,0.978049349819813)) ;
#67990=DIRECTION('center_axis',(0.,-1.,0.)) ;
#67991=DIRECTION('ref_axis',(-0.453990499739546,0.,-0.891006524188368)) ;
#67992=DIRECTION('center_axis',(0.,1.,0.)) ;
#67993=DIRECTION('ref_axis',(-0.208373389176835,0.,0.978049349819813)) ;
#67994=DIRECTION('center_axis',(0.,-1.,0.)) ;
#67995=DIRECTION('ref_axis',(-0.707106781186547,0.,-0.707106781186548)) ;
#67996=DIRECTION('center_axis',(0.,1.,0.)) ;
#67997=DIRECTION('ref_axis',(-0.208373389176835,0.,0.978049349819813)) ;
#67998=DIRECTION('center_axis',(0.,-1.,0.)) ;
#67999=DIRECTION('ref_axis',(-0.891006524188368,0.,-0.453990499739547)) ;
#68000=DIRECTION('center_axis',(0.,1.,0.)) ;
#68001=DIRECTION('ref_axis',(-0.208373389176835,0.,0.978049349819813)) ;
#68002=DIRECTION('center_axis',(0.,-1.,0.)) ;
#68003=DIRECTION('ref_axis',(-0.987688340595138,0.,-0.156434465040231)) ;
#68004=DIRECTION('center_axis',(0.,1.,0.)) ;
#68005=DIRECTION('ref_axis',(-0.208373389176835,0.,0.978049349819813)) ;
#68006=DIRECTION('center_axis',(0.,-1.,0.)) ;
#68007=DIRECTION('ref_axis',(-0.987688340595138,0.,0.156434465040229)) ;
#68008=DIRECTION('center_axis',(0.,1.,0.)) ;
#68009=DIRECTION('ref_axis',(-0.208373389176835,0.,0.978049349819813)) ;
#68010=DIRECTION('center_axis',(0.,-1.,0.)) ;
#68011=DIRECTION('ref_axis',(-0.891006524188369,0.,0.453990499739545)) ;
#68012=DIRECTION('center_axis',(0.,1.,0.)) ;
#68013=DIRECTION('ref_axis',(-0.208373389176835,0.,0.978049349819813)) ;
#68014=DIRECTION('center_axis',(0.,-1.,0.)) ;
#68015=DIRECTION('ref_axis',(-0.707106781186548,0.,0.707106781186547)) ;
#68016=DIRECTION('center_axis',(0.,1.,0.)) ;
#68017=DIRECTION('ref_axis',(-0.208373389176835,0.,0.978049349819813)) ;
#68018=DIRECTION('center_axis',(0.,-1.,0.)) ;
#68019=DIRECTION('ref_axis',(-0.453990499739546,0.,0.891006524188368)) ;
#68020=DIRECTION('center_axis',(0.,1.,0.)) ;
#68021=DIRECTION('ref_axis',(-0.208373389176835,0.,0.978049349819813)) ;
#68022=DIRECTION('center_axis',(0.,-1.,0.)) ;
#68023=DIRECTION('ref_axis',(-0.156434465040232,0.,0.987688340595138)) ;
#68024=DIRECTION('center_axis',(0.,1.,0.)) ;
#68025=DIRECTION('ref_axis',(-0.208373389176835,0.,0.978049349819813)) ;
#68026=DIRECTION('center_axis',(0.,-1.,0.)) ;
#68027=DIRECTION('ref_axis',(0.156434465040233,0.,0.987688340595137)) ;
#68028=DIRECTION('center_axis',(0.,1.,0.)) ;
#68029=DIRECTION('ref_axis',(-0.208373389176835,0.,0.978049349819813)) ;
#68030=DIRECTION('center_axis',(0.,-1.,0.)) ;
#68031=DIRECTION('ref_axis',(0.453990499739549,0.,0.891006524188367)) ;
#68032=DIRECTION('center_axis',(0.,1.,0.)) ;
#68033=DIRECTION('ref_axis',(-0.208373389176835,0.,0.978049349819813)) ;
#68034=DIRECTION('center_axis',(0.,-1.,0.)) ;
#68035=DIRECTION('ref_axis',(0.707106781186548,0.,0.707106781186547)) ;
#68036=DIRECTION('center_axis',(0.,1.,0.)) ;
#68037=DIRECTION('ref_axis',(-0.208373389176835,0.,0.978049349819813)) ;
#68038=DIRECTION('center_axis',(0.,-1.,0.)) ;
#68039=DIRECTION('ref_axis',(0.891006524188368,0.,0.453990499739546)) ;
#68040=DIRECTION('center_axis',(0.,1.,0.)) ;
#68041=DIRECTION('ref_axis',(-0.208373389176835,0.,0.978049349819813)) ;
#68042=DIRECTION('center_axis',(0.,-1.,0.)) ;
#68043=DIRECTION('ref_axis',(0.987688340595138,0.,0.156434465040232)) ;
#68044=DIRECTION('center_axis',(0.,1.,0.)) ;
#68045=DIRECTION('ref_axis',(-0.208373389176835,0.,0.978049349819813)) ;
#68046=DIRECTION('center_axis',(0.,-1.,0.)) ;
#68047=DIRECTION('ref_axis',(0.987688340595138,0.,-0.156434465040228)) ;
#68048=DIRECTION('center_axis',(0.,1.,0.)) ;
#68049=DIRECTION('ref_axis',(-0.208373389176835,0.,0.978049349819813)) ;
#68050=DIRECTION('center_axis',(0.,-1.,0.)) ;
#68051=DIRECTION('ref_axis',(0.891006524188368,0.,-0.453990499739547)) ;
#68052=DIRECTION('center_axis',(0.,1.,0.)) ;
#68053=DIRECTION('ref_axis',(-0.208373389176835,0.,0.978049349819813)) ;
#68054=DIRECTION('center_axis',(0.,-1.,0.)) ;
#68055=DIRECTION('ref_axis',(0.707106781186547,0.,-0.707106781186547)) ;
#68056=DIRECTION('center_axis',(0.,1.,0.)) ;
#68057=DIRECTION('ref_axis',(-0.208373389176835,0.,0.978049349819813)) ;
#68058=DIRECTION('center_axis',(0.,-1.,0.)) ;
#68059=DIRECTION('ref_axis',(0.453990499739547,0.,-0.891006524188368)) ;
#68060=DIRECTION('center_axis',(0.,1.,0.)) ;
#68061=DIRECTION('ref_axis',(-0.208373389176835,0.,0.978049349819813)) ;
#68062=DIRECTION('center_axis',(0.,-1.,0.)) ;
#68063=DIRECTION('ref_axis',(0.156434465040232,0.,-0.987688340595138)) ;
#68064=DIRECTION('center_axis',(0.,1.,0.)) ;
#68065=DIRECTION('ref_axis',(-0.208373389176835,0.,0.978049349819813)) ;
#68066=DIRECTION('center_axis',(0.,1.,0.)) ;
#68067=DIRECTION('ref_axis',(-1.,0.,0.)) ;
#68068=DIRECTION('',(-0.309016994374948,0.,0.951056516295153)) ;
#68069=DIRECTION('center_axis',(0.,-1.,0.)) ;
#68070=DIRECTION('ref_axis',(0.309016994374945,0.,-0.951056516295154)) ;
#68071=DIRECTION('',(0.309016994374948,0.,-0.951056516295153)) ;
#68072=DIRECTION('center_axis',(0.,1.,0.)) ;
#68073=DIRECTION('ref_axis',(-1.,0.,0.)) ;
#68074=DIRECTION('',(-0.587785252292473,0.,0.809016994374947)) ;
#68075=DIRECTION('center_axis',(0.,-1.,0.)) ;
#68076=DIRECTION('ref_axis',(0.587785252292468,0.,-0.809016994374951)) ;
#68077=DIRECTION('',(0.587785252292473,0.,-0.809016994374947)) ;
#68078=DIRECTION('center_axis',(0.,1.,0.)) ;
#68079=DIRECTION('ref_axis',(-1.,0.,0.)) ;
#68080=DIRECTION('',(-0.809016994374948,0.,0.587785252292473)) ;
#68081=DIRECTION('center_axis',(0.,-1.,0.)) ;
#68082=DIRECTION('ref_axis',(0.809016994374947,0.,-0.587785252292474)) ;
#68083=DIRECTION('',(0.809016994374948,0.,-0.587785252292473)) ;
#68084=DIRECTION('center_axis',(0.,1.,0.)) ;
#68085=DIRECTION('ref_axis',(-1.,0.,0.)) ;
#68086=DIRECTION('',(-0.951056516295154,0.,0.309016994374947)) ;
#68087=DIRECTION('center_axis',(0.,-1.,0.)) ;
#68088=DIRECTION('ref_axis',(0.951056516295153,0.,-0.309016994374948)) ;
#68089=DIRECTION('',(0.951056516295154,0.,-0.309016994374947)) ;
#68090=DIRECTION('center_axis',(0.,1.,0.)) ;
#68091=DIRECTION('ref_axis',(-1.,0.,0.)) ;
#68092=DIRECTION('',(-1.,0.,-2.22044604925031E-16)) ;
#68093=DIRECTION('center_axis',(0.,-1.,0.)) ;
#68094=DIRECTION('ref_axis',(1.,0.,0.)) ;
#68095=DIRECTION('',(1.,0.,2.22044604925031E-16)) ;
#68096=DIRECTION('center_axis',(0.,1.,0.)) ;
#68097=DIRECTION('ref_axis',(-1.,0.,0.)) ;
#68098=DIRECTION('',(-0.951056516295153,0.,-0.309016994374948)) ;
#68099=DIRECTION('center_axis',(0.,-1.,0.)) ;
#68100=DIRECTION('ref_axis',(0.951056516295153,0.,0.309016994374948)) ;
#68101=DIRECTION('',(0.951056516295153,0.,0.309016994374948)) ;
#68102=DIRECTION('center_axis',(0.,1.,0.)) ;
#68103=DIRECTION('ref_axis',(-1.,0.,0.)) ;
#68104=DIRECTION('',(-0.809016994374947,0.,-0.587785252292473)) ;
#68105=DIRECTION('center_axis',(0.,-1.,0.)) ;
#68106=DIRECTION('ref_axis',(0.809016994374947,0.,0.587785252292474)) ;
#68107=DIRECTION('',(0.809016994374947,0.,0.587785252292473)) ;
#68108=DIRECTION('center_axis',(0.,1.,0.)) ;
#68109=DIRECTION('ref_axis',(-1.,0.,0.)) ;
#68110=DIRECTION('',(-0.587785252292473,0.,-0.809016994374947)) ;
#68111=DIRECTION('center_axis',(0.,-1.,0.)) ;
#68112=DIRECTION('ref_axis',(0.587785252292468,0.,0.809016994374951)) ;
#68113=DIRECTION('',(0.587785252292473,0.,0.809016994374947)) ;
#68114=DIRECTION('center_axis',(0.,1.,0.)) ;
#68115=DIRECTION('ref_axis',(-1.,0.,0.)) ;
#68116=DIRECTION('',(-0.309016994374947,0.,-0.951056516295154)) ;
#68117=DIRECTION('center_axis',(0.,-1.,0.)) ;
#68118=DIRECTION('ref_axis',(0.309016994374945,0.,0.951056516295154)) ;
#68119=DIRECTION('',(0.309016994374947,0.,0.951056516295154)) ;
#68120=DIRECTION('center_axis',(0.,1.,0.)) ;
#68121=DIRECTION('ref_axis',(-1.,0.,0.)) ;
#68122=DIRECTION('',(1.11022302462516E-16,0.,-1.)) ;
#68123=DIRECTION('center_axis',(0.,-1.,0.)) ;
#68124=DIRECTION('ref_axis',(0.,0.,1.)) ;
#68125=DIRECTION('',(-1.11022302462516E-16,0.,1.)) ;
#68126=DIRECTION('center_axis',(0.,1.,0.)) ;
#68127=DIRECTION('ref_axis',(-1.,0.,0.)) ;
#68128=DIRECTION('',(0.309016994374948,0.,-0.951056516295154)) ;
#68129=DIRECTION('center_axis',(0.,-1.,0.)) ;
#68130=DIRECTION('ref_axis',(-0.309016994374945,0.,0.951056516295154)) ;
#68131=DIRECTION('',(-0.309016994374948,0.,0.951056516295154)) ;
#68132=DIRECTION('center_axis',(0.,1.,0.)) ;
#68133=DIRECTION('ref_axis',(-1.,0.,0.)) ;
#68134=DIRECTION('',(0.587785252292473,0.,-0.809016994374947)) ;
#68135=DIRECTION('center_axis',(0.,-1.,0.)) ;
#68136=DIRECTION('ref_axis',(-0.587785252292474,0.,0.809016994374947)) ;
#68137=DIRECTION('',(-0.587785252292473,0.,0.809016994374947)) ;
#68138=DIRECTION('center_axis',(0.,1.,0.)) ;
#68139=DIRECTION('ref_axis',(-1.,0.,0.)) ;
#68140=DIRECTION('',(0.809016994374947,0.,-0.587785252292473)) ;
#68141=DIRECTION('center_axis',(0.,-1.,0.)) ;
#68142=DIRECTION('ref_axis',(-0.809016994374947,0.,0.587785252292474)) ;
#68143=DIRECTION('',(-0.809016994374947,0.,0.587785252292473)) ;
#68144=DIRECTION('center_axis',(0.,1.,0.)) ;
#68145=DIRECTION('ref_axis',(-1.,0.,0.)) ;
#68146=DIRECTION('',(0.951056516295154,0.,-0.309016994374947)) ;
#68147=DIRECTION('center_axis',(0.,-1.,0.)) ;
#68148=DIRECTION('ref_axis',(-0.951056516295154,0.,0.309016994374945)) ;
#68149=DIRECTION('',(-0.951056516295154,0.,0.309016994374947)) ;
#68150=DIRECTION('center_axis',(0.,1.,0.)) ;
#68151=DIRECTION('ref_axis',(-1.,0.,0.)) ;
#68152=DIRECTION('',(1.,0.,5.55111512312578E-17)) ;
#68153=DIRECTION('center_axis',(0.,-1.,0.)) ;
#68154=DIRECTION('ref_axis',(-1.,0.,0.)) ;
#68155=DIRECTION('',(-1.,0.,-5.55111512312578E-17)) ;
#68156=DIRECTION('center_axis',(0.,1.,0.)) ;
#68157=DIRECTION('ref_axis',(-1.,0.,0.)) ;
#68158=DIRECTION('',(0.951056516295154,0.,0.309016994374948)) ;
#68159=DIRECTION('center_axis',(0.,-1.,0.)) ;
#68160=DIRECTION('ref_axis',(-0.951056516295154,0.,-0.309016994374945)) ;
#68161=DIRECTION('',(-0.951056516295154,0.,-0.309016994374948)) ;
#68162=DIRECTION('center_axis',(0.,1.,0.)) ;
#68163=DIRECTION('ref_axis',(-1.,0.,0.)) ;
#68164=DIRECTION('',(0.809016994374947,0.,0.587785252292473)) ;
#68165=DIRECTION('center_axis',(0.,-1.,0.)) ;
#68166=DIRECTION('ref_axis',(-0.809016994374947,0.,-0.587785252292474)) ;
#68167=DIRECTION('',(-0.809016994374947,0.,-0.587785252292473)) ;
#68168=DIRECTION('center_axis',(0.,1.,0.)) ;
#68169=DIRECTION('ref_axis',(-1.,0.,0.)) ;
#68170=DIRECTION('',(0.587785252292473,0.,0.809016994374947)) ;
#68171=DIRECTION('center_axis',(0.,-1.,0.)) ;
#68172=DIRECTION('ref_axis',(-0.587785252292474,0.,-0.809016994374947)) ;
#68173=DIRECTION('',(-0.587785252292473,0.,-0.809016994374947)) ;
#68174=DIRECTION('center_axis',(0.,1.,0.)) ;
#68175=DIRECTION('ref_axis',(-1.,0.,0.)) ;
#68176=DIRECTION('',(0.309016994374947,0.,0.951056516295154)) ;
#68177=DIRECTION('center_axis',(0.,-1.,0.)) ;
#68178=DIRECTION('ref_axis',(-0.309016994374945,0.,-0.951056516295154)) ;
#68179=DIRECTION('',(-0.309016994374947,0.,-0.951056516295154)) ;
#68180=DIRECTION('center_axis',(0.,1.,0.)) ;
#68181=DIRECTION('ref_axis',(-1.,0.,0.)) ;
#68182=DIRECTION('',(0.,0.,1.)) ;
#68183=DIRECTION('center_axis',(0.,-1.,0.)) ;
#68184=DIRECTION('ref_axis',(0.,0.,-1.)) ;
#68185=DIRECTION('',(0.,0.,-1.)) ;
#68186=DIRECTION('center_axis',(0.,1.,0.)) ;
#68187=DIRECTION('ref_axis',(0.,0.,1.)) ;
#68188=DIRECTION('center_axis',(0.,1.,0.)) ;
#68189=DIRECTION('ref_axis',(-0.156434465040232,0.,0.987688340595138)) ;
#68190=DIRECTION('center_axis',(0.309016994374948,0.,-0.951056516295154)) ;
#68191=DIRECTION('ref_axis',(0.672498511963948,0.707106781186557,0.218508012224408)) ;
#68192=DIRECTION('',(0.309016994374948,0.,-0.951056516295154)) ;
#68193=DIRECTION('center_axis',(1.11022302462516E-16,0.,-1.)) ;
#68194=DIRECTION('ref_axis',(-0.707106781186547,0.707106781186547,-7.8504622934189E-17)) ;
#68195=DIRECTION('',(-1.11022302462516E-16,0.,1.)) ;
#68196=DIRECTION('center_axis',(0.309016994374948,0.,-0.951056516295154)) ;
#68197=DIRECTION('ref_axis',(-0.672498511963948,0.707106781186557,-0.218508012224408)) ;
#68198=DIRECTION('',(-0.309016994374948,0.,0.951056516295154)) ;
#68199=DIRECTION('center_axis',(0.,1.,0.)) ;
#68200=DIRECTION('ref_axis',(0.,0.,1.)) ;
#68201=DIRECTION('center_axis',(0.587785252292473,0.,-0.809016994374947)) ;
#68202=DIRECTION('ref_axis',(0.572061402817672,0.707106781186563,0.415626937777444)) ;
#68203=DIRECTION('center_axis',(-0.309016994374947,0.,-0.951056516295154)) ;
#68204=DIRECTION('ref_axis',(-0.672498511963948,0.707106781186557,0.218508012224407)) ;
#68205=DIRECTION('',(0.309016994374947,0.,0.951056516295154)) ;
#68206=DIRECTION('center_axis',(0.587785252292473,0.,-0.809016994374947)) ;
#68207=DIRECTION('ref_axis',(-0.572061402817681,0.707106781186551,-0.415626937777452)) ;
#68208=DIRECTION('center_axis',(0.,1.,0.)) ;
#68209=DIRECTION('ref_axis',(0.,0.,1.)) ;
#68210=DIRECTION('center_axis',(0.809016994374948,0.,-0.587785252292473)) ;
#68211=DIRECTION('ref_axis',(0.415626937777444,0.707106781186563,0.572061402817672)) ;
#68212=DIRECTION('center_axis',(-0.587785252292473,0.,-0.809016994374948)) ;
#68213=DIRECTION('ref_axis',(-0.572061402817695,0.707106781186534,0.415626937777461)) ;
#68214=DIRECTION('',(0.587785252292473,0.,0.809016994374947)) ;
#68215=DIRECTION('center_axis',(0.809016994374948,0.,-0.587785252292473)) ;
#68216=DIRECTION('ref_axis',(-0.415626937777444,0.707106781186563,-0.572061402817672)) ;
#68217=DIRECTION('center_axis',(0.,1.,0.)) ;
#68218=DIRECTION('ref_axis',(0.,0.,1.)) ;
#68219=DIRECTION('center_axis',(0.951056516295154,0.,-0.309016994374947)) ;
#68220=DIRECTION('ref_axis',(0.218508012224407,0.707106781186557,0.672498511963948)) ;
#68221=DIRECTION('center_axis',(-0.809016994374947,0.,-0.587785252292473)) ;
#68222=DIRECTION('ref_axis',(-0.415626937777452,0.707106781186551,0.572061402817681)) ;
#68223=DIRECTION('',(0.809016994374947,0.,0.587785252292473)) ;
#68224=DIRECTION('center_axis',(0.951056516295154,0.,-0.309016994374947)) ;
#68225=DIRECTION('ref_axis',(-0.218508012224407,0.707106781186557,-0.672498511963948)) ;
#68226=DIRECTION('center_axis',(0.,1.,0.)) ;
#68227=DIRECTION('ref_axis',(0.,0.,1.)) ;
#68228=DIRECTION('center_axis',(1.,0.,5.55111512312578E-17)) ;
#68229=DIRECTION('ref_axis',(-3.92523114670932E-17,0.707106781186568,0.707106781186527)) ;
#68230=DIRECTION('center_axis',(-0.951056516295154,0.,-0.309016994374948)) ;
#68231=DIRECTION('ref_axis',(-0.2185080122244,0.707106781186583,0.672498511963923)) ;
#68232=DIRECTION('',(0.951056516295153,0.,0.309016994374948)) ;
#68233=DIRECTION('center_axis',(1.,0.,5.55111512312578E-17)) ;
#68234=DIRECTION('ref_axis',(3.92523114670932E-17,0.707106781186568,-0.707106781186527)) ;
#68235=DIRECTION('center_axis',(0.,1.,0.)) ;
#68236=DIRECTION('ref_axis',(0.,0.,1.)) ;
#68237=DIRECTION('center_axis',(0.951056516295154,0.,0.309016994374948)) ;
#68238=DIRECTION('ref_axis',(-0.218508012224408,0.707106781186557,0.672498511963948)) ;
#68239=DIRECTION('center_axis',(-1.,0.,-2.22044604925031E-16)) ;
#68240=DIRECTION('ref_axis',(-1.57009245868373E-16,0.707106781186568,0.707106781186527)) ;
#68241=DIRECTION('',(1.,0.,2.22044604925031E-16)) ;
#68242=DIRECTION('center_axis',(0.951056516295154,0.,0.309016994374948)) ;
#68243=DIRECTION('ref_axis',(0.218508012224408,0.707106781186557,-0.672498511963948)) ;
#68244=DIRECTION('center_axis',(0.,1.,0.)) ;
#68245=DIRECTION('ref_axis',(0.,0.,1.)) ;
#68246=DIRECTION('center_axis',(0.809016994374947,0.,0.587785252292473)) ;
#68247=DIRECTION('ref_axis',(-0.415626937777444,0.707106781186563,0.572061402817672)) ;
#68248=DIRECTION('center_axis',(-0.951056516295154,0.,0.309016994374947)) ;
#68249=DIRECTION('ref_axis',(0.218508012224405,0.707106781186563,0.672498511963943)) ;
#68250=DIRECTION('',(0.951056516295154,0.,-0.309016994374947)) ;
#68251=DIRECTION('center_axis',(0.809016994374947,0.,0.587785252292473)) ;
#68252=DIRECTION('ref_axis',(0.415626937777442,0.707106781186568,-0.572061402817668)) ;
#68253=DIRECTION('center_axis',(0.,1.,0.)) ;
#68254=DIRECTION('ref_axis',(0.,0.,1.)) ;
#68255=DIRECTION('center_axis',(0.587785252292473,0.,0.809016994374948)) ;
#68256=DIRECTION('ref_axis',(-0.572061402817672,0.707106781186563,0.415626937777444)) ;
#68257=DIRECTION('center_axis',(-0.809016994374948,0.,0.587785252292473)) ;
#68258=DIRECTION('ref_axis',(0.415626937777451,0.707106781186551,0.572061402817682)) ;
#68259=DIRECTION('',(0.809016994374948,0.,-0.587785252292473)) ;
#68260=DIRECTION('center_axis',(0.587785252292473,0.,0.809016994374948)) ;
#68261=DIRECTION('ref_axis',(0.572061402817682,0.707106781186551,-0.415626937777451)) ;
#68262=DIRECTION('center_axis',(0.,1.,0.)) ;
#68263=DIRECTION('ref_axis',(0.,0.,1.)) ;
#68264=DIRECTION('center_axis',(0.309016994374947,0.,0.951056516295154)) ;
#68265=DIRECTION('ref_axis',(-0.672498511963948,0.707106781186557,0.218508012224407)) ;
#68266=DIRECTION('center_axis',(-0.587785252292473,0.,0.809016994374947)) ;
#68267=DIRECTION('ref_axis',(0.572061402817695,0.707106781186534,0.415626937777461)) ;
#68268=DIRECTION('',(0.587785252292473,0.,-0.809016994374947)) ;
#68269=DIRECTION('center_axis',(0.309016994374947,0.,0.951056516295154)) ;
#68270=DIRECTION('ref_axis',(0.672498511963948,0.707106781186557,-0.218508012224407)) ;
#68271=DIRECTION('center_axis',(0.,1.,0.)) ;
#68272=DIRECTION('ref_axis',(0.,0.,1.)) ;
#68273=DIRECTION('center_axis',(0.,0.,1.)) ;
#68274=DIRECTION('ref_axis',(-0.707106781186527,0.707106781186568,0.)) ;
#68275=DIRECTION('center_axis',(-0.309016994374948,0.,0.951056516295154)) ;
#68276=DIRECTION('ref_axis',(0.672498511963948,0.707106781186557,0.218508012224408)) ;
#68277=DIRECTION('center_axis',(0.,0.,1.)) ;
#68278=DIRECTION('ref_axis',(0.707106781186506,0.707106781186589,0.)) ;
#68279=DIRECTION('center_axis',(0.,1.,0.)) ;
#68280=DIRECTION('ref_axis',(0.,0.,1.)) ;
#68281=DIRECTION('center_axis',(-0.309016994374948,0.,0.951056516295154)) ;
#68282=DIRECTION('ref_axis',(-0.672498511963948,0.707106781186557,-0.218508012224408)) ;
#68283=DIRECTION('center_axis',(0.,1.,0.)) ;
#68284=DIRECTION('ref_axis',(0.309016994374031,0.,-0.951056516295451)) ;
#68285=DIRECTION('center_axis',(0.,1.,0.)) ;
#68286=DIRECTION('ref_axis',(-3.69482222595252E-13,0.,-1.)) ;
#68287=DIRECTION('center_axis',(0.,1.,0.)) ;
#68288=DIRECTION('ref_axis',(0.,0.,1.)) ;
#68289=DIRECTION('center_axis',(0.,1.,0.)) ;
#68290=DIRECTION('ref_axis',(0.453990499739547,0.,-0.891006524188368)) ;
#68291=DIRECTION('center_axis',(-0.587785252292473,0.,0.809016994374947)) ;
#68292=DIRECTION('ref_axis',(-0.572061402817695,0.707106781186534,-0.415626937777461)) ;
#68293=DIRECTION('',(-0.587785252292473,0.,0.809016994374947)) ;
#68294=DIRECTION('center_axis',(0.,1.,0.)) ;
#68295=DIRECTION('ref_axis',(0.587785252293384,0.,-0.809016994374286)) ;
#68296=DIRECTION('center_axis',(0.,1.,0.)) ;
#68297=DIRECTION('ref_axis',(0.587785252292468,0.,-0.809016994374951)) ;
#68298=DIRECTION('center_axis',(0.,1.,0.)) ;
#68299=DIRECTION('ref_axis',(-0.309016994375651,0.,-0.951056516294925)) ;
#68300=DIRECTION('center_axis',(0.,1.,0.)) ;
#68301=DIRECTION('ref_axis',(0.,0.,1.)) ;
#68302=DIRECTION('center_axis',(0.,1.,0.)) ;
#68303=DIRECTION('ref_axis',(0.707106781186547,0.,-0.707106781186547)) ;
#68304=DIRECTION('center_axis',(-0.809016994374948,0.,0.587785252292473)) ;
#68305=DIRECTION('ref_axis',(-0.415626937777437,0.707106781186575,-0.572061402817662)) ;
#68306=DIRECTION('',(-0.809016994374948,0.,0.587785252292473)) ;
#68307=DIRECTION('center_axis',(0.,1.,0.)) ;
#68308=DIRECTION('ref_axis',(0.809016994375308,0.,-0.587785252291977)) ;
#68309=DIRECTION('center_axis',(0.,1.,0.)) ;
#68310=DIRECTION('ref_axis',(0.809016994374947,0.,-0.587785252292474)) ;
#68311=DIRECTION('center_axis',(0.,1.,0.)) ;
#68312=DIRECTION('ref_axis',(-0.587785252292334,0.,-0.809016994375048)) ;
#68313=DIRECTION('center_axis',(0.,1.,0.)) ;
#68314=DIRECTION('ref_axis',(0.,0.,1.)) ;
#68315=DIRECTION('center_axis',(0.,1.,0.)) ;
#68316=DIRECTION('ref_axis',(0.891006524188368,0.,-0.453990499739547)) ;
#68317=DIRECTION('center_axis',(-0.951056516295154,0.,0.309016994374947)) ;
#68318=DIRECTION('ref_axis',(-0.218508012224405,0.707106781186563,-0.672498511963943)) ;
#68319=DIRECTION('',(-0.951056516295154,0.,0.309016994374947)) ;
#68320=DIRECTION('center_axis',(0.,1.,0.)) ;
#68321=DIRECTION('ref_axis',(0.951056516294886,0.,-0.309016994375771)) ;
#68322=DIRECTION('center_axis',(0.,1.,0.)) ;
#68323=DIRECTION('ref_axis',(0.951056516295153,0.,-0.309016994374948)) ;
#68324=DIRECTION('center_axis',(0.,1.,0.)) ;
#68325=DIRECTION('ref_axis',(-0.809016994374774,0.,-0.587785252292712)) ;
#68326=DIRECTION('center_axis',(0.,1.,0.)) ;
#68327=DIRECTION('ref_axis',(0.,0.,1.)) ;
#68328=DIRECTION('center_axis',(0.,1.,0.)) ;
#68329=DIRECTION('ref_axis',(0.987688340595138,0.,-0.156434465040228)) ;
#68330=DIRECTION('center_axis',(-1.,0.,-2.22044604925031E-16)) ;
#68331=DIRECTION('ref_axis',(1.57009245868373E-16,0.707106781186568,-0.707106781186527)) ;
#68332=DIRECTION('',(-1.,0.,-2.22044604925031E-16)) ;
#68333=DIRECTION('center_axis',(0.,1.,0.)) ;
#68334=DIRECTION('ref_axis',(1.,0.,-4.2632564145606E-14)) ;
#68335=DIRECTION('center_axis',(0.,1.,0.)) ;
#68336=DIRECTION('ref_axis',(1.,0.,0.)) ;
#68337=DIRECTION('center_axis',(0.,1.,0.)) ;
#68338=DIRECTION('ref_axis',(-0.951056516295327,0.,-0.309016994374414)) ;
#68339=DIRECTION('center_axis',(0.,1.,0.)) ;
#68340=DIRECTION('ref_axis',(0.,0.,1.)) ;
#68341=DIRECTION('center_axis',(0.,1.,0.)) ;
#68342=DIRECTION('ref_axis',(0.987688340595138,0.,0.156434465040232)) ;
#68343=DIRECTION('center_axis',(-0.951056516295154,0.,-0.309016994374948)) ;
#68344=DIRECTION('ref_axis',(0.218508012224406,0.707106781186563,-0.672498511963942)) ;
#68345=DIRECTION('',(-0.951056516295153,0.,-0.309016994374948)) ;
#68346=DIRECTION('center_axis',(0.,1.,0.)) ;
#68347=DIRECTION('ref_axis',(0.,0.,1.)) ;
#68348=DIRECTION('center_axis',(0.,1.,0.)) ;
#68349=DIRECTION('ref_axis',(0.951056516295153,0.,0.309016994374948)) ;
#68350=DIRECTION('center_axis',(0.,1.,0.)) ;
#68351=DIRECTION('ref_axis',(-1.,0.,4.68958205601666E-13)) ;
#68352=DIRECTION('center_axis',(0.,1.,0.)) ;
#68353=DIRECTION('ref_axis',(0.,0.,1.)) ;
#68354=DIRECTION('center_axis',(0.,1.,0.)) ;
#68355=DIRECTION('ref_axis',(0.891006524188368,0.,0.453990499739546)) ;
#68356=DIRECTION('center_axis',(-0.809016994374947,0.,-0.587785252292473)) ;
#68357=DIRECTION('ref_axis',(0.415626937777427,0.707106781186592,-0.572061402817648)) ;
#68358=DIRECTION('',(-0.809016994374947,0.,-0.587785252292473)) ;
#68359=DIRECTION('center_axis',(0.,1.,0.)) ;
#68360=DIRECTION('ref_axis',(0.,0.,1.)) ;
#68361=DIRECTION('center_axis',(0.,1.,0.)) ;
#68362=DIRECTION('ref_axis',(0.809016994374947,0.,0.587785252292474)) ;
#68363=DIRECTION('center_axis',(0.,1.,0.)) ;
#68364=DIRECTION('ref_axis',(0.,0.,1.)) ;
#68365=DIRECTION('center_axis',(0.,1.,0.)) ;
#68366=DIRECTION('ref_axis',(0.,0.,1.)) ;
#68367=DIRECTION('center_axis',(0.,1.,0.)) ;
#68368=DIRECTION('ref_axis',(0.707106781186548,0.,0.707106781186547)) ;
#68369=DIRECTION('center_axis',(-0.587785252292473,0.,-0.809016994374948)) ;
#68370=DIRECTION('ref_axis',(0.572061402817668,0.707106781186568,-0.415626937777441)) ;
#68371=DIRECTION('',(-0.587785252292473,0.,-0.809016994374947)) ;
#68372=DIRECTION('center_axis',(0.,1.,0.)) ;
#68373=DIRECTION('ref_axis',(0.,0.,1.)) ;
#68374=DIRECTION('center_axis',(0.,1.,0.)) ;
#68375=DIRECTION('ref_axis',(0.587785252292468,0.,0.809016994374951)) ;
#68376=DIRECTION('center_axis',(0.,1.,0.)) ;
#68377=DIRECTION('ref_axis',(0.,0.,1.)) ;
#68378=DIRECTION('center_axis',(0.,1.,0.)) ;
#68379=DIRECTION('ref_axis',(0.,0.,1.)) ;
#68380=DIRECTION('center_axis',(0.,1.,0.)) ;
#68381=DIRECTION('ref_axis',(0.453990499739549,0.,0.891006524188367)) ;
#68382=DIRECTION('center_axis',(-0.309016994374947,0.,-0.951056516295154)) ;
#68383=DIRECTION('ref_axis',(0.672498511963948,0.707106781186557,-0.218508012224407)) ;
#68384=DIRECTION('',(-0.309016994374947,0.,-0.951056516295154)) ;
#68385=DIRECTION('center_axis',(0.,1.,0.)) ;
#68386=DIRECTION('ref_axis',(0.,0.,1.)) ;
#68387=DIRECTION('center_axis',(0.,1.,0.)) ;
#68388=DIRECTION('ref_axis',(0.309016994374945,0.,0.951056516295154)) ;
#68389=DIRECTION('center_axis',(0.,1.,0.)) ;
#68390=DIRECTION('ref_axis',(0.,0.,1.)) ;
#68391=DIRECTION('center_axis',(0.,1.,0.)) ;
#68392=DIRECTION('ref_axis',(0.,0.,1.)) ;
#68393=DIRECTION('center_axis',(0.,1.,0.)) ;
#68394=DIRECTION('ref_axis',(0.156434465040233,0.,0.987688340595137)) ;
#68395=DIRECTION('center_axis',(1.11022302462516E-16,0.,-1.)) ;
#68396=DIRECTION('ref_axis',(0.707106781186506,0.707106781186589,7.85046229341844E-17)) ;
#68397=DIRECTION('',(1.11022302462516E-16,0.,-1.)) ;
#68398=DIRECTION('center_axis',(0.,1.,0.)) ;
#68399=DIRECTION('ref_axis',(0.,0.,1.)) ;
#68400=DIRECTION('center_axis',(0.,1.,0.)) ;
#68401=DIRECTION('ref_axis',(0.,0.,1.)) ;
#68402=DIRECTION('center_axis',(0.,1.,0.)) ;
#68403=DIRECTION('ref_axis',(0.,0.,1.)) ;
#68404=DIRECTION('center_axis',(0.,1.,0.)) ;
#68405=DIRECTION('ref_axis',(-0.309016994374945,0.,0.951056516295154)) ;
#68406=DIRECTION('center_axis',(0.,-1.,0.)) ;
#68407=DIRECTION('ref_axis',(-1.,0.,0.)) ;
#68408=DIRECTION('',(0.,1.,0.)) ;
#68409=DIRECTION('',(0.,-1.,0.)) ;
#68410=DIRECTION('center_axis',(0.951056516295154,0.,0.309016994374948)) ;
#68411=DIRECTION('ref_axis',(-0.309016994374948,0.,0.951056516295154)) ;
#68412=DIRECTION('',(0.,-1.,0.)) ;
#68413=DIRECTION('center_axis',(0.,-1.,0.)) ;
#68414=DIRECTION('ref_axis',(-0.309016994374937,0.,0.951056516295157)) ;
#68415=DIRECTION('',(0.,-1.,0.)) ;
#68416=DIRECTION('center_axis',(-0.951056516295154,0.,-0.309016994374948)) ;
#68417=DIRECTION('ref_axis',(0.309016994374948,0.,-0.951056516295154)) ;
#68418=DIRECTION('center_axis',(-0.809016994374947,0.,-0.587785252292473)) ;
#68419=DIRECTION('ref_axis',(0.587785252292473,0.,-0.809016994374947)) ;
#68420=DIRECTION('',(0.,-1.,0.)) ;
#68421=DIRECTION('',(0.,-1.,0.)) ;
#68422=DIRECTION('center_axis',(0.809016994374947,0.,0.587785252292473)) ;
#68423=DIRECTION('ref_axis',(-0.587785252292473,0.,0.809016994374947)) ;
#68424=DIRECTION('',(0.,-1.,0.)) ;
#68425=DIRECTION('',(0.,1.,0.)) ;
#68426=DIRECTION('center_axis',(0.,-1.,0.)) ;
#68427=DIRECTION('ref_axis',(0.58778525229247,0.,-0.80901699437495)) ;
#68428=DIRECTION('center_axis',(-0.587785252292473,0.,-0.809016994374948)) ;
#68429=DIRECTION('ref_axis',(0.809016994374948,0.,-0.587785252292473)) ;
#68430=DIRECTION('',(0.,-1.,0.)) ;
#68431=DIRECTION('',(0.,-1.,0.)) ;
#68432=DIRECTION('center_axis',(0.587785252292473,0.,0.809016994374948)) ;
#68433=DIRECTION('ref_axis',(-0.809016994374948,0.,0.587785252292473)) ;
#68434=DIRECTION('',(0.,-1.,0.)) ;
#68435=DIRECTION('',(0.,1.,0.)) ;
#68436=DIRECTION('center_axis',(0.,-1.,0.)) ;
#68437=DIRECTION('ref_axis',(0.809016994374946,0.,-0.587785252292475)) ;
#68438=DIRECTION('center_axis',(-0.309016994374947,0.,-0.951056516295154)) ;
#68439=DIRECTION('ref_axis',(0.951056516295154,0.,-0.309016994374947)) ;
#68440=DIRECTION('',(0.,-1.,0.)) ;
#68441=DIRECTION('',(0.,-1.,0.)) ;
#68442=DIRECTION('center_axis',(0.309016994374947,0.,0.951056516295154)) ;
#68443=DIRECTION('ref_axis',(-0.951056516295154,0.,0.309016994374947)) ;
#68444=DIRECTION('',(0.,-1.,0.)) ;
#68445=DIRECTION('',(0.,1.,0.)) ;
#68446=DIRECTION('center_axis',(0.,-1.,0.)) ;
#68447=DIRECTION('ref_axis',(0.951056516295149,0.,-0.309016994374963)) ;
#68448=DIRECTION('center_axis',(2.22044604925031E-16,0.,-1.)) ;
#68449=DIRECTION('ref_axis',(1.,0.,2.22044604925031E-16)) ;
#68450=DIRECTION('',(0.,-1.,0.)) ;
#68451=DIRECTION('',(0.,-1.,0.)) ;
#68452=DIRECTION('center_axis',(-2.22044604925031E-16,0.,1.)) ;
#68453=DIRECTION('ref_axis',(-1.,0.,-2.22044604925031E-16)) ;
#68454=DIRECTION('',(0.,-1.,0.)) ;
#68455=DIRECTION('',(0.,1.,0.)) ;
#68456=DIRECTION('center_axis',(0.,-1.,0.)) ;
#68457=DIRECTION('ref_axis',(1.,0.,-5.19199337615246E-16)) ;
#68458=DIRECTION('center_axis',(0.309016994374948,0.,-0.951056516295154)) ;
#68459=DIRECTION('ref_axis',(0.951056516295154,0.,0.309016994374948)) ;
#68460=DIRECTION('',(0.,-1.,0.)) ;
#68461=DIRECTION('',(0.,-1.,0.)) ;
#68462=DIRECTION('center_axis',(-0.309016994374948,0.,0.951056516295154)) ;
#68463=DIRECTION('ref_axis',(-0.951056516295154,0.,-0.309016994374948)) ;
#68464=DIRECTION('',(0.,-1.,0.)) ;
#68465=DIRECTION('',(0.,1.,0.)) ;
#68466=DIRECTION('center_axis',(0.,-1.,0.)) ;
#68467=DIRECTION('ref_axis',(0.951056516295154,0.,0.309016994374945)) ;
#68468=DIRECTION('center_axis',(0.587785252292473,0.,-0.809016994374947)) ;
#68469=DIRECTION('ref_axis',(0.809016994374947,0.,0.587785252292473)) ;
#68470=DIRECTION('',(0.,-1.,0.)) ;
#68471=DIRECTION('',(0.,-1.,0.)) ;
#68472=DIRECTION('center_axis',(-0.587785252292473,0.,0.809016994374947)) ;
#68473=DIRECTION('ref_axis',(-0.809016994374947,0.,-0.587785252292473)) ;
#68474=DIRECTION('',(0.,-1.,0.)) ;
#68475=DIRECTION('',(0.,1.,0.)) ;
#68476=DIRECTION('center_axis',(0.,-1.,0.)) ;
#68477=DIRECTION('ref_axis',(0.809016994374945,0.,0.587785252292477)) ;
#68478=DIRECTION('center_axis',(0.809016994374948,0.,-0.587785252292473)) ;
#68479=DIRECTION('ref_axis',(0.587785252292473,0.,0.809016994374948)) ;
#68480=DIRECTION('',(0.,-1.,0.)) ;
#68481=DIRECTION('',(0.,-1.,0.)) ;
#68482=DIRECTION('center_axis',(-0.809016994374948,0.,0.587785252292473)) ;
#68483=DIRECTION('ref_axis',(-0.587785252292473,0.,-0.809016994374948)) ;
#68484=DIRECTION('',(0.,-1.,0.)) ;
#68485=DIRECTION('',(0.,1.,0.)) ;
#68486=DIRECTION('center_axis',(0.,-1.,0.)) ;
#68487=DIRECTION('ref_axis',(0.587785252292472,0.,0.809016994374948)) ;
#68488=DIRECTION('center_axis',(0.951056516295154,0.,-0.309016994374947)) ;
#68489=DIRECTION('ref_axis',(0.309016994374947,0.,0.951056516295154)) ;
#68490=DIRECTION('',(0.,-1.,0.)) ;
#68491=DIRECTION('',(0.,-1.,0.)) ;
#68492=DIRECTION('center_axis',(-0.951056516295154,0.,0.309016994374947)) ;
#68493=DIRECTION('ref_axis',(-0.309016994374947,0.,-0.951056516295154)) ;
#68494=DIRECTION('',(0.,-1.,0.)) ;
#68495=DIRECTION('',(0.,1.,0.)) ;
#68496=DIRECTION('center_axis',(0.,-1.,0.)) ;
#68497=DIRECTION('ref_axis',(0.309016994374948,0.,0.951056516295153)) ;
#68498=DIRECTION('center_axis',(1.,0.,1.11022302462516E-16)) ;
#68499=DIRECTION('ref_axis',(-1.11022302462516E-16,0.,1.)) ;
#68500=DIRECTION('',(0.,-1.,0.)) ;
#68501=DIRECTION('',(0.,-1.,0.)) ;
#68502=DIRECTION('center_axis',(-1.,0.,-1.11022302462516E-16)) ;
#68503=DIRECTION('ref_axis',(1.11022302462516E-16,0.,-1.)) ;
#68504=DIRECTION('',(0.,-1.,0.)) ;
#68505=DIRECTION('center_axis',(0.,-1.,0.)) ;
#68506=DIRECTION('ref_axis',(8.83893312840001E-15,0.,1.)) ;
#68507=DIRECTION('center_axis',(0.,-1.,0.)) ;
#68508=DIRECTION('ref_axis',(-1.,0.,0.)) ;
#68509=DIRECTION('center_axis',(0.,-1.,0.)) ;
#68510=DIRECTION('ref_axis',(-1.,0.,0.)) ;
#68511=DIRECTION('center_axis',(0.,-1.,0.)) ;
#68512=DIRECTION('ref_axis',(-1.,0.,0.)) ;
#68513=DIRECTION('center_axis',(0.,-1.,0.)) ;
#68514=DIRECTION('ref_axis',(-1.,0.,0.)) ;
#68515=DIRECTION('center_axis',(0.,-1.,0.)) ;
#68516=DIRECTION('ref_axis',(-1.,0.,0.)) ;
#68517=DIRECTION('center_axis',(0.,-1.,0.)) ;
#68518=DIRECTION('ref_axis',(-1.,0.,0.)) ;
#68519=DIRECTION('center_axis',(0.,-1.,0.)) ;
#68520=DIRECTION('ref_axis',(-1.,0.,0.)) ;
#68521=DIRECTION('center_axis',(0.,-1.,0.)) ;
#68522=DIRECTION('ref_axis',(-1.,0.,0.)) ;
#68523=DIRECTION('center_axis',(0.,-1.,0.)) ;
#68524=DIRECTION('ref_axis',(-1.,0.,0.)) ;
#68525=DIRECTION('center_axis',(0.,-1.,0.)) ;
#68526=DIRECTION('ref_axis',(-1.,0.,0.)) ;
#68527=DIRECTION('',(0.,-1.,0.)) ;
#101745=CARTESIAN_POINT('',(0.,0.,0.)) ;
#101746=CARTESIAN_POINT('Origin',(40.2,252.25,25.0213203435596)) ;
#101747=CARTESIAN_POINT('',(37.2,252.5,25.0213203435596)) ;
#101748=CARTESIAN_POINT('Origin',(40.2,252.5,25.0213203435596)) ;
#101749=CARTESIAN_POINT('',(36.2317541634482,253.25,25.0213203435596)) ;
#101750=CARTESIAN_POINT('Origin',(36.2317541634482,252.25,25.0213203435596)) ;
#101751=CARTESIAN_POINT('Origin',(40.2,253.25,25.0213203435596)) ;
#101752=CARTESIAN_POINT('Origin',(40.2,253.25,25.0213203435596)) ;
#101753=CARTESIAN_POINT('',(44.6022755871902,253.25,25.0172786696089)) ;
#101754=CARTESIAN_POINT('Ctrl Pts',(44.6022755871902,253.25,25.0172786696089)) ;
#101755=CARTESIAN_POINT('Ctrl Pts',(44.6016731513632,253.25,24.3610929985028)) ;
#101756=CARTESIAN_POINT('Ctrl Pts',(44.299934454168,253.25,23.0448769970944)) ;
#101757=CARTESIAN_POINT('Ctrl Pts',(43.0334270863444,253.25,21.4586695119602)) ;
#101758=CARTESIAN_POINT('Ctrl Pts',(41.2054355147352,253.25,20.58342963668)) ;
#101759=CARTESIAN_POINT('Ctrl Pts',(39.1790659113798,253.25,20.5860610515089)) ;
#101760=CARTESIAN_POINT('Ctrl Pts',(37.352045429714,253.25,21.4697629418411)) ;
#101761=CARTESIAN_POINT('Ctrl Pts',(36.093585354216,253.25,23.0571242602466)) ;
#101762=CARTESIAN_POINT('Ctrl Pts',(35.6505014385247,253.25,25.0155164250954)) ;
#101763=CARTESIAN_POINT('Ctrl Pts',(36.2385167868871,253.25,27.6706849907353)) ;
#101764=CARTESIAN_POINT('Ctrl Pts',(38.5052376987099,253.25,29.4709001024427)) ;
#101765=CARTESIAN_POINT('Ctrl Pts',(41.2187227037567,253.25,29.4547811745837)) ;
#101766=CARTESIAN_POINT('Ctrl Pts',(43.0385614834865,253.25,28.5801018538648)) ;
#101767=CARTESIAN_POINT('Ctrl Pts',(44.3064740862875,253.25,26.9912625003605)) ;
#101768=CARTESIAN_POINT('Ctrl Pts',(44.6028780230171,253.25,25.6734643407148)) ;
#101769=CARTESIAN_POINT('Ctrl Pts',(44.6022755871902,253.25,25.0172786696089)) ;
#101770=CARTESIAN_POINT('Origin',(40.2,259.75,25.0213203435596)) ;
#101771=CARTESIAN_POINT('',(40.2,258.75,29.0213203435596)) ;
#101772=CARTESIAN_POINT('Origin',(40.2,258.75,25.0213203435596)) ;
#101773=CARTESIAN_POINT('',(40.2,259.75,28.0213203435596)) ;
#101774=CARTESIAN_POINT('Origin',(40.2,259.75,29.0213203435596)) ;
#101775=CARTESIAN_POINT('Origin',(40.2,259.75,25.0213203435596)) ;
#101776=CARTESIAN_POINT('Origin',(40.2,258.75,25.0213203435596)) ;
#101777=CARTESIAN_POINT('',(44.6022762317189,258.75,25.0245853614825)) ;
#101778=CARTESIAN_POINT('Ctrl Pts',(44.6022762317189,258.75,25.0245853614825)) ;
#101779=CARTESIAN_POINT('Ctrl Pts',(44.6017895611471,258.75,25.6807711286595)) ;
#101780=CARTESIAN_POINT('Ctrl Pts',(44.3002814452206,258.75,26.9970327213995)) ;
#101781=CARTESIAN_POINT('Ctrl Pts',(43.0340508036911,258.75,28.5834625307185)) ;
#101782=CARTESIAN_POINT('Ctrl Pts',(41.2062107944581,258.75,29.4590205229256)) ;
#101783=CARTESIAN_POINT('Ctrl Pts',(39.179840924666,258.75,29.4567488348315)) ;
#101784=CARTESIAN_POINT('Ctrl Pts',(37.352661518855,258.75,28.573366641583)) ;
#101785=CARTESIAN_POINT('Ctrl Pts',(36.0939258948918,258.75,26.9862351082814)) ;
#101786=CARTESIAN_POINT('Ctrl Pts',(35.6504972551226,258.75,25.0279233442809)) ;
#101787=CARTESIAN_POINT('Ctrl Pts',(36.2380473385298,258.75,22.3726556510516)) ;
#101788=CARTESIAN_POINT('Ctrl Pts',(38.5044538726149,258.75,20.5720464136779)) ;
#101789=CARTESIAN_POINT('Ctrl Pts',(41.2179394265067,258.75,20.5876861131438)) ;
#101790=CARTESIAN_POINT('Ctrl Pts',(43.0379329486519,258.75,21.4620443915897)) ;
#101791=CARTESIAN_POINT('Ctrl Pts',(44.3061264144813,258.75,23.0506570013303)) ;
#101792=CARTESIAN_POINT('Ctrl Pts',(44.6027629022906,258.75,24.3683995943056)) ;
#101793=CARTESIAN_POINT('Ctrl Pts',(44.6022762317189,258.75,25.0245853614825)) ;
#101794=CARTESIAN_POINT('Origin',(40.2,259.75,25.0213203435596)) ;
#101795=CARTESIAN_POINT('',(42.2,259.75,25.0213203435596)) ;
#101796=CARTESIAN_POINT('Origin',(40.2,259.75,25.0213203435596)) ;
#101797=CARTESIAN_POINT('Origin',(40.2,252.5,25.0213203435596)) ;
#101798=CARTESIAN_POINT('',(42.2,252.5,25.0213203435596)) ;
#101799=CARTESIAN_POINT('Origin',(40.2,252.5,25.0213203435596)) ;
#101800=CARTESIAN_POINT('Ctrl Pts',(45.000619097497,253.613636363636,25.0169129554328)) ;
#101801=CARTESIAN_POINT('Ctrl Pts',(45.0012760452229,253.613636363636,25.7324741241569)) ;
#101802=CARTESIAN_POINT('Ctrl Pts',(44.6780517556355,253.613636363636,27.1695143290567)) ;
#101803=CARTESIAN_POINT('Ctrl Pts',(43.2954110430288,253.613636363636,28.9021211121218)) ;
#101804=CARTESIAN_POINT('Ctrl Pts',(41.310902661555,253.613636363636,29.8559465072077)) ;
#101805=CARTESIAN_POINT('Ctrl Pts',(38.3518857445079,253.613636363636,29.8735239694493)) ;
#101806=CARTESIAN_POINT('Ctrl Pts',(35.8800587353911,253.613636363636,27.9104149196633)) ;
#101807=CARTESIAN_POINT('Ctrl Pts',(35.2388363368697,253.613636363636,25.0149912527819)) ;
#101808=CARTESIAN_POINT('Ctrl Pts',(35.7220130633906,253.613636363636,22.8793923697138)) ;
#101809=CARTESIAN_POINT('Ctrl Pts',(37.0943459290232,253.613636363636,21.1483973629633)) ;
#101810=CARTESIAN_POINT('Ctrl Pts',(39.0866858546119,253.613636363636,20.1847329836666)) ;
#101811=CARTESIAN_POINT('Ctrl Pts',(41.2964131703577,253.613636363636,20.1818634631127)) ;
#101812=CARTESIAN_POINT('Ctrl Pts',(43.2898120557582,253.613636363636,21.1363001349984)) ;
#101813=CARTESIAN_POINT('Ctrl Pts',(44.6709203795502,253.613636363636,22.8660369029294)) ;
#101814=CARTESIAN_POINT('Ctrl Pts',(44.9999621497711,253.613636363636,24.3013517867086)) ;
#101815=CARTESIAN_POINT('Ctrl Pts',(45.000619097497,253.613636363636,25.0169129554328)) ;
#101816=CARTESIAN_POINT('Ctrl Pts',(44.9916508494659,253.515394087275,25.0169211890687)) ;
#101817=CARTESIAN_POINT('Ctrl Pts',(44.9923066581649,253.515394087275,25.7312417059043)) ;
#101818=CARTESIAN_POINT('Ctrl Pts',(44.669806273871,253.515394087275,27.1656710082603)) ;
#101819=CARTESIAN_POINT('Ctrl Pts',(43.2898068204824,253.515394087275,28.8951621017486)) ;
#101820=CARTESIAN_POINT('Ctrl Pts',(41.3087556470725,253.515394087275,29.8473173528403)) ;
#101821=CARTESIAN_POINT('Ctrl Pts',(38.3550913443632,253.515394087275,29.8648827277838)) ;
#101822=CARTESIAN_POINT('Ctrl Pts',(35.8876347144536,253.515394087275,27.9052827379527)) ;
#101823=CARTESIAN_POINT('Ctrl Pts',(35.2476065093219,253.515394087275,25.0150115927248)) ;
#101824=CARTESIAN_POINT('Ctrl Pts',(35.7298834843815,253.515394087275,22.8831639909817)) ;
#101825=CARTESIAN_POINT('Ctrl Pts',(37.0998098286885,253.515394087275,21.1552793273844)) ;
#101826=CARTESIAN_POINT('Ctrl Pts',(39.0885241435459,253.515394087275,20.1932807299511)) ;
#101827=CARTESIAN_POINT('Ctrl Pts',(41.2942811943996,253.515394087275,20.1904751850317)) ;
#101828=CARTESIAN_POINT('Ctrl Pts',(43.2840998769856,253.515394087275,21.1431751573701)) ;
#101829=CARTESIAN_POINT('Ctrl Pts',(44.6626199958403,253.515394087275,22.8698547975249)) ;
#101830=CARTESIAN_POINT('Ctrl Pts',(44.990995040767,253.515394087275,24.3026006722331)) ;
#101831=CARTESIAN_POINT('Ctrl Pts',(44.9916508494659,253.515394087275,25.0169211890687)) ;
#101832=CARTESIAN_POINT('Ctrl Pts',(44.8975094841571,253.326587333482,25.0170076190744)) ;
#101833=CARTESIAN_POINT('Ctrl Pts',(44.8981522927289,253.326587333482,25.7171681262213)) ;
#101834=CARTESIAN_POINT('Ctrl Pts',(44.5818309261722,253.326587333482,27.1233188158886)) ;
#101835=CARTESIAN_POINT('Ctrl Pts',(43.2288679887831,253.326587333482,28.8186722353256)) ;
#101836=CARTESIAN_POINT('Ctrl Pts',(41.287065783851,253.326587333482,29.7519743071556)) ;
#101837=CARTESIAN_POINT('Ctrl Pts',(38.3916613445224,253.326587333482,29.7691674220623)) ;
#101838=CARTESIAN_POINT('Ctrl Pts',(35.9730064201748,253.326587333482,27.848274780733)) ;
#101839=CARTESIAN_POINT('Ctrl Pts',(35.345557667694,253.326587333482,25.0151243958764)) ;
#101840=CARTESIAN_POINT('Ctrl Pts',(35.8183555821575,253.326587333482,22.9254729931295)) ;
#101841=CARTESIAN_POINT('Ctrl Pts',(37.1611613325258,253.326587333482,21.2316974982721)) ;
#101842=CARTESIAN_POINT('Ctrl Pts',(39.1106773513727,253.326587333482,20.2887752336348)) ;
#101843=CARTESIAN_POINT('Ctrl Pts',(41.2728914527978,253.326587333482,20.2859481042472)) ;
#101844=CARTESIAN_POINT('Ctrl Pts',(43.223428131217,253.326587333482,21.2198697969633)) ;
#101845=CARTESIAN_POINT('Ctrl Pts',(44.5748751166589,253.326587333482,22.9123973805586)) ;
#101846=CARTESIAN_POINT('Ctrl Pts',(44.8968666755852,253.326587333482,24.3168471119274)) ;
#101847=CARTESIAN_POINT('Ctrl Pts',(44.8975094841571,253.326587333482,25.0170076190744)) ;
#101848=CARTESIAN_POINT('Ctrl Pts',(44.7009263155318,253.25,25.0171880996136)) ;
#101849=CARTESIAN_POINT('Ctrl Pts',(44.7015422706035,253.25,25.6880992141915)) ;
#101850=CARTESIAN_POINT('Ctrl Pts',(44.3985223913072,253.25,27.0354440223192)) ;
#101851=CARTESIAN_POINT('Ctrl Pts',(43.1022098056181,253.25,28.6599141245163)) ;
#101852=CARTESIAN_POINT('Ctrl Pts',(41.2415356604866,253.25,29.5542185254571)) ;
#101853=CARTESIAN_POINT('Ctrl Pts',(38.4672058727508,253.25,29.5707031873526)) ;
#101854=CARTESIAN_POINT('Ctrl Pts',(36.1496360084533,253.25,27.7301124807667)) ;
#101855=CARTESIAN_POINT('Ctrl Pts',(35.5484429988492,253.25,25.0153882218719)) ;
#101856=CARTESIAN_POINT('Ctrl Pts',(36.0014566262198,253.25,23.0130584206935)) ;
#101857=CARTESIAN_POINT('Ctrl Pts',(37.2881518479859,253.25,21.3900989657002)) ;
#101858=CARTESIAN_POINT('Ctrl Pts',(39.1561351002536,253.25,20.4865648490839)) ;
#101859=CARTESIAN_POINT('Ctrl Pts',(41.2279480953328,253.25,20.4838872476943)) ;
#101860=CARTESIAN_POINT('Ctrl Pts',(43.0969345312123,253.25,21.3787505013531)) ;
#101861=CARTESIAN_POINT('Ctrl Pts',(44.391821336157,253.25,23.000541357777)) ;
#101862=CARTESIAN_POINT('Ctrl Pts',(44.70031036046,253.25,24.3462769850356)) ;
#101863=CARTESIAN_POINT('Ctrl Pts',(44.7009263155318,253.25,25.0171880996136)) ;
#101864=CARTESIAN_POINT('Ctrl Pts',(44.6022755871902,253.25,25.0172786696089)) ;
#101865=CARTESIAN_POINT('Ctrl Pts',(44.6028780230171,253.25,25.6734643407148)) ;
#101866=CARTESIAN_POINT('Ctrl Pts',(44.3064740862875,253.25,26.9912625003605)) ;
#101867=CARTESIAN_POINT('Ctrl Pts',(43.0385614834865,253.25,28.5801018538648)) ;
#101868=CARTESIAN_POINT('Ctrl Pts',(41.2187227037567,253.25,29.4547811745837)) ;
#101869=CARTESIAN_POINT('Ctrl Pts',(38.5052376987099,253.25,29.4709001024427)) ;
#101870=CARTESIAN_POINT('Ctrl Pts',(36.2385167868871,253.25,27.6706849907353)) ;
#101871=CARTESIAN_POINT('Ctrl Pts',(35.6505014385247,253.25,25.0155164250954)) ;
#101872=CARTESIAN_POINT('Ctrl Pts',(36.093585354216,253.25,23.0571242602466)) ;
#101873=CARTESIAN_POINT('Ctrl Pts',(37.352045429714,253.25,21.4697629418411)) ;
#101874=CARTESIAN_POINT('Ctrl Pts',(39.1790659113798,253.25,20.5860610515089)) ;
#101875=CARTESIAN_POINT('Ctrl Pts',(41.2054355147352,253.25,20.58342963668)) ;
#101876=CARTESIAN_POINT('Ctrl Pts',(43.0334270863444,253.25,21.4586695119602)) ;
#101877=CARTESIAN_POINT('Ctrl Pts',(44.299934454168,253.25,23.0448769970944)) ;
#101878=CARTESIAN_POINT('Ctrl Pts',(44.6016731513632,253.25,24.3610929985028)) ;
#101879=CARTESIAN_POINT('Ctrl Pts',(44.6022755871902,253.25,25.0172786696089)) ;
#101880=CARTESIAN_POINT('',(45.000619097497,253.613636363636,25.0169129554328)) ;
#101881=CARTESIAN_POINT('Ctrl Pts',(44.6022755871902,253.25,25.0172786696089)) ;
#101882=CARTESIAN_POINT('Ctrl Pts',(44.7009263155318,253.25,25.0171880996136)) ;
#101883=CARTESIAN_POINT('Ctrl Pts',(44.8975094841571,253.326587333482,25.0170076190744)) ;
#101884=CARTESIAN_POINT('Ctrl Pts',(44.9916508494659,253.515394087275,25.0169211890687)) ;
#101885=CARTESIAN_POINT('Ctrl Pts',(45.000619097497,253.613636363636,25.0169129554328)) ;
#101886=CARTESIAN_POINT('',(40.199018407139,253.613636363636,29.8223164415809)) ;
#101887=CARTESIAN_POINT('Ctrl Pts',(45.000619097497,253.613636363636,25.0169129554328)) ;
#101888=CARTESIAN_POINT('Ctrl Pts',(45.0012760452229,253.613636363636,25.7324741241569)) ;
#101889=CARTESIAN_POINT('Ctrl Pts',(44.6780517556355,253.613636363636,27.1695143290567)) ;
#101890=CARTESIAN_POINT('Ctrl Pts',(43.2954110430288,253.613636363636,28.9021211121218)) ;
#101891=CARTESIAN_POINT('Ctrl Pts',(41.6409075118807,253.613636363636,29.6973344249002)) ;
#101892=CARTESIAN_POINT('Ctrl Pts',(40.5597413925216,253.613636363636,29.8213340913974)) ;
#101893=CARTESIAN_POINT('Ctrl Pts',(40.199018407139,253.613636363636,29.8223164415809)) ;
#101894=CARTESIAN_POINT('Ctrl Pts',(40.199018407139,253.613636363636,29.8223164415809)) ;
#101895=CARTESIAN_POINT('Ctrl Pts',(39.8399201468488,253.613636363636,29.8232943671808)) ;
#101896=CARTESIAN_POINT('Ctrl Pts',(38.0422099661677,253.613636363636,29.6275814659016)) ;
#101897=CARTESIAN_POINT('Ctrl Pts',(35.8800587353911,253.613636363636,27.9104149196633)) ;
#101898=CARTESIAN_POINT('Ctrl Pts',(35.2388363368697,253.613636363636,25.0149912527819)) ;
#101899=CARTESIAN_POINT('Ctrl Pts',(35.7220130633906,253.613636363636,22.8793923697138)) ;
#101900=CARTESIAN_POINT('Ctrl Pts',(37.0943459290232,253.613636363636,21.1483973629633)) ;
#101901=CARTESIAN_POINT('Ctrl Pts',(39.0866858546119,253.613636363636,20.1847329836666)) ;
#101902=CARTESIAN_POINT('Ctrl Pts',(41.2964131703577,253.613636363636,20.1818634631127)) ;
#101903=CARTESIAN_POINT('Ctrl Pts',(43.2898120557582,253.613636363636,21.1363001349984)) ;
#101904=CARTESIAN_POINT('Ctrl Pts',(44.6709203795502,253.613636363636,22.8660369029294)) ;
#101905=CARTESIAN_POINT('Ctrl Pts',(44.9999621497711,253.613636363636,24.3013517867086)) ;
#101906=CARTESIAN_POINT('Ctrl Pts',(45.000619097497,253.613636363636,25.0169129554328)) ;
#101907=CARTESIAN_POINT('Ctrl Pts',(45.0006198003464,258.386363636364,25.0248807993021)) ;
#101908=CARTESIAN_POINT('Ctrl Pts',(45.0011505077032,258.386363636364,24.309319525814)) ;
#101909=CARTESIAN_POINT('Ctrl Pts',(44.6776726244613,258.386363636364,22.8723399155802)) ;
#101910=CARTESIAN_POINT('Ctrl Pts',(43.2947256347052,258.386363636364,21.1399803933739)) ;
#101911=CARTESIAN_POINT('Ctrl Pts',(41.3100485088219,258.386363636364,20.1865050903338)) ;
#101912=CARTESIAN_POINT('Ctrl Pts',(38.351030993267,258.386363636364,20.1694502198588)) ;
#101913=CARTESIAN_POINT('Ctrl Pts',(35.8795468086148,258.386363636364,22.1329890580946)) ;
#101914=CARTESIAN_POINT('Ctrl Pts',(35.2388317749291,258.386363636364,25.0285208222065)) ;
#101915=CARTESIAN_POINT('Ctrl Pts',(35.7223844181683,258.386363636364,27.1640320292898)) ;
#101916=CARTESIAN_POINT('Ctrl Pts',(37.0950177654945,258.386363636364,28.8947764586432)) ;
#101917=CARTESIAN_POINT('Ctrl Pts',(39.0875309956096,258.386363636364,29.8580922128038)) ;
#101918=CARTESIAN_POINT('Ctrl Pts',(41.297258601901,258.386363636364,29.8605694564547)) ;
#101919=CARTESIAN_POINT('Ctrl Pts',(43.2904922106796,258.386363636364,28.9057858825717)) ;
#101920=CARTESIAN_POINT('Ctrl Pts',(44.6712987683722,258.386363636364,27.1758066732701)) ;
#101921=CARTESIAN_POINT('Ctrl Pts',(45.0000890929896,258.386363636364,25.7404420727902)) ;
#101922=CARTESIAN_POINT('Ctrl Pts',(45.0006198003464,258.386363636364,25.0248807993021)) ;
#101923=CARTESIAN_POINT('Ctrl Pts',(44.9916515510023,258.484605912725,25.0248741478579)) ;
#101924=CARTESIAN_POINT('Ctrl Pts',(44.9921813382098,258.484605912725,24.31055352644)) ;
#101925=CARTESIAN_POINT('Ctrl Pts',(44.6694274518689,258.484605912725,22.876183617039)) ;
#101926=CARTESIAN_POINT('Ctrl Pts',(43.2891212929352,258.484605912725,21.1469383147985)) ;
#101927=CARTESIAN_POINT('Ctrl Pts',(41.3079016216169,258.484605912725,20.1951323949763)) ;
#101928=CARTESIAN_POINT('Ctrl Pts',(38.3542352604705,258.484605912725,20.1780888057549)) ;
#101929=CARTESIAN_POINT('Ctrl Pts',(35.8871201680428,258.484605912725,22.1381188352666)) ;
#101930=CARTESIAN_POINT('Ctrl Pts',(35.2475978217452,258.484605912725,25.0284991827555)) ;
#101931=CARTESIAN_POINT('Ctrl Pts',(35.7302504339899,258.484605912725,27.1602597668809)) ;
#101932=CARTESIAN_POINT('Ctrl Pts',(37.1004769335098,258.484605912725,28.8878953905237)) ;
#101933=CARTESIAN_POINT('Ctrl Pts',(39.0893652161804,258.484605912725,29.8495459249166)) ;
#101934=CARTESIAN_POINT('Ctrl Pts',(41.2951234207584,258.484605912725,29.8519604630792)) ;
#101935=CARTESIAN_POINT('Ctrl Pts',(43.2847776365318,258.484605912725,28.8989133639222)) ;
#101936=CARTESIAN_POINT('Ctrl Pts',(44.6629974245713,258.484605912725,27.1719911235959)) ;
#101937=CARTESIAN_POINT('Ctrl Pts',(44.9911217637948,258.484605912725,25.7391947692758)) ;
#101938=CARTESIAN_POINT('Ctrl Pts',(44.9916515510023,258.484605912725,25.0248741478579)) ;
#101939=CARTESIAN_POINT('Ctrl Pts',(44.8975099394367,258.673412411855,25.0248043262399)) ;
#101940=CARTESIAN_POINT('Ctrl Pts',(44.8980292246472,258.673412411855,24.3246437165838)) ;
#101941=CARTESIAN_POINT('Ctrl Pts',(44.5814598954824,258.673412411855,22.9185527200586)) ;
#101942=CARTESIAN_POINT('Ctrl Pts',(43.228197675365,258.673412411855,21.2234416213897)) ;
#101943=CARTESIAN_POINT('Ctrl Pts',(41.2862303788559,258.673412411855,20.2904821630844)) ;
#101944=CARTESIAN_POINT('Ctrl Pts',(38.390825913078,258.673412411855,20.2738003530344)) ;
#101945=CARTESIAN_POINT('Ctrl Pts',(35.9725066923928,258.673412411855,22.1951131679698)) ;
#101946=CARTESIAN_POINT('Ctrl Pts',(35.3455546200851,258.673412411855,25.0283688520011)) ;
#101947=CARTESIAN_POINT('Ctrl Pts',(35.8187202161855,258.673412411855,27.1179342822305)) ;
#101948=CARTESIAN_POINT('Ctrl Pts',(37.1618199075666,258.673412411855,28.8114641917246)) ;
#101949=CARTESIAN_POINT('Ctrl Pts',(39.1115051232266,258.673412411855,29.7540453502129)) ;
#101950=CARTESIAN_POINT('Ctrl Pts',(41.2737191756229,258.673412411855,29.7564884307353)) ;
#101951=CARTESIAN_POINT('Ctrl Pts',(43.2240939182987,258.673412411855,28.822227602684)) ;
#101952=CARTESIAN_POINT('Ctrl Pts',(44.5752452635221,258.673412411855,27.1294630065087)) ;
#101953=CARTESIAN_POINT('Ctrl Pts',(44.8969906542263,258.673412411855,25.7249649358961)) ;
#101954=CARTESIAN_POINT('Ctrl Pts',(44.8975099394367,258.673412411855,25.0248043262399)) ;
#101955=CARTESIAN_POINT('Ctrl Pts',(44.7009269745037,258.75,25.0246585273691)) ;
#101956=CARTESIAN_POINT('Ctrl Pts',(44.7014245664355,258.75,24.3537473145643)) ;
#101957=CARTESIAN_POINT('Ctrl Pts',(44.3981668414899,258.75,23.006459080954)) ;
#101958=CARTESIAN_POINT('Ctrl Pts',(43.1015668807325,258.75,21.382220583903)) ;
#101959=CARTESIAN_POINT('Ctrl Pts',(41.24073451057,258.75,20.4882443962037)) ;
#101960=CARTESIAN_POINT('Ctrl Pts',(38.466403843111,258.75,20.472249738864)) ;
#101961=CARTESIAN_POINT('Ctrl Pts',(36.1491552604752,258.75,22.3132436329432)) ;
#101962=CARTESIAN_POINT('Ctrl Pts',(35.5484378202547,258.75,25.0280695257637)) ;
#101963=CARTESIAN_POINT('Ctrl Pts',(36.0018039888119,258.75,27.0303172322302)) ;
#101964=CARTESIAN_POINT('Ctrl Pts',(37.2887809850285,258.75,28.6530419860233)) ;
#101965=CARTESIAN_POINT('Ctrl Pts',(39.1569269380008,258.75,29.5562492220073)) ;
#101966=CARTESIAN_POINT('Ctrl Pts',(41.2287403938204,258.75,29.5585591526955)) ;
#101967=CARTESIAN_POINT('Ctrl Pts',(43.0975719802107,258.75,28.663370463087)) ;
#101968=CARTESIAN_POINT('Ctrl Pts',(44.3921760477315,258.75,27.0413521670251)) ;
#101969=CARTESIAN_POINT('Ctrl Pts',(44.7004293825719,258.75,25.6955697401738)) ;
#101970=CARTESIAN_POINT('Ctrl Pts',(44.7009269745037,258.75,25.0246585273691)) ;
#101971=CARTESIAN_POINT('Ctrl Pts',(44.6022762317189,258.75,25.0245853614825)) ;
#101972=CARTESIAN_POINT('Ctrl Pts',(44.6027629022906,258.75,24.3683995943056)) ;
#101973=CARTESIAN_POINT('Ctrl Pts',(44.3061264144813,258.75,23.0506570013303)) ;
#101974=CARTESIAN_POINT('Ctrl Pts',(43.0379329486519,258.75,21.4620443915897)) ;
#101975=CARTESIAN_POINT('Ctrl Pts',(41.2179394265067,258.75,20.5876861131438)) ;
#101976=CARTESIAN_POINT('Ctrl Pts',(38.5044538726149,258.75,20.5720464136779)) ;
#101977=CARTESIAN_POINT('Ctrl Pts',(36.2380473385298,258.75,22.3726556510516)) ;
#101978=CARTESIAN_POINT('Ctrl Pts',(35.6504972551226,258.75,25.0279233442809)) ;
#101979=CARTESIAN_POINT('Ctrl Pts',(36.0939258948918,258.75,26.9862351082814)) ;
#101980=CARTESIAN_POINT('Ctrl Pts',(37.352661518855,258.75,28.573366641583)) ;
#101981=CARTESIAN_POINT('Ctrl Pts',(39.179840924666,258.75,29.4567488348315)) ;
#101982=CARTESIAN_POINT('Ctrl Pts',(41.2062107944581,258.75,29.4590205229256)) ;
#101983=CARTESIAN_POINT('Ctrl Pts',(43.0340508036911,258.75,28.5834625307185)) ;
#101984=CARTESIAN_POINT('Ctrl Pts',(44.3002814452206,258.75,26.9970327213995)) ;
#101985=CARTESIAN_POINT('Ctrl Pts',(44.6017895611471,258.75,25.6807711286595)) ;
#101986=CARTESIAN_POINT('Ctrl Pts',(44.6022762317189,258.75,25.0245853614825)) ;
#101987=CARTESIAN_POINT('',(45.0006198003464,258.386363636364,25.0248807993021)) ;
#101988=CARTESIAN_POINT('Ctrl Pts',(44.6022762317189,258.75,25.0245853614825)) ;
#101989=CARTESIAN_POINT('Ctrl Pts',(44.7009269745037,258.75,25.0246585273691)) ;
#101990=CARTESIAN_POINT('Ctrl Pts',(44.8975099394367,258.673412411855,25.0248043262399)) ;
#101991=CARTESIAN_POINT('Ctrl Pts',(44.9916515510023,258.484605912725,25.0248741478579)) ;
#101992=CARTESIAN_POINT('Ctrl Pts',(45.0006198003464,258.386363636364,25.0248807993021)) ;
#101993=CARTESIAN_POINT('',(40.1990240993093,258.386363636364,20.2203337107496)) ;
#101994=CARTESIAN_POINT('Ctrl Pts',(45.0006198003464,258.386363636364,25.0248807993021)) ;
#101995=CARTESIAN_POINT('Ctrl Pts',(45.0011505077032,258.386363636364,24.309319525814)) ;
#101996=CARTESIAN_POINT('Ctrl Pts',(44.6776726244613,258.386363636364,22.8723399155802)) ;
#101997=CARTESIAN_POINT('Ctrl Pts',(43.2947256347052,258.386363636364,21.1399803933739)) ;
#101998=CARTESIAN_POINT('Ctrl Pts',(41.6403427347236,258.386363636364,20.3451844961812)) ;
#101999=CARTESIAN_POINT('Ctrl Pts',(40.5594630598394,258.386363636364,20.2213153661189)) ;
#102000=CARTESIAN_POINT('Ctrl Pts',(40.1990240993093,258.386363636364,20.2203337107496)) ;
#102001=CARTESIAN_POINT('Ctrl Pts',(40.1990240993093,258.386363636364,20.2203337107496)) ;
#102002=CARTESIAN_POINT('Ctrl Pts',(39.8396412077929,258.386363636364,20.2193549315838)) ;
#102003=CARTESIAN_POINT('Ctrl Pts',(38.0416422229935,258.386363636364,20.4152526693822)) ;
#102004=CARTESIAN_POINT('Ctrl Pts',(35.8795468086148,258.386363636364,22.1329890580946)) ;
#102005=CARTESIAN_POINT('Ctrl Pts',(35.2388317749291,258.386363636364,25.0285208222065)) ;
#102006=CARTESIAN_POINT('Ctrl Pts',(35.7223844181683,258.386363636364,27.1640320292898)) ;
#102007=CARTESIAN_POINT('Ctrl Pts',(37.0950177654945,258.386363636364,28.8947764586432)) ;
#102008=CARTESIAN_POINT('Ctrl Pts',(39.0875309956096,258.386363636364,29.8580922128038)) ;
#102009=CARTESIAN_POINT('Ctrl Pts',(41.297258601901,258.386363636364,29.8605694564547)) ;
#102010=CARTESIAN_POINT('Ctrl Pts',(43.2904922106796,258.386363636364,28.9057858825717)) ;
#102011=CARTESIAN_POINT('Ctrl Pts',(44.6712987683722,258.386363636364,27.1758066732701)) ;
#102012=CARTESIAN_POINT('Ctrl Pts',(45.0000890929896,258.386363636364,25.7404420727902)) ;
#102013=CARTESIAN_POINT('Ctrl Pts',(45.0006198003464,258.386363636364,25.0248807993021)) ;
#102014=CARTESIAN_POINT('Origin',(40.2,253.9,25.0213203435596)) ;
#102015=CARTESIAN_POINT('',(38.3418047738311,253.75,29.6093057948708)) ;
#102016=CARTESIAN_POINT('',(37.580461549766,253.75,29.2213820464094)) ;
#102017=CARTESIAN_POINT('Origin',(40.2,253.75,25.0213203435596)) ;
#102018=CARTESIAN_POINT('',(38.1565530819608,253.9,29.694041680549)) ;
#102019=CARTESIAN_POINT('Ctrl Pts',(38.3418047738311,253.75,29.6093057948708)) ;
#102020=CARTESIAN_POINT('Ctrl Pts',(38.3410897979463,253.75,29.6096388244826)) ;
#102021=CARTESIAN_POINT('Ctrl Pts',(38.3403747898381,253.750003330106,29.6099717982194)) ;
#102022=CARTESIAN_POINT('Ctrl Pts',(38.3212338170963,253.750181671152,29.6188837045809)) ;
#102023=CARTESIAN_POINT('Ctrl Pts',(38.3027198224331,253.752566842488,29.6274555764536)) ;
#102024=CARTESIAN_POINT('Ctrl Pts',(38.2675842178259,253.761740190968,29.6436380121775)) ;
#102025=CARTESIAN_POINT('Ctrl Pts',(38.2507597781158,253.768377217198,29.6513456347974)) ;
#102026=CARTESIAN_POINT('Ctrl Pts',(38.2177054917617,253.78721321578,29.6664219076506)) ;
#102027=CARTESIAN_POINT('Ctrl Pts',(38.2015932119542,253.800023548159,29.6737287158086)) ;
#102028=CARTESIAN_POINT('Ctrl Pts',(38.1781795794102,253.828041657271,29.6843112161272)) ;
#102029=CARTESIAN_POINT('Ctrl Pts',(38.1698022074386,253.841958224525,29.6880838741351)) ;
#102030=CARTESIAN_POINT('Ctrl Pts',(38.1592036720168,253.870954690135,29.6928518010587)) ;
#102031=CARTESIAN_POINT('Ctrl Pts',(38.1565530819608,253.885320776746,29.694041680549)) ;
#102032=CARTESIAN_POINT('Ctrl Pts',(38.1565530819608,253.9,29.694041680549)) ;
#102033=CARTESIAN_POINT('',(37.6207969906631,253.9,29.4210603173112)) ;
#102034=CARTESIAN_POINT('Origin',(40.2,253.9,25.0213203435596)) ;
#102035=CARTESIAN_POINT('Ctrl Pts',(37.580461549766,253.75,29.2213820464094)) ;
#102036=CARTESIAN_POINT('Ctrl Pts',(37.5806123754316,253.75,29.2221562239469)) ;
#102037=CARTESIAN_POINT('Ctrl Pts',(37.5807632652411,253.750003330105,29.2229303947064)) ;
#102038=CARTESIAN_POINT('Ctrl Pts',(37.5848041630354,253.750181671152,29.2436540540753)) ;
#102039=CARTESIAN_POINT('Ctrl Pts',(37.5887516260403,253.752566842488,29.2636706102621)) ;
#102040=CARTESIAN_POINT('Ctrl Pts',(37.5963119507477,253.761740190968,29.3016077085614)) ;
#102041=CARTESIAN_POINT('Ctrl Pts',(37.5999655106017,253.768377217198,29.3197493931139)) ;
#102042=CARTESIAN_POINT('Ctrl Pts',(37.6071973716956,253.78721321578,29.3553524833539)) ;
#102043=CARTESIAN_POINT('Ctrl Pts',(37.6107566001729,253.800023548159,29.372682425613)) ;
#102044=CARTESIAN_POINT('Ctrl Pts',(37.6159573654841,253.828041657271,29.3978446898608)) ;
#102045=CARTESIAN_POINT('Ctrl Pts',(37.6178293167396,253.841958224525,29.406839638893)) ;
#102046=CARTESIAN_POINT('Ctrl Pts',(37.6202016456472,253.870954690135,29.4182165512944)) ;
#102047=CARTESIAN_POINT('Ctrl Pts',(37.6207969906631,253.885320776746,29.4210603173112)) ;
#102048=CARTESIAN_POINT('Ctrl Pts',(37.6207969906631,253.9,29.4210603173112)) ;
#102049=CARTESIAN_POINT('Origin',(39.0213365437268,253.9,27.5179220536754)) ;
#102050=CARTESIAN_POINT('',(38.1739035596879,253.75,30.1260525975112)) ;
#102051=CARTESIAN_POINT('',(39.0213365437268,253.75,27.5179220536754)) ;
#102052=CARTESIAN_POINT('',(38.0323928885057,253.9,30.0761674639184)) ;
#102053=CARTESIAN_POINT('Ctrl Pts',(38.1739035596879,253.75,30.1260525975112)) ;
#102054=CARTESIAN_POINT('Ctrl Pts',(38.172529049521,253.75,30.1255643186931)) ;
#102055=CARTESIAN_POINT('Ctrl Pts',(38.1711545707753,253.750021261236,30.1250761825186)) ;
#102056=CARTESIAN_POINT('Ctrl Pts',(38.1697805624966,253.750063777237,30.1245883423369)) ;
#102057=CARTESIAN_POINT('Ctrl Pts',(38.1521290671495,253.750609968276,30.1183211976405)) ;
#102058=CARTESIAN_POINT('Ctrl Pts',(38.1347220873535,253.754658837467,30.1121625030257)) ;
#102059=CARTESIAN_POINT('Ctrl Pts',(38.1184645303643,253.762001431812,30.1064243414529)) ;
#102060=CARTESIAN_POINT('Ctrl Pts',(38.1015160468841,253.769656077527,30.1004423149597)) ;
#102061=CARTESIAN_POINT('Ctrl Pts',(38.0861341004722,253.78074710398,30.0950289612179)) ;
#102062=CARTESIAN_POINT('Ctrl Pts',(38.0731882320494,253.794651469056,30.0904794283364)) ;
#102063=CARTESIAN_POINT('Ctrl Pts',(38.0602458273977,253.808552113907,30.0859311127188)) ;
#102064=CARTESIAN_POINT('Ctrl Pts',(38.0499858937768,253.824998688613,30.0823329269323)) ;
#102065=CARTESIAN_POINT('Ctrl Pts',(38.0429889324131,253.843066458683,30.0798802263626)) ;
#102066=CARTESIAN_POINT('Ctrl Pts',(38.0359928332805,253.861132002274,30.0774278280375)) ;
#102067=CARTESIAN_POINT('Ctrl Pts',(38.0323928885057,253.880472526098,30.0761674639184)) ;
#102068=CARTESIAN_POINT('Ctrl Pts',(38.0323928885057,253.9,30.0761674639184)) ;
#102069=CARTESIAN_POINT('',(38.8786780662825,253.9,27.4715695045192)) ;
#102070=CARTESIAN_POINT('Origin',(38.5004065309378,253.9,30.252131183183)) ;
#102071=CARTESIAN_POINT('',(38.8386601166806,253.75,30.3420450960781)) ;
#102072=CARTESIAN_POINT('Origin',(38.5004065309378,253.75,30.252131183183)) ;
#102073=CARTESIAN_POINT('',(38.982466400387,253.9,30.3848650607978)) ;
#102074=CARTESIAN_POINT('Ctrl Pts',(38.8386601166829,253.75,30.3420450960789)) ;
#102075=CARTESIAN_POINT('Ctrl Pts',(38.8400591218546,253.75,30.3424579870221)) ;
#102076=CARTESIAN_POINT('Ctrl Pts',(38.8414580177618,253.750021261236,30.3428709748967)) ;
#102077=CARTESIAN_POINT('Ctrl Pts',(38.8428563590733,253.750063777237,30.343283925702)) ;
#102078=CARTESIAN_POINT('Ctrl Pts',(38.8608204540119,253.750609968276,30.3485889877857)) ;
#102079=CARTESIAN_POINT('Ctrl Pts',(38.8785229863552,253.754658837467,30.3538380651884)) ;
#102080=CARTESIAN_POINT('Ctrl Pts',(38.8950484329941,253.762001431812,30.3587517471959)) ;
#102081=CARTESIAN_POINT('Ctrl Pts',(38.9122761911101,253.769656077527,30.3638742547404)) ;
#102082=CARTESIAN_POINT('Ctrl Pts',(38.927902336659,253.78074710398,30.3685360408181)) ;
#102083=CARTESIAN_POINT('Ctrl Pts',(38.9410499125525,253.794651469056,30.3724647819375)) ;
#102084=CARTESIAN_POINT('Ctrl Pts',(38.9541939707066,253.808552113907,30.3763924718906)) ;
#102085=CARTESIAN_POINT('Ctrl Pts',(38.9646093919075,253.824998688613,30.3795121161123)) ;
#102086=CARTESIAN_POINT('Ctrl Pts',(38.9717117137828,253.843066458683,30.3816405503697)) ;
#102087=CARTESIAN_POINT('Ctrl Pts',(38.9788131604437,253.861132002274,30.3837687223415)) ;
#102088=CARTESIAN_POINT('Ctrl Pts',(38.982466400387,253.880472526098,30.3848650607978)) ;
#102089=CARTESIAN_POINT('Ctrl Pts',(38.982466400387,253.9,30.3848650607978)) ;
#102090=CARTESIAN_POINT('Origin',(38.5004065309378,253.9,30.252131183183)) ;
#102091=CARTESIAN_POINT('Origin',(39.7947637665017,253.9,27.3994606331908)) ;
#102092=CARTESIAN_POINT('',(39.0065613308239,253.75,29.8252982934377)) ;
#102093=CARTESIAN_POINT('',(39.7947637665017,253.75,27.3994606331908)) ;
#102094=CARTESIAN_POINT('',(39.1066265938421,253.9,30.0027392774284)) ;
#102095=CARTESIAN_POINT('Ctrl Pts',(39.0065613308239,253.75,29.8252982934377)) ;
#102096=CARTESIAN_POINT('Ctrl Pts',(39.0069440085702,253.75,29.8259879723329)) ;
#102097=CARTESIAN_POINT('Ctrl Pts',(39.0073267452283,253.750003330105,29.8266776249647)) ;
#102098=CARTESIAN_POINT('Ctrl Pts',(39.0175738303363,253.750181671152,29.8451382901555)) ;
#102099=CARTESIAN_POINT('Ctrl Pts',(39.0275135467812,253.752566842487,29.8629553331985)) ;
#102100=CARTESIAN_POINT('Ctrl Pts',(39.0464270509519,253.761740190968,29.896699388929)) ;
#102101=CARTESIAN_POINT('Ctrl Pts',(39.0555078816925,253.768377217198,29.9128241441551)) ;
#102102=CARTESIAN_POINT('Ctrl Pts',(39.0733877502475,253.78721321578,29.9444499271496)) ;
#102103=CARTESIAN_POINT('Ctrl Pts',(39.0821280243534,253.800023548159,29.9598318195758)) ;
#102104=CARTESIAN_POINT('Ctrl Pts',(39.0948498133619,253.828041657271,29.9821554300886)) ;
#102105=CARTESIAN_POINT('Ctrl Pts',(39.0994097369161,253.841958224525,29.9901316702288)) ;
#102106=CARTESIAN_POINT('Ctrl Pts',(39.1051816150581,253.870954690135,30.0002186669547)) ;
#102107=CARTESIAN_POINT('Ctrl Pts',(39.1066265938421,253.885320776746,30.0027392774284)) ;
#102108=CARTESIAN_POINT('Ctrl Pts',(39.1066265938421,253.9,30.0027392774284)) ;
#102109=CARTESIAN_POINT('',(39.9374222439459,253.9,27.445813182347)) ;
#102110=CARTESIAN_POINT('Origin',(40.2,253.9,25.0213203435596)) ;
#102111=CARTESIAN_POINT('',(39.8505167960037,253.75,29.9589677074491)) ;
#102112=CARTESIAN_POINT('Origin',(40.2,253.75,25.0213203435596)) ;
#102113=CARTESIAN_POINT('',(39.7005167960037,253.9,30.096802244712)) ;
#102114=CARTESIAN_POINT('Ctrl Pts',(39.8505167960037,253.75,29.9589677074491)) ;
#102115=CARTESIAN_POINT('Ctrl Pts',(39.8499397253402,253.75,29.9595053771295)) ;
#102116=CARTESIAN_POINT('Ctrl Pts',(39.849362606764,253.750003330105,29.9600430036272)) ;
#102117=CARTESIAN_POINT('Ctrl Pts',(39.8339123904279,253.750181671152,29.9744336161108)) ;
#102118=CARTESIAN_POINT('Ctrl Pts',(39.8189533892428,253.752566842487,29.9883070896973)) ;
#102119=CARTESIAN_POINT('Ctrl Pts',(39.7905380911752,253.761740190968,30.0145549995742)) ;
#102120=CARTESIAN_POINT('Ctrl Pts',(39.7769188845312,253.768377217198,30.0270844220837)) ;
#102121=CARTESIAN_POINT('Ctrl Pts',(39.7501412146258,253.78721321578,30.0516371458428)) ;
#102122=CARTESIAN_POINT('Ctrl Pts',(39.7370754538178,253.800023548159,30.0635653016335)) ;
#102123=CARTESIAN_POINT('Ctrl Pts',(39.7180779384581,253.828041657271,30.0808650678764)) ;
#102124=CARTESIAN_POINT('Ctrl Pts',(39.7112763996935,253.841958224525,30.087041829166)) ;
#102125=CARTESIAN_POINT('Ctrl Pts',(39.7026699639647,253.870954690135,30.0948515246968)) ;
#102126=CARTESIAN_POINT('Ctrl Pts',(39.7005167960037,253.885320776746,30.096802244712)) ;
#102127=CARTESIAN_POINT('Ctrl Pts',(39.7005167960037,253.9,30.096802244712)) ;
#102128=CARTESIAN_POINT('Origin',(40.2,253.9,25.0213203435596)) ;
#102129=CARTESIAN_POINT('Origin',(39.8505167960037,253.9,27.759956707196)) ;
#102130=CARTESIAN_POINT('',(39.8505167960037,253.75,30.5023074499214)) ;
#102131=CARTESIAN_POINT('',(39.8505167960037,253.75,27.759956707196)) ;
#102132=CARTESIAN_POINT('',(39.7005167960037,253.9,30.4985930708324)) ;
#102133=CARTESIAN_POINT('Ctrl Pts',(39.8505167960037,253.75,30.5023074499214)) ;
#102134=CARTESIAN_POINT('Ctrl Pts',(39.8490586726999,253.75,30.5022678161701)) ;
#102135=CARTESIAN_POINT('Ctrl Pts',(39.8476006233589,253.750021261236,30.5022283083714)) ;
#102136=CARTESIAN_POINT('Ctrl Pts',(39.8461431129253,253.750063777237,30.5021889366963)) ;
#102137=CARTESIAN_POINT('Ctrl Pts',(39.8274188890355,253.750609968276,30.5016831399336)) ;
#102138=CARTESIAN_POINT('Ctrl Pts',(39.8089607261724,253.754658837467,30.5012049258669)) ;
#102139=CARTESIAN_POINT('Ctrl Pts',(39.7917256812164,253.762001431812,30.5007714713078)) ;
#102140=CARTESIAN_POINT('Ctrl Pts',(39.7737581677139,253.769656077527,30.5003195954547)) ;
#102141=CARTESIAN_POINT('Ctrl Pts',(39.757456249043,253.78074710398,30.49992447295)) ;
#102142=CARTESIAN_POINT('Ctrl Pts',(39.7437381135436,253.794651469056,30.4995981034064)) ;
#102143=CARTESIAN_POINT('Ctrl Pts',(39.7300236484415,253.808552113907,30.4992718211856)) ;
#102144=CARTESIAN_POINT('Ctrl Pts',(39.7191539711575,253.824998688613,30.4990202369966)) ;
#102145=CARTESIAN_POINT('Ctrl Pts',(39.7117415393002,253.843066458683,30.4988497601076)) ;
#102146=CARTESIAN_POINT('Ctrl Pts',(39.704330020872,253.861132002274,30.4986793042264)) ;
#102147=CARTESIAN_POINT('Ctrl Pts',(39.7005167960037,253.880472526098,30.4985930708322)) ;
#102148=CARTESIAN_POINT('Ctrl Pts',(39.7005167960037,253.9,30.4985930708322)) ;
#102149=CARTESIAN_POINT('',(39.7005167960037,253.9,27.759956707196)) ;
#102150=CARTESIAN_POINT('Origin',(40.2,253.9,30.5213203435596)) ;
#102151=CARTESIAN_POINT('',(40.5494832039963,253.75,30.5023074499214)) ;
#102152=CARTESIAN_POINT('Origin',(40.2,253.75,30.5213203435596)) ;
#102153=CARTESIAN_POINT('',(40.6994832039963,253.9,30.4985930708324)) ;
#102154=CARTESIAN_POINT('Ctrl Pts',(40.5494832039964,253.75,30.5023074499214)) ;
#102155=CARTESIAN_POINT('Ctrl Pts',(40.5509413273002,253.75,30.5022678161702)) ;
#102156=CARTESIAN_POINT('Ctrl Pts',(40.5523993766411,253.750021261236,30.5022283083715)) ;
#102157=CARTESIAN_POINT('Ctrl Pts',(40.5538568870747,253.750063777237,30.5021889366964)) ;
#102158=CARTESIAN_POINT('Ctrl Pts',(40.5725811109645,253.750609968276,30.5016831399329)) ;
#102159=CARTESIAN_POINT('Ctrl Pts',(40.5910392738275,253.754658837467,30.5012049258645)) ;
#102160=CARTESIAN_POINT('Ctrl Pts',(40.6082743187836,253.762001431812,30.500771471306)) ;
#102161=CARTESIAN_POINT('Ctrl Pts',(40.6262418322859,253.769656077527,30.5003195954534)) ;
#102162=CARTESIAN_POINT('Ctrl Pts',(40.642543750957,253.78074710398,30.4999244729504)) ;
#102163=CARTESIAN_POINT('Ctrl Pts',(40.6562618864565,253.794651469056,30.4995981034069)) ;
#102164=CARTESIAN_POINT('Ctrl Pts',(40.6699763515586,253.808552113907,30.4992718211861)) ;
#102165=CARTESIAN_POINT('Ctrl Pts',(40.6808460288425,253.824998688613,30.4990202369969)) ;
#102166=CARTESIAN_POINT('Ctrl Pts',(40.6882584606999,253.843066458683,30.4988497601079)) ;
#102167=CARTESIAN_POINT('Ctrl Pts',(40.695669979128,253.861132002274,30.4986793042266)) ;
#102168=CARTESIAN_POINT('Ctrl Pts',(40.6994832039963,253.880472526098,30.4985930708323)) ;
#102169=CARTESIAN_POINT('Ctrl Pts',(40.6994832039963,253.9,30.4985930708323)) ;
#102170=CARTESIAN_POINT('Origin',(40.2,253.9,30.5213203435596)) ;
#102171=CARTESIAN_POINT('Origin',(40.5494832039963,253.9,27.4082910455649)) ;
#102172=CARTESIAN_POINT('',(40.5494832039963,253.75,29.9589677074491)) ;
#102173=CARTESIAN_POINT('',(40.5494832039963,253.75,27.4082910455649)) ;
#102174=CARTESIAN_POINT('',(40.6994832039963,253.9,30.096802244712)) ;
#102175=CARTESIAN_POINT('Ctrl Pts',(40.5494832039963,253.75,29.9589677074491)) ;
#102176=CARTESIAN_POINT('Ctrl Pts',(40.5500602746609,253.75,29.9595053771305)) ;
#102177=CARTESIAN_POINT('Ctrl Pts',(40.5506373932381,253.750003330106,29.9600430036291)) ;
#102178=CARTESIAN_POINT('Ctrl Pts',(40.5660876095744,253.750181671152,29.974433616113)) ;
#102179=CARTESIAN_POINT('Ctrl Pts',(40.5810466107592,253.752566842488,29.9883070896991)) ;
#102180=CARTESIAN_POINT('Ctrl Pts',(40.6094619088257,253.761740190968,30.014554999575)) ;
#102181=CARTESIAN_POINT('Ctrl Pts',(40.6230811154693,253.768377217198,30.027084422084)) ;
#102182=CARTESIAN_POINT('Ctrl Pts',(40.6498587853742,253.78721321578,30.0516371458428)) ;
#102183=CARTESIAN_POINT('Ctrl Pts',(40.6629245461822,253.800023548159,30.0635653016335)) ;
#102184=CARTESIAN_POINT('Ctrl Pts',(40.681922061542,253.828041657271,30.0808650678764)) ;
#102185=CARTESIAN_POINT('Ctrl Pts',(40.6887236003065,253.841958224525,30.087041829166)) ;
#102186=CARTESIAN_POINT('Ctrl Pts',(40.6973300360353,253.870954690135,30.0948515246968)) ;
#102187=CARTESIAN_POINT('Ctrl Pts',(40.6994832039963,253.885320776746,30.096802244712)) ;
#102188=CARTESIAN_POINT('Ctrl Pts',(40.6994832039963,253.9,30.096802244712)) ;
#102189=CARTESIAN_POINT('',(40.6994832039963,253.9,27.4082910455649)) ;
#102190=CARTESIAN_POINT('Origin',(40.2,253.9,25.0213203435596)) ;
#102191=CARTESIAN_POINT('',(41.3934386691762,253.75,29.8252982934377)) ;
#102192=CARTESIAN_POINT('Origin',(40.2,253.75,25.0213203435596)) ;
#102193=CARTESIAN_POINT('',(41.293373406158,253.9,30.0027392774284)) ;
#102194=CARTESIAN_POINT('Ctrl Pts',(41.3934386691762,253.75,29.8252982934377)) ;
#102195=CARTESIAN_POINT('Ctrl Pts',(41.3930559914298,253.75,29.8259879723329)) ;
#102196=CARTESIAN_POINT('Ctrl Pts',(41.3926732547717,253.750003330105,29.8266776249647)) ;
#102197=CARTESIAN_POINT('Ctrl Pts',(41.3824261696638,253.750181671152,29.8451382901554)) ;
#102198=CARTESIAN_POINT('Ctrl Pts',(41.3724864532188,253.752566842487,29.8629553331985)) ;
#102199=CARTESIAN_POINT('Ctrl Pts',(41.3535729490481,253.761740190968,29.896699388929)) ;
#102200=CARTESIAN_POINT('Ctrl Pts',(41.3444921183076,253.768377217198,29.912824144155)) ;
#102201=CARTESIAN_POINT('Ctrl Pts',(41.3266122497526,253.78721321578,29.9444499271496)) ;
#102202=CARTESIAN_POINT('Ctrl Pts',(41.3178719756467,253.800023548159,29.9598318195758)) ;
#102203=CARTESIAN_POINT('Ctrl Pts',(41.3051501866382,253.828041657271,29.9821554300886)) ;
#102204=CARTESIAN_POINT('Ctrl Pts',(41.300590263084,253.841958224525,29.9901316702288)) ;
#102205=CARTESIAN_POINT('Ctrl Pts',(41.294818384942,253.870954690135,30.0002186669547)) ;
#102206=CARTESIAN_POINT('Ctrl Pts',(41.293373406158,253.885320776746,30.0027392774284)) ;
#102207=CARTESIAN_POINT('Ctrl Pts',(41.293373406158,253.9,30.0027392774284)) ;
#102208=CARTESIAN_POINT('Origin',(40.2,253.9,25.0213203435596)) ;
#102209=CARTESIAN_POINT('Origin',(40.7139068992805,253.9,27.7339145522423)) ;
#102210=CARTESIAN_POINT('',(41.5613398833194,253.75,30.342045096078)) ;
#102211=CARTESIAN_POINT('',(40.7139068992805,253.75,27.7339145522423)) ;
#102212=CARTESIAN_POINT('',(41.4175335996131,253.9,30.3848650607978)) ;
#102213=CARTESIAN_POINT('Ctrl Pts',(41.5613398833194,253.75,30.342045096078)) ;
#102214=CARTESIAN_POINT('Ctrl Pts',(41.559940878147,253.75,30.3424579870215)) ;
#102215=CARTESIAN_POINT('Ctrl Pts',(41.558541982239,253.750021261236,30.3428709748967)) ;
#102216=CARTESIAN_POINT('Ctrl Pts',(41.5571436409268,253.750063777237,30.3432839257022)) ;
#102217=CARTESIAN_POINT('Ctrl Pts',(41.5391795459883,253.750609968276,30.3485889877849)) ;
#102218=CARTESIAN_POINT('Ctrl Pts',(41.521477013645,253.754658837467,30.3538380651887)) ;
#102219=CARTESIAN_POINT('Ctrl Pts',(41.504951567006,253.762001431812,30.3587517471961)) ;
#102220=CARTESIAN_POINT('Ctrl Pts',(41.4877238088899,253.769656077527,30.3638742547405)) ;
#102221=CARTESIAN_POINT('Ctrl Pts',(41.472097663341,253.78074710398,30.368536040818)) ;
#102222=CARTESIAN_POINT('Ctrl Pts',(41.4589500874475,253.794651469056,30.3724647819372)) ;
#102223=CARTESIAN_POINT('Ctrl Pts',(41.4458060292934,253.808552113907,30.3763924718902)) ;
#102224=CARTESIAN_POINT('Ctrl Pts',(41.4353906080926,253.824998688613,30.3795121161121)) ;
#102225=CARTESIAN_POINT('Ctrl Pts',(41.4282882862172,253.843066458683,30.3816405503694)) ;
#102226=CARTESIAN_POINT('Ctrl Pts',(41.4211868395563,253.861132002274,30.3837687223411)) ;
#102227=CARTESIAN_POINT('Ctrl Pts',(41.4175335996131,253.880472526098,30.3848650607977)) ;
#102228=CARTESIAN_POINT('Ctrl Pts',(41.4175335996131,253.9,30.3848650607977)) ;
#102229=CARTESIAN_POINT('',(40.5712484218362,253.9,27.7802671013986)) ;
#102230=CARTESIAN_POINT('Origin',(41.8995934690622,253.9,30.252131183183)) ;
#102231=CARTESIAN_POINT('',(42.2260964403122,253.75,30.1260525975114)) ;
#102232=CARTESIAN_POINT('Origin',(41.8995934690622,253.75,30.252131183183)) ;
#102233=CARTESIAN_POINT('',(42.3676071114944,253.9,30.0761674639184)) ;
#102234=CARTESIAN_POINT('Ctrl Pts',(42.2260964403122,253.75,30.1260525975113)) ;
#102235=CARTESIAN_POINT('Ctrl Pts',(42.2274709504791,253.75,30.1255643186932)) ;
#102236=CARTESIAN_POINT('Ctrl Pts',(42.2288454292249,253.750021261236,30.1250761825188)) ;
#102237=CARTESIAN_POINT('Ctrl Pts',(42.2302194375035,253.750063777237,30.1245883423371)) ;
#102238=CARTESIAN_POINT('Ctrl Pts',(42.24787093285,253.750609968276,30.1183211976397)) ;
#102239=CARTESIAN_POINT('Ctrl Pts',(42.2652779126467,253.754658837467,30.112162503026)) ;
#102240=CARTESIAN_POINT('Ctrl Pts',(42.2815354696359,253.762001431812,30.1064243414531)) ;
#102241=CARTESIAN_POINT('Ctrl Pts',(42.298483953116,253.769656077527,30.1004423149599)) ;
#102242=CARTESIAN_POINT('Ctrl Pts',(42.3138658995278,253.78074710398,30.095028961218)) ;
#102243=CARTESIAN_POINT('Ctrl Pts',(42.3268117679506,253.794651469056,30.0904794283365)) ;
#102244=CARTESIAN_POINT('Ctrl Pts',(42.3397541726023,253.808552113907,30.085931112719)) ;
#102245=CARTESIAN_POINT('Ctrl Pts',(42.3500141062232,253.824998688613,30.0823329269323)) ;
#102246=CARTESIAN_POINT('Ctrl Pts',(42.3570110675869,253.843066458683,30.0798802263626)) ;
#102247=CARTESIAN_POINT('Ctrl Pts',(42.3640071667196,253.861132002274,30.0774278280376)) ;
#102248=CARTESIAN_POINT('Ctrl Pts',(42.3676071114944,253.880472526098,30.0761674639185)) ;
#102249=CARTESIAN_POINT('Ctrl Pts',(42.3676071114944,253.9,30.0761674639186)) ;
#102250=CARTESIAN_POINT('Origin',(41.8995934690622,253.9,30.252131183183)) ;
#102251=CARTESIAN_POINT('Origin',(41.2699927904911,253.9,27.1834681346239)) ;
#102252=CARTESIAN_POINT('',(42.0581952261689,253.75,29.6093057948708)) ;
#102253=CARTESIAN_POINT('',(41.2699927904911,253.75,27.1834681346239)) ;
#102254=CARTESIAN_POINT('',(42.2434469180392,253.9,29.694041680549)) ;
#102255=CARTESIAN_POINT('Ctrl Pts',(42.0581952261689,253.75,29.6093057948708)) ;
#102256=CARTESIAN_POINT('Ctrl Pts',(42.0589102020537,253.75,29.6096388244826)) ;
#102257=CARTESIAN_POINT('Ctrl Pts',(42.059625210162,253.750003330106,29.6099717982194)) ;
#102258=CARTESIAN_POINT('Ctrl Pts',(42.0787661829038,253.750181671152,29.6188837045809)) ;
#102259=CARTESIAN_POINT('Ctrl Pts',(42.0972801775669,253.752566842488,29.6274555764536)) ;
#102260=CARTESIAN_POINT('Ctrl Pts',(42.1324157821739,253.761740190968,29.6436380121774)) ;
#102261=CARTESIAN_POINT('Ctrl Pts',(42.1492402218841,253.768377217198,29.6513456347973)) ;
#102262=CARTESIAN_POINT('Ctrl Pts',(42.1822945082382,253.78721321578,29.6664219076506)) ;
#102263=CARTESIAN_POINT('Ctrl Pts',(42.1984067880458,253.800023548159,29.6737287158085)) ;
#102264=CARTESIAN_POINT('Ctrl Pts',(42.2218204205898,253.828041657271,29.6843112161272)) ;
#102265=CARTESIAN_POINT('Ctrl Pts',(42.2301977925614,253.841958224525,29.6880838741351)) ;
#102266=CARTESIAN_POINT('Ctrl Pts',(42.2407963279832,253.870954690135,29.6928518010587)) ;
#102267=CARTESIAN_POINT('Ctrl Pts',(42.2434469180392,253.885320776746,29.694041680549)) ;
#102268=CARTESIAN_POINT('Ctrl Pts',(42.2434469180392,253.9,29.694041680549)) ;
#102269=CARTESIAN_POINT('',(41.4126512679354,253.9,27.1371155854676)) ;
#102270=CARTESIAN_POINT('Origin',(40.2,253.9,25.0213203435596)) ;
#102271=CARTESIAN_POINT('',(42.8195384502335,253.75,29.2213820464098)) ;
#102272=CARTESIAN_POINT('Origin',(40.2,253.75,25.0213203435596)) ;
#102273=CARTESIAN_POINT('',(42.7792030093369,253.9,29.4210603173112)) ;
#102274=CARTESIAN_POINT('Ctrl Pts',(42.8195384502335,253.75,29.2213820464098)) ;
#102275=CARTESIAN_POINT('Ctrl Pts',(42.8193876245675,253.75,29.222156223949)) ;
#102276=CARTESIAN_POINT('Ctrl Pts',(42.8192367347585,253.750003330105,29.2229303947088)) ;
#102277=CARTESIAN_POINT('Ctrl Pts',(42.8151958369642,253.750181671152,29.2436540540784)) ;
#102278=CARTESIAN_POINT('Ctrl Pts',(42.8112483739592,253.752566842488,29.2636706102647)) ;
#102279=CARTESIAN_POINT('Ctrl Pts',(42.8036880492521,253.761740190969,29.3016077085626)) ;
#102280=CARTESIAN_POINT('Ctrl Pts',(42.8000344893982,253.768377217198,29.3197493931144)) ;
#102281=CARTESIAN_POINT('Ctrl Pts',(42.7928026283045,253.78721321578,29.3553524833538)) ;
#102282=CARTESIAN_POINT('Ctrl Pts',(42.7892433998272,253.800023548159,29.3726824256129)) ;
#102283=CARTESIAN_POINT('Ctrl Pts',(42.784042634516,253.828041657271,29.3978446898607)) ;
#102284=CARTESIAN_POINT('Ctrl Pts',(42.7821706832604,253.841958224525,29.4068396388929)) ;
#102285=CARTESIAN_POINT('Ctrl Pts',(42.7797983543528,253.870954690135,29.4182165512944)) ;
#102286=CARTESIAN_POINT('Ctrl Pts',(42.7792030093369,253.885320776746,29.4210603173112)) ;
#102287=CARTESIAN_POINT('Ctrl Pts',(42.7792030093369,253.9,29.4210603173112)) ;
#102288=CARTESIAN_POINT('Origin',(40.2,253.9,25.0213203435596)) ;
#102289=CARTESIAN_POINT('Origin',(41.5269922146558,253.9,27.4423447763876)) ;
#102290=CARTESIAN_POINT('',(43.1389055378431,253.75,29.6609531317893)) ;
#102291=CARTESIAN_POINT('',(41.5269922146558,253.75,27.4423447763876)) ;
#102292=CARTESIAN_POINT('',(43.0153697314369,253.9,29.7461159238265)) ;
#102293=CARTESIAN_POINT('Ctrl Pts',(43.1389055378431,253.75,29.6609531317893)) ;
#102294=CARTESIAN_POINT('Ctrl Pts',(43.1377025951759,253.75,29.661778130785)) ;
#102295=CARTESIAN_POINT('Ctrl Pts',(43.1364997863788,253.750021261236,29.6626031882036)) ;
#102296=CARTESIAN_POINT('Ctrl Pts',(43.1352974935786,253.750063777237,29.6634280389876)) ;
#102297=CARTESIAN_POINT('Ctrl Pts',(43.1198519783685,253.750609968276,29.6740246634766)) ;
#102298=CARTESIAN_POINT('Ctrl Pts',(43.1046379237495,253.754658837467,29.6844872160813)) ;
#102299=CARTESIAN_POINT('Ctrl Pts',(43.0904397012843,253.762001431812,29.6942670492247)) ;
#102300=CARTESIAN_POINT('Ctrl Pts',(43.0756380715522,253.769656077527,29.7044625134375)) ;
#102301=CARTESIAN_POINT('Ctrl Pts',(43.0622172951262,253.78074710398,29.7137248799966)) ;
#102302=CARTESIAN_POINT('Ctrl Pts',(43.0509272551715,253.794651469056,29.7215241592249)) ;
#102303=CARTESIAN_POINT('Ctrl Pts',(43.0396402359576,253.808552113907,29.7293213516934)) ;
#102304=CARTESIAN_POINT('Ctrl Pts',(43.0306986048354,253.824998688613,29.7355068518135)) ;
#102305=CARTESIAN_POINT('Ctrl Pts',(43.0246016176919,253.843066458683,29.7397258512424)) ;
#102306=CARTESIAN_POINT('Ctrl Pts',(43.0185053818762,253.861132002274,29.7439443307668)) ;
#102307=CARTESIAN_POINT('Ctrl Pts',(43.0153697314371,253.880472526098,29.7461159238268)) ;
#102308=CARTESIAN_POINT('Ctrl Pts',(43.015369731437,253.9,29.7461159238267)) ;
#102309=CARTESIAN_POINT('',(41.4056396654995,253.9,27.5305125642315)) ;
#102310=CARTESIAN_POINT('Origin',(43.4328188876086,253.9,29.4709138126218)) ;
#102311=CARTESIAN_POINT('',(43.7043812404062,253.75,29.2501109853232)) ;
#102312=CARTESIAN_POINT('Origin',(43.4328188876086,253.75,29.4709138126218)) ;
#102313=CARTESIAN_POINT('',(43.8235505323126,253.9,29.1589382016729)) ;
#102314=CARTESIAN_POINT('Ctrl Pts',(43.7043812404062,253.75,29.2501109853232)) ;
#102315=CARTESIAN_POINT('Ctrl Pts',(43.7055375908048,253.75,29.2492218575706)) ;
#102316=CARTESIAN_POINT('Ctrl Pts',(43.7066939553966,253.750021261236,29.2483328751888)) ;
#102317=CARTESIAN_POINT('Ctrl Pts',(43.7078499640179,253.750063777237,29.2474443196972)) ;
#102318=CARTESIAN_POINT('Ctrl Pts',(43.7227008794821,253.750609968276,29.2360292988668)) ;
#102319=CARTESIAN_POINT('Ctrl Pts',(43.7373527597389,253.754658837467,29.2247929796351)) ;
#102320=CARTESIAN_POINT('Ctrl Pts',(43.7510414258099,253.762001431812,29.2143118022833)) ;
#102321=CARTESIAN_POINT('Ctrl Pts',(43.7653118436181,253.769656077527,29.2033851875821)) ;
#102322=CARTESIAN_POINT('Ctrl Pts',(43.7782681256832,253.78074710398,29.1934834993827)) ;
#102323=CARTESIAN_POINT('Ctrl Pts',(43.7891744952288,253.794651469056,29.18515614314)) ;
#102324=CARTESIAN_POINT('Ctrl Pts',(43.8000779466878,253.808552113907,29.1768310149483)) ;
#102325=CARTESIAN_POINT('Ctrl Pts',(43.808723822858,253.824998688613,29.1702384430595)) ;
#102326=CARTESIAN_POINT('Ctrl Pts',(43.8146204023989,253.843066458683,29.1657436062296)) ;
#102327=CARTESIAN_POINT('Ctrl Pts',(43.8205162553081,253.861132002274,29.1612493232955)) ;
#102328=CARTESIAN_POINT('Ctrl Pts',(43.8235505323127,253.880472526098,29.1589382016731)) ;
#102329=CARTESIAN_POINT('Ctrl Pts',(43.8235505323126,253.9,29.1589382016729)) ;
#102330=CARTESIAN_POINT('Origin',(43.4328188876086,253.9,29.4709138126218)) ;
#102331=CARTESIAN_POINT('Origin',(41.8857640275745,253.9,26.746999133324)) ;
#102332=CARTESIAN_POINT('',(43.3850141527966,253.75,28.8105398999439)) ;
#102333=CARTESIAN_POINT('',(41.8857640275745,253.75,26.746999133324)) ;
#102334=CARTESIAN_POINT('',(43.5873838102126,253.9,28.8338825951576)) ;
#102335=CARTESIAN_POINT('Ctrl Pts',(43.3850141527966,253.75,28.8105398999439)) ;
#102336=CARTESIAN_POINT('Ctrl Pts',(43.3857970470792,253.75,28.8106356902272)) ;
#102337=CARTESIAN_POINT('Ctrl Pts',(43.3865799547416,253.750003330105,28.8107314174126)) ;
#102338=CARTESIAN_POINT('Ctrl Pts',(43.4075380321148,253.750181671152,28.8132922581638)) ;
#102339=CARTESIAN_POINT('Ctrl Pts',(43.4277947414637,253.752566842487,28.815723453781)) ;
#102340=CARTESIAN_POINT('Ctrl Pts',(43.4662113348296,253.761740190968,28.8202563657946)) ;
#102341=CARTESIAN_POINT('Ctrl Pts',(43.4845941142253,253.768377217198,28.8223877127212)) ;
#102342=CARTESIAN_POINT('Ctrl Pts',(43.5206894331777,253.78721321578,28.8265117640394)) ;
#102343=CARTESIAN_POINT('Ctrl Pts',(43.5382710497767,253.800023548159,28.8284819832727)) ;
#102344=CARTESIAN_POINT('Ctrl Pts',(43.5638089100193,253.828041657271,28.8313113288033)) ;
#102345=CARTESIAN_POINT('Ctrl Pts',(43.5729420796607,253.841958224525,28.832310589478)) ;
#102346=CARTESIAN_POINT('Ctrl Pts',(43.584495256284,253.870954690135,28.8335700298871)) ;
#102347=CARTESIAN_POINT('Ctrl Pts',(43.5873838102126,253.885320776746,28.8338825951576)) ;
#102348=CARTESIAN_POINT('Ctrl Pts',(43.5873838102126,253.9,28.8338825951576)) ;
#102349=CARTESIAN_POINT('',(42.0071165767308,253.9,26.6588313454802)) ;
#102350=CARTESIAN_POINT('Origin',(40.2,253.9,25.0213203435596)) ;
#102351=CARTESIAN_POINT('',(43.9892195563843,253.75,28.2063344963563)) ;
#102352=CARTESIAN_POINT('Origin',(40.2,253.75,25.0213203435596)) ;
#102353=CARTESIAN_POINT('',(44.012562251598,253.9,28.4087041537722)) ;
#102354=CARTESIAN_POINT('Ctrl Pts',(43.9892195563843,253.75,28.2063344963563)) ;
#102355=CARTESIAN_POINT('Ctrl Pts',(43.9893153466677,253.75,28.2071173906402)) ;
#102356=CARTESIAN_POINT('Ctrl Pts',(43.9894110738533,253.750003330106,28.2079002983041)) ;
#102357=CARTESIAN_POINT('Ctrl Pts',(43.9919719146048,253.750181671152,28.2288583756769)) ;
#102358=CARTESIAN_POINT('Ctrl Pts',(43.9944031102216,253.752566842488,28.2491150850258)) ;
#102359=CARTESIAN_POINT('Ctrl Pts',(43.9989360222351,253.761740190968,28.2875316783904)) ;
#102360=CARTESIAN_POINT('Ctrl Pts',(44.0010673691616,253.768377217198,28.3059144577855)) ;
#102361=CARTESIAN_POINT('Ctrl Pts',(44.0051914204798,253.78721321578,28.3420097767375)) ;
#102362=CARTESIAN_POINT('Ctrl Pts',(44.0071616397131,253.800023548159,28.3595913933363)) ;
#102363=CARTESIAN_POINT('Ctrl Pts',(44.0099909852436,253.828041657271,28.3851292535788)) ;
#102364=CARTESIAN_POINT('Ctrl Pts',(44.0109902459184,253.841958224525,28.3942624232203)) ;
#102365=CARTESIAN_POINT('Ctrl Pts',(44.0122496863275,253.870954690135,28.4058155998437)) ;
#102366=CARTESIAN_POINT('Ctrl Pts',(44.012562251598,253.885320776746,28.4087041537722)) ;
#102367=CARTESIAN_POINT('Ctrl Pts',(44.012562251598,253.9,28.4087041537722)) ;
#102368=CARTESIAN_POINT('Origin',(40.2,253.9,25.0213203435596)) ;
#102369=CARTESIAN_POINT('Origin',(42.2101822863621,253.9,26.9137882607786)) ;
#102370=CARTESIAN_POINT('',(44.4287906417639,253.75,28.5257015839661)) ;
#102371=CARTESIAN_POINT('',(42.2101822863621,253.75,26.9137882607786)) ;
#102372=CARTESIAN_POINT('',(44.3376178581133,253.9,28.6448708758722)) ;
#102373=CARTESIAN_POINT('Ctrl Pts',(44.4287906417639,253.75,28.5257015839661)) ;
#102374=CARTESIAN_POINT('Ctrl Pts',(44.4279015140116,253.75,28.5268579343644)) ;
#102375=CARTESIAN_POINT('Ctrl Pts',(44.4270125316306,253.750021261236,28.5280142989575)) ;
#102376=CARTESIAN_POINT('Ctrl Pts',(44.4261239761386,253.750063777237,28.5291703075782)) ;
#102377=CARTESIAN_POINT('Ctrl Pts',(44.4147089553012,253.750609968276,28.5440212230371)) ;
#102378=CARTESIAN_POINT('Ctrl Pts',(44.403472636075,253.754658837467,28.5586731032981)) ;
#102379=CARTESIAN_POINT('Ctrl Pts',(44.3929914587233,253.762001431812,28.5723617693692)) ;
#102380=CARTESIAN_POINT('Ctrl Pts',(44.3820648440222,253.769656077527,28.5866321871774)) ;
#102381=CARTESIAN_POINT('Ctrl Pts',(44.3721631558234,253.78074710398,28.5995884692429)) ;
#102382=CARTESIAN_POINT('Ctrl Pts',(44.3638357995806,253.794651469056,28.6104948387886)) ;
#102383=CARTESIAN_POINT('Ctrl Pts',(44.3555106713888,253.808552113907,28.6213982902475)) ;
#102384=CARTESIAN_POINT('Ctrl Pts',(44.3489180994998,253.824998688613,28.6300441664176)) ;
#102385=CARTESIAN_POINT('Ctrl Pts',(44.3444232626699,253.843066458683,28.6359407459585)) ;
#102386=CARTESIAN_POINT('Ctrl Pts',(44.3399289797359,253.861132002274,28.6418365988678)) ;
#102387=CARTESIAN_POINT('Ctrl Pts',(44.3376178581134,253.880472526098,28.6448708758723)) ;
#102388=CARTESIAN_POINT('Ctrl Pts',(44.3376178581134,253.9,28.6448708758723)) ;
#102389=CARTESIAN_POINT('',(42.1220144985182,253.9,27.0351408099348)) ;
#102390=CARTESIAN_POINT('Origin',(44.6495934690622,253.9,28.2541392311682)) ;
#102391=CARTESIAN_POINT('',(44.8396327882296,253.75,27.9602258814027)) ;
#102392=CARTESIAN_POINT('Origin',(44.6495934690622,253.75,28.2541392311682)) ;
#102393=CARTESIAN_POINT('',(44.9247955802669,253.9,27.8366900749965)) ;
#102394=CARTESIAN_POINT('Ctrl Pts',(44.8396327882335,253.75,27.9602258813973)) ;
#102395=CARTESIAN_POINT('Ctrl Pts',(44.8404577872282,253.75,27.9590229387317)) ;
#102396=CARTESIAN_POINT('Ctrl Pts',(44.841282844644,253.750021261236,27.957820129936)) ;
#102397=CARTESIAN_POINT('Ctrl Pts',(44.8421076954273,253.750063777237,27.9566178371377)) ;
#102398=CARTESIAN_POINT('Ctrl Pts',(44.8527043199225,253.750609968276,27.9411723219304)) ;
#102399=CARTESIAN_POINT('Ctrl Pts',(44.8631668725218,253.754658837467,27.9259582673091)) ;
#102400=CARTESIAN_POINT('Ctrl Pts',(44.8729467056653,253.762001431812,27.911760044844)) ;
#102401=CARTESIAN_POINT('Ctrl Pts',(44.8831421698783,253.769656077527,27.8969584151118)) ;
#102402=CARTESIAN_POINT('Ctrl Pts',(44.8924045364365,253.78074710398,27.8835376386854)) ;
#102403=CARTESIAN_POINT('Ctrl Pts',(44.9002038156648,253.794651469056,27.8722475987308)) ;
#102404=CARTESIAN_POINT('Ctrl Pts',(44.9080010081334,253.808552113907,27.8609605795169)) ;
#102405=CARTESIAN_POINT('Ctrl Pts',(44.9141865082541,253.824998688613,27.8520189483951)) ;
#102406=CARTESIAN_POINT('Ctrl Pts',(44.918405507683,253.843066458683,27.8459219612516)) ;
#102407=CARTESIAN_POINT('Ctrl Pts',(44.9226239872073,253.861132002274,27.8398257254358)) ;
#102408=CARTESIAN_POINT('Ctrl Pts',(44.9247955802671,253.880472526098,27.8366900749966)) ;
#102409=CARTESIAN_POINT('Ctrl Pts',(44.924795580267,253.9,27.8366900749965)) ;
#102410=CARTESIAN_POINT('Origin',(44.6495934690622,253.9,28.2541392311682)) ;
#102411=CARTESIAN_POINT('Origin',(42.3365209362303,253.9,26.1416086685709)) ;
#102412=CARTESIAN_POINT('',(44.4000617028502,253.75,27.6408587937931)) ;
#102413=CARTESIAN_POINT('',(42.3365209362303,253.75,26.1416086685709)) ;
#102414=CARTESIAN_POINT('',(44.5997399737516,253.9,27.6005233528965)) ;
#102415=CARTESIAN_POINT('Ctrl Pts',(44.4000617028502,253.75,27.6408587937931)) ;
#102416=CARTESIAN_POINT('Ctrl Pts',(44.4008358803894,253.75,27.6407079681271)) ;
#102417=CARTESIAN_POINT('Ctrl Pts',(44.4016100511492,253.750003330105,27.6405570783181)) ;
#102418=CARTESIAN_POINT('Ctrl Pts',(44.4223337105192,253.750181671152,27.6365161805235)) ;
#102419=CARTESIAN_POINT('Ctrl Pts',(44.4423502667051,253.752566842488,27.6325687175188)) ;
#102420=CARTESIAN_POINT('Ctrl Pts',(44.480287365003,253.761740190969,27.6250083928117)) ;
#102421=CARTESIAN_POINT('Ctrl Pts',(44.4984290495548,253.768377217198,27.6213548329578)) ;
#102422=CARTESIAN_POINT('Ctrl Pts',(44.5340321397943,253.78721321578,27.6141229718641)) ;
#102423=CARTESIAN_POINT('Ctrl Pts',(44.5513620820533,253.800023548159,27.6105637433868)) ;
#102424=CARTESIAN_POINT('Ctrl Pts',(44.5765243463011,253.828041657271,27.6053629780756)) ;
#102425=CARTESIAN_POINT('Ctrl Pts',(44.5855192953333,253.841958224525,27.6034910268201)) ;
#102426=CARTESIAN_POINT('Ctrl Pts',(44.5968962077348,253.870954690135,27.6011186979124)) ;
#102427=CARTESIAN_POINT('Ctrl Pts',(44.5997399737516,253.885320776746,27.6005233528965)) ;
#102428=CARTESIAN_POINT('Ctrl Pts',(44.5997399737516,253.9,27.6005233528965)) ;
#102429=CARTESIAN_POINT('',(42.4246887240742,253.9,26.0202561194147)) ;
#102430=CARTESIAN_POINT('Origin',(40.2,253.9,25.0213203435596)) ;
#102431=CARTESIAN_POINT('',(44.7879854513112,253.75,26.8795155697285)) ;
#102432=CARTESIAN_POINT('Origin',(40.2,253.75,25.0213203435596)) ;
#102433=CARTESIAN_POINT('',(44.8727213369894,253.9,27.0647672615988)) ;
#102434=CARTESIAN_POINT('Ctrl Pts',(44.7879854513112,253.75,26.8795155697285)) ;
#102435=CARTESIAN_POINT('Ctrl Pts',(44.788318480923,253.75,26.8802305456133)) ;
#102436=CARTESIAN_POINT('Ctrl Pts',(44.7886514546598,253.750003330106,26.8809455537216)) ;
#102437=CARTESIAN_POINT('Ctrl Pts',(44.7975633610213,253.750181671152,26.9000865264628)) ;
#102438=CARTESIAN_POINT('Ctrl Pts',(44.806135232894,253.752566842488,26.9186005211264)) ;
#102439=CARTESIAN_POINT('Ctrl Pts',(44.8223176686178,253.761740190968,26.9537361257334)) ;
#102440=CARTESIAN_POINT('Ctrl Pts',(44.8300252912377,253.768377217198,26.9705605654437)) ;
#102441=CARTESIAN_POINT('Ctrl Pts',(44.845101564091,253.78721321578,27.0036148517979)) ;
#102442=CARTESIAN_POINT('Ctrl Pts',(44.8524083722489,253.800023548159,27.0197271316054)) ;
#102443=CARTESIAN_POINT('Ctrl Pts',(44.8629908725676,253.828041657271,27.0431407641494)) ;
#102444=CARTESIAN_POINT('Ctrl Pts',(44.8667635305755,253.841958224525,27.051518136121)) ;
#102445=CARTESIAN_POINT('Ctrl Pts',(44.8715314574991,253.870954690135,27.0621166715429)) ;
#102446=CARTESIAN_POINT('Ctrl Pts',(44.8727213369894,253.885320776746,27.0647672615988)) ;
#102447=CARTESIAN_POINT('Ctrl Pts',(44.8727213369894,253.9,27.0647672615988)) ;
#102448=CARTESIAN_POINT('Origin',(40.2,253.9,25.0213203435596)) ;
#102449=CARTESIAN_POINT('Origin',(42.6966017101158,253.9,26.1999837998328)) ;
#102450=CARTESIAN_POINT('',(45.3047322539518,253.75,27.0474167838718)) ;
#102451=CARTESIAN_POINT('',(42.6966017101158,253.75,26.1999837998328)) ;
#102452=CARTESIAN_POINT('',(45.2548471203588,253.9,27.188927455054)) ;
#102453=CARTESIAN_POINT('Ctrl Pts',(45.3047322539518,253.75,27.0474167838718)) ;
#102454=CARTESIAN_POINT('Ctrl Pts',(45.3042439751337,253.75,27.0487912940387)) ;
#102455=CARTESIAN_POINT('Ctrl Pts',(45.3037558389592,253.750021261236,27.0501657727844)) ;
#102456=CARTESIAN_POINT('Ctrl Pts',(45.3032679987773,253.750063777237,27.0515397810629)) ;
#102457=CARTESIAN_POINT('Ctrl Pts',(45.2970008540777,253.750609968276,27.0691912764083)) ;
#102458=CARTESIAN_POINT('Ctrl Pts',(45.2908421594672,253.754658837467,27.0865982562064)) ;
#102459=CARTESIAN_POINT('Ctrl Pts',(45.2851039978939,253.762001431812,27.1028558131956)) ;
#102460=CARTESIAN_POINT('Ctrl Pts',(45.2791219714003,253.769656077527,27.1198042966757)) ;
#102461=CARTESIAN_POINT('Ctrl Pts',(45.2737086176584,253.78074710398,27.1351862430874)) ;
#102462=CARTESIAN_POINT('Ctrl Pts',(45.2691590847767,253.794651469056,27.1481321115101)) ;
#102463=CARTESIAN_POINT('Ctrl Pts',(45.2646107691591,253.808552113907,27.1610745161618)) ;
#102464=CARTESIAN_POINT('Ctrl Pts',(45.2610125833728,253.824998688613,27.1713344497829)) ;
#102465=CARTESIAN_POINT('Ctrl Pts',(45.2585598828031,253.843066458683,27.1783314111466)) ;
#102466=CARTESIAN_POINT('Ctrl Pts',(45.2561074844782,253.861132002274,27.1853275102792)) ;
#102467=CARTESIAN_POINT('Ctrl Pts',(45.2548471203586,253.880472526098,27.1889274550539)) ;
#102468=CARTESIAN_POINT('Ctrl Pts',(45.2548471203588,253.9,27.1889274550539)) ;
#102469=CARTESIAN_POINT('',(42.6502491609595,253.9,26.3426422772771)) ;
#102470=CARTESIAN_POINT('Origin',(45.4308108396234,253.9,26.7209138126218)) ;
#102471=CARTESIAN_POINT('',(45.5207247525186,253.75,26.382660226879)) ;
#102472=CARTESIAN_POINT('Origin',(45.4308108396234,253.75,26.7209138126218)) ;
#102473=CARTESIAN_POINT('',(45.5635447172382,253.9,26.2388539431727)) ;
#102474=CARTESIAN_POINT('Ctrl Pts',(45.5207247525205,253.75,26.3826602268732)) ;
#102475=CARTESIAN_POINT('Ctrl Pts',(45.5211376434635,253.75,26.3812612217023)) ;
#102476=CARTESIAN_POINT('Ctrl Pts',(45.5215506313349,253.750021261236,26.3798623257963)) ;
#102477=CARTESIAN_POINT('Ctrl Pts',(45.521963582141,253.750063777237,26.3784639844859)) ;
#102478=CARTESIAN_POINT('Ctrl Pts',(45.5272686442386,253.750609968276,26.3604998895502)) ;
#102479=CARTESIAN_POINT('Ctrl Pts',(45.5325177216272,253.754658837467,26.3427973572037)) ;
#102480=CARTESIAN_POINT('Ctrl Pts',(45.5374314036352,253.762001431812,26.3262719105652)) ;
#102481=CARTESIAN_POINT('Ctrl Pts',(45.5425539111803,253.769656077527,26.3090441524495)) ;
#102482=CARTESIAN_POINT('Ctrl Pts',(45.5472156972587,253.78074710398,26.2934180069008)) ;
#102483=CARTESIAN_POINT('Ctrl Pts',(45.551144438378,253.794651469056,26.2802704310072)) ;
#102484=CARTESIAN_POINT('Ctrl Pts',(45.5550721283311,253.808552113907,26.2671263728531)) ;
#102485=CARTESIAN_POINT('Ctrl Pts',(45.5581917725533,253.824998688613,26.2567109516524)) ;
#102486=CARTESIAN_POINT('Ctrl Pts',(45.5603202068105,253.843066458683,26.249608629777)) ;
#102487=CARTESIAN_POINT('Ctrl Pts',(45.5624483787821,253.861132002274,26.2425071831161)) ;
#102488=CARTESIAN_POINT('Ctrl Pts',(45.5635447172386,253.880472526098,26.2388539431728)) ;
#102489=CARTESIAN_POINT('Ctrl Pts',(45.5635447172384,253.9,26.2388539431728)) ;
#102490=CARTESIAN_POINT('Origin',(45.4308108396234,253.9,26.7209138126218)) ;
#102491=CARTESIAN_POINT('Origin',(42.5781402896312,253.9,25.426556577058)) ;
#102492=CARTESIAN_POINT('',(45.0039779498781,253.75,26.2147590127358)) ;
#102493=CARTESIAN_POINT('',(42.5781402896312,253.75,25.426556577058)) ;
#102494=CARTESIAN_POINT('',(45.1814189338688,253.9,26.1146937497175)) ;
#102495=CARTESIAN_POINT('Ctrl Pts',(45.0039779498781,253.75,26.2147590127358)) ;
#102496=CARTESIAN_POINT('Ctrl Pts',(45.0046676287764,253.75,26.2143763349877)) ;
#102497=CARTESIAN_POINT('Ctrl Pts',(45.0053572814057,253.750003330105,26.213993598331)) ;
#102498=CARTESIAN_POINT('Ctrl Pts',(45.0238179465998,253.750181671152,26.2037465132207)) ;
#102499=CARTESIAN_POINT('Ctrl Pts',(45.0416349896415,253.752566842488,26.1938067967769)) ;
#102500=CARTESIAN_POINT('Ctrl Pts',(45.0753790453708,253.761740190968,26.1748932926068)) ;
#102501=CARTESIAN_POINT('Ctrl Pts',(45.0915038005961,253.768377217198,26.1658124618668)) ;
#102502=CARTESIAN_POINT('Ctrl Pts',(45.1231295835901,253.78721321578,26.1479325933121)) ;
#102503=CARTESIAN_POINT('Ctrl Pts',(45.1385114760162,253.800023548159,26.1391923192062)) ;
#102504=CARTESIAN_POINT('Ctrl Pts',(45.1608350865289,253.828041657271,26.1264705301978)) ;
#102505=CARTESIAN_POINT('Ctrl Pts',(45.1688113266691,253.841958224525,26.1219106066435)) ;
#102506=CARTESIAN_POINT('Ctrl Pts',(45.1788983233951,253.870954690135,26.1161387285016)) ;
#102507=CARTESIAN_POINT('Ctrl Pts',(45.1814189338688,253.885320776746,26.1146937497175)) ;
#102508=CARTESIAN_POINT('Ctrl Pts',(45.1814189338688,253.9,26.1146937497175)) ;
#102509=CARTESIAN_POINT('',(42.6244928387874,253.9,25.2838980996137)) ;
#102510=CARTESIAN_POINT('Origin',(40.2,253.9,25.0213203435596)) ;
#102511=CARTESIAN_POINT('',(45.1376473638895,253.75,25.3708035475559)) ;
#102512=CARTESIAN_POINT('Origin',(40.2,253.75,25.0213203435596)) ;
#102513=CARTESIAN_POINT('',(45.2754819011524,253.9,25.5208035475559)) ;
#102514=CARTESIAN_POINT('Ctrl Pts',(45.1376473638895,253.75,25.3708035475559)) ;
#102515=CARTESIAN_POINT('Ctrl Pts',(45.1381850335709,253.75,25.3713806182205)) ;
#102516=CARTESIAN_POINT('Ctrl Pts',(45.1387226600695,253.750003330106,25.3719577367977)) ;
#102517=CARTESIAN_POINT('Ctrl Pts',(45.1531132725536,253.750181671152,25.3874079531344)) ;
#102518=CARTESIAN_POINT('Ctrl Pts',(45.1669867461395,253.752566842488,25.4023669543188)) ;
#102519=CARTESIAN_POINT('Ctrl Pts',(45.1932346560153,253.761740190968,25.4307822523852)) ;
#102520=CARTESIAN_POINT('Ctrl Pts',(45.2057640785244,253.768377217198,25.4444014590288)) ;
#102521=CARTESIAN_POINT('Ctrl Pts',(45.2303168022832,253.78721321578,25.4711791289338)) ;
#102522=CARTESIAN_POINT('Ctrl Pts',(45.2422449580739,253.800023548158,25.4842448897418)) ;
#102523=CARTESIAN_POINT('Ctrl Pts',(45.2595447243168,253.828041657271,25.5032424051016)) ;
#102524=CARTESIAN_POINT('Ctrl Pts',(45.2657214856064,253.841958224525,25.5100439438662)) ;
#102525=CARTESIAN_POINT('Ctrl Pts',(45.2735311811371,253.870954690135,25.5186503795949)) ;
#102526=CARTESIAN_POINT('Ctrl Pts',(45.2754819011524,253.885320776746,25.5208035475559)) ;
#102527=CARTESIAN_POINT('Ctrl Pts',(45.2754819011524,253.9,25.5208035475559)) ;
#102528=CARTESIAN_POINT('Origin',(40.2,253.9,25.0213203435596)) ;
#102529=CARTESIAN_POINT('Origin',(42.9386363636364,253.9,25.3708035475559)) ;
#102530=CARTESIAN_POINT('',(45.6809871063618,253.75,25.3708035475559)) ;
#102531=CARTESIAN_POINT('',(42.9386363636364,253.75,25.3708035475559)) ;
#102532=CARTESIAN_POINT('',(45.6772727272728,253.9,25.5208035475559)) ;
#102533=CARTESIAN_POINT('Ctrl Pts',(45.6809871063618,253.75,25.3708035475559)) ;
#102534=CARTESIAN_POINT('Ctrl Pts',(45.6809474726106,253.75,25.3722616708597)) ;
#102535=CARTESIAN_POINT('Ctrl Pts',(45.6809079648117,253.750021261236,25.3737197202007)) ;
#102536=CARTESIAN_POINT('Ctrl Pts',(45.6808685931366,253.750063777237,25.3751772306343)) ;
#102537=CARTESIAN_POINT('Ctrl Pts',(45.6803627963739,253.750609968276,25.3939014545242)) ;
#102538=CARTESIAN_POINT('Ctrl Pts',(45.6798845823057,253.754658837467,25.4123596173872)) ;
#102539=CARTESIAN_POINT('Ctrl Pts',(45.679451127747,253.762001431812,25.4295946623432)) ;
#102540=CARTESIAN_POINT('Ctrl Pts',(45.6789992518942,253.769656077527,25.4475621758455)) ;
#102541=CARTESIAN_POINT('Ctrl Pts',(45.6786041293909,253.78074710398,25.4638640945166)) ;
#102542=CARTESIAN_POINT('Ctrl Pts',(45.6782777598473,253.794651469056,25.4775822300161)) ;
#102543=CARTESIAN_POINT('Ctrl Pts',(45.6779514776265,253.808552113907,25.4912966951182)) ;
#102544=CARTESIAN_POINT('Ctrl Pts',(45.6776998934371,253.824998688613,25.5021663724021)) ;
#102545=CARTESIAN_POINT('Ctrl Pts',(45.6775294165481,253.843066458683,25.5095788042595)) ;
#102546=CARTESIAN_POINT('Ctrl Pts',(45.6773589606669,253.861132002274,25.5169903226876)) ;
#102547=CARTESIAN_POINT('Ctrl Pts',(45.6772727272728,253.880472526098,25.5208035475559)) ;
#102548=CARTESIAN_POINT('Ctrl Pts',(45.6772727272728,253.9,25.5208035475559)) ;
#102549=CARTESIAN_POINT('',(42.9386363636364,253.9,25.5208035475559)) ;
#102550=CARTESIAN_POINT('Origin',(45.7,253.9,25.0213203435596)) ;
#102551=CARTESIAN_POINT('',(45.6809871063617,253.75,24.6718371395634)) ;
#102552=CARTESIAN_POINT('Origin',(45.7,253.75,25.0213203435596)) ;
#102553=CARTESIAN_POINT('',(45.6772727272728,253.9,24.5218371395634)) ;
#102554=CARTESIAN_POINT('Ctrl Pts',(45.6809871063617,253.75,24.6718371395631)) ;
#102555=CARTESIAN_POINT('Ctrl Pts',(45.6809474726104,253.75,24.6703790162594)) ;
#102556=CARTESIAN_POINT('Ctrl Pts',(45.6809079648117,253.750021261236,24.6689209669185)) ;
#102557=CARTESIAN_POINT('Ctrl Pts',(45.6808685931366,253.750063777237,24.667463456485)) ;
#102558=CARTESIAN_POINT('Ctrl Pts',(45.6803627963739,253.750609968276,24.6487392325951)) ;
#102559=CARTESIAN_POINT('Ctrl Pts',(45.679884582305,253.754658837467,24.6302810697321)) ;
#102560=CARTESIAN_POINT('Ctrl Pts',(45.6794511277464,253.762001431812,24.6130460247761)) ;
#102561=CARTESIAN_POINT('Ctrl Pts',(45.6789992518938,253.769656077527,24.5950785112738)) ;
#102562=CARTESIAN_POINT('Ctrl Pts',(45.6786041293905,253.78074710398,24.5787765926027)) ;
#102563=CARTESIAN_POINT('Ctrl Pts',(45.678277759847,253.794651469056,24.5650584571032)) ;
#102564=CARTESIAN_POINT('Ctrl Pts',(45.6779514776263,253.808552113907,24.5513439920011)) ;
#102565=CARTESIAN_POINT('Ctrl Pts',(45.6776998934372,253.824998688613,24.5404743147172)) ;
#102566=CARTESIAN_POINT('Ctrl Pts',(45.6775294165482,253.843066458683,24.5330618828599)) ;
#102567=CARTESIAN_POINT('Ctrl Pts',(45.6773589606669,253.861132002274,24.5256503644317)) ;
#102568=CARTESIAN_POINT('Ctrl Pts',(45.6772727272727,253.880472526098,24.5218371395634)) ;
#102569=CARTESIAN_POINT('Ctrl Pts',(45.6772727272727,253.9,24.5218371395634)) ;
#102570=CARTESIAN_POINT('Origin',(45.7,253.9,25.0213203435596)) ;
#102571=CARTESIAN_POINT('Origin',(42.5869707020053,253.9,24.6718371395634)) ;
#102572=CARTESIAN_POINT('',(45.1376473638895,253.75,24.6718371395634)) ;
#102573=CARTESIAN_POINT('',(42.5869707020053,253.75,24.6718371395634)) ;
#102574=CARTESIAN_POINT('',(45.2754819011524,253.9,24.5218371395634)) ;
#102575=CARTESIAN_POINT('Ctrl Pts',(45.1376473638895,253.75,24.6718371395634)) ;
#102576=CARTESIAN_POINT('Ctrl Pts',(45.1381850335709,253.75,24.6712600688988)) ;
#102577=CARTESIAN_POINT('Ctrl Pts',(45.1387226600695,253.750003330106,24.6706829503216)) ;
#102578=CARTESIAN_POINT('Ctrl Pts',(45.1531132725535,253.750181671152,24.655232733985)) ;
#102579=CARTESIAN_POINT('Ctrl Pts',(45.1669867461395,253.752566842488,24.6402737328004)) ;
#102580=CARTESIAN_POINT('Ctrl Pts',(45.1932346560154,253.761740190968,24.611858434734)) ;
#102581=CARTESIAN_POINT('Ctrl Pts',(45.2057640785244,253.768377217198,24.5982392280904)) ;
#102582=CARTESIAN_POINT('Ctrl Pts',(45.2303168022832,253.78721321578,24.5714615581854)) ;
#102583=CARTESIAN_POINT('Ctrl Pts',(45.2422449580739,253.800023548159,24.5583957973774)) ;
#102584=CARTESIAN_POINT('Ctrl Pts',(45.2595447243168,253.828041657271,24.5393982820176)) ;
#102585=CARTESIAN_POINT('Ctrl Pts',(45.2657214856064,253.841958224525,24.5325967432531)) ;
#102586=CARTESIAN_POINT('Ctrl Pts',(45.2735311811371,253.870954690135,24.5239903075244)) ;
#102587=CARTESIAN_POINT('Ctrl Pts',(45.2754819011524,253.885320776746,24.5218371395634)) ;
#102588=CARTESIAN_POINT('Ctrl Pts',(45.2754819011524,253.9,24.5218371395634)) ;
#102589=CARTESIAN_POINT('',(42.5869707020053,253.9,24.5218371395634)) ;
#102590=CARTESIAN_POINT('Origin',(40.2,253.9,25.0213203435596)) ;
#102591=CARTESIAN_POINT('',(45.0039779498781,253.75,23.8278816743835)) ;
#102592=CARTESIAN_POINT('Origin',(40.2,253.75,25.0213203435596)) ;
#102593=CARTESIAN_POINT('',(45.1814189338688,253.9,23.9279469374017)) ;
#102594=CARTESIAN_POINT('Ctrl Pts',(45.0039779498781,253.75,23.8278816743835)) ;
#102595=CARTESIAN_POINT('Ctrl Pts',(45.0046676287764,253.75,23.8282643521316)) ;
#102596=CARTESIAN_POINT('Ctrl Pts',(45.0053572814057,253.750003330105,23.8286470887883)) ;
#102597=CARTESIAN_POINT('Ctrl Pts',(45.0238179465996,253.750181671152,23.8388941738984)) ;
#102598=CARTESIAN_POINT('Ctrl Pts',(45.0416349896414,253.752566842488,23.8488338903424)) ;
#102599=CARTESIAN_POINT('Ctrl Pts',(45.0753790453708,253.761740190968,23.8677473945125)) ;
#102600=CARTESIAN_POINT('Ctrl Pts',(45.0915038005961,253.768377217198,23.8768282252525)) ;
#102601=CARTESIAN_POINT('Ctrl Pts',(45.12312958359,253.78721321578,23.8947080938071)) ;
#102602=CARTESIAN_POINT('Ctrl Pts',(45.1385114760162,253.800023548159,23.903448367913)) ;
#102603=CARTESIAN_POINT('Ctrl Pts',(45.1608350865289,253.828041657271,23.9161701569215)) ;
#102604=CARTESIAN_POINT('Ctrl Pts',(45.1688113266691,253.841958224525,23.9207300804757)) ;
#102605=CARTESIAN_POINT('Ctrl Pts',(45.1788983233951,253.870954690135,23.9265019586177)) ;
#102606=CARTESIAN_POINT('Ctrl Pts',(45.1814189338688,253.885320776746,23.9279469374017)) ;
#102607=CARTESIAN_POINT('Ctrl Pts',(45.1814189338688,253.9,23.9279469374017)) ;
#102608=CARTESIAN_POINT('Origin',(40.2,253.9,25.0213203435596)) ;
#102609=CARTESIAN_POINT('Origin',(42.9125942086827,253.9,24.5074134442792)) ;
#102610=CARTESIAN_POINT('',(45.5207247525188,253.75,23.6599804602402)) ;
#102611=CARTESIAN_POINT('',(42.9125942086827,253.75,24.5074134442792)) ;
#102612=CARTESIAN_POINT('',(45.5635447172382,253.9,23.8037867439466)) ;
#102613=CARTESIAN_POINT('Ctrl Pts',(45.5207247525188,253.75,23.6599804602402)) ;
#102614=CARTESIAN_POINT('Ctrl Pts',(45.5211376434623,253.75,23.661379465413)) ;
#102615=CARTESIAN_POINT('Ctrl Pts',(45.5215506313346,253.750021261236,23.662778361321)) ;
#102616=CARTESIAN_POINT('Ctrl Pts',(45.5219635821411,253.750063777237,23.6641767026334)) ;
#102617=CARTESIAN_POINT('Ctrl Pts',(45.5272686442365,253.750609968276,23.6821407975692)) ;
#102618=CARTESIAN_POINT('Ctrl Pts',(45.5325177216276,253.754658837467,23.6998433299153)) ;
#102619=CARTESIAN_POINT('Ctrl Pts',(45.5374314036355,253.762001431812,23.716368776554)) ;
#102620=CARTESIAN_POINT('Ctrl Pts',(45.5425539111805,253.769656077527,23.7335965346699)) ;
#102621=CARTESIAN_POINT('Ctrl Pts',(45.5472156972587,253.78074710398,23.7492226802186)) ;
#102622=CARTESIAN_POINT('Ctrl Pts',(45.551144438378,253.794651469056,23.7623702561121)) ;
#102623=CARTESIAN_POINT('Ctrl Pts',(45.555072128331,253.808552113907,23.7755143142662)) ;
#102624=CARTESIAN_POINT('Ctrl Pts',(45.5581917725533,253.824998688613,23.7859297354669)) ;
#102625=CARTESIAN_POINT('Ctrl Pts',(45.5603202068105,253.843066458683,23.7930320573423)) ;
#102626=CARTESIAN_POINT('Ctrl Pts',(45.5624483787821,253.861132002274,23.8001335040032)) ;
#102627=CARTESIAN_POINT('Ctrl Pts',(45.5635447172385,253.880472526098,23.8037867439465)) ;
#102628=CARTESIAN_POINT('Ctrl Pts',(45.5635447172382,253.9,23.8037867439466)) ;
#102629=CARTESIAN_POINT('',(42.9589467578389,253.9,24.6500719217234)) ;
#102630=CARTESIAN_POINT('Origin',(45.4308108396234,253.9,23.3217268744974)) ;
#102631=CARTESIAN_POINT('',(45.3047322539519,253.75,22.9952239032474)) ;
#102632=CARTESIAN_POINT('Origin',(45.4308108396234,253.75,23.3217268744974)) ;
#102633=CARTESIAN_POINT('',(45.2548471203588,253.9,22.8537132320653)) ;
#102634=CARTESIAN_POINT('Ctrl Pts',(45.3047322539504,253.75,22.9952239032429)) ;
#102635=CARTESIAN_POINT('Ctrl Pts',(45.3042439751329,253.75,22.9938493930776)) ;
#102636=CARTESIAN_POINT('Ctrl Pts',(45.303755838959,253.750021261236,22.9924749143332)) ;
#102637=CARTESIAN_POINT('Ctrl Pts',(45.3032679987774,253.750063777237,22.9911009060563)) ;
#102638=CARTESIAN_POINT('Ctrl Pts',(45.2970008540754,253.750609968276,22.9734494107125)) ;
#102639=CARTESIAN_POINT('Ctrl Pts',(45.290842159469,253.754658837467,22.9560424309124)) ;
#102640=CARTESIAN_POINT('Ctrl Pts',(45.2851039978953,253.762001431812,22.9397848739232)) ;
#102641=CARTESIAN_POINT('Ctrl Pts',(45.2791219714013,253.769656077527,22.9228363904432)) ;
#102642=CARTESIAN_POINT('Ctrl Pts',(45.2737086176589,253.78074710398,22.9074544440317)) ;
#102643=CARTESIAN_POINT('Ctrl Pts',(45.2691590847773,253.794651469056,22.8945085756089)) ;
#102644=CARTESIAN_POINT('Ctrl Pts',(45.2646107691597,253.808552113907,22.8815661709572)) ;
#102645=CARTESIAN_POINT('Ctrl Pts',(45.2610125833727,253.824998688613,22.8713062373364)) ;
#102646=CARTESIAN_POINT('Ctrl Pts',(45.2585598828031,253.843066458683,22.8643092759728)) ;
#102647=CARTESIAN_POINT('Ctrl Pts',(45.2561074844782,253.861132002274,22.85731317684)) ;
#102648=CARTESIAN_POINT('Ctrl Pts',(45.2548471203588,253.880472526098,22.8537132320654)) ;
#102649=CARTESIAN_POINT('Ctrl Pts',(45.254847120359,253.9,22.8537132320653)) ;
#102650=CARTESIAN_POINT('Origin',(45.4308108396234,253.9,23.3217268744974)) ;
#102651=CARTESIAN_POINT('Origin',(42.3621477910643,253.9,23.9513275530686)) ;
#102652=CARTESIAN_POINT('',(44.7879854513112,253.75,23.1631251173908)) ;
#102653=CARTESIAN_POINT('',(42.3621477910643,253.75,23.9513275530686)) ;
#102654=CARTESIAN_POINT('',(44.8727213369894,253.9,22.9778734255204)) ;
#102655=CARTESIAN_POINT('Ctrl Pts',(44.7879854513112,253.75,23.1631251173908)) ;
#102656=CARTESIAN_POINT('Ctrl Pts',(44.788318480923,253.75,23.162410141506)) ;
#102657=CARTESIAN_POINT('Ctrl Pts',(44.7886514546598,253.750003330106,23.1616951333976)) ;
#102658=CARTESIAN_POINT('Ctrl Pts',(44.7975633610212,253.750181671152,23.1425541606572)) ;
#102659=CARTESIAN_POINT('Ctrl Pts',(44.8061352328939,253.752566842488,23.1240401659929)) ;
#102660=CARTESIAN_POINT('Ctrl Pts',(44.8223176686178,253.761740190968,23.0889045613858)) ;
#102661=CARTESIAN_POINT('Ctrl Pts',(44.8300252912377,253.768377217198,23.0720801216756)) ;
#102662=CARTESIAN_POINT('Ctrl Pts',(44.845101564091,253.78721321578,23.0390258353215)) ;
#102663=CARTESIAN_POINT('Ctrl Pts',(44.8524083722489,253.800023548159,23.0229135555138)) ;
#102664=CARTESIAN_POINT('Ctrl Pts',(44.8629908725676,253.828041657271,22.9994999229698)) ;
#102665=CARTESIAN_POINT('Ctrl Pts',(44.8667635305755,253.841958224525,22.9911225509982)) ;
#102666=CARTESIAN_POINT('Ctrl Pts',(44.8715314574991,253.870954690135,22.9805240155764)) ;
#102667=CARTESIAN_POINT('Ctrl Pts',(44.8727213369894,253.885320776746,22.9778734255204)) ;
#102668=CARTESIAN_POINT('Ctrl Pts',(44.8727213369894,253.9,22.9778734255204)) ;
#102669=CARTESIAN_POINT('',(42.315795241908,253.9,23.8086690756243)) ;
#102670=CARTESIAN_POINT('Origin',(40.2,253.9,25.0213203435596)) ;
#102671=CARTESIAN_POINT('',(44.4000617028502,253.75,22.4017818933262)) ;
#102672=CARTESIAN_POINT('Origin',(40.2,253.75,25.0213203435596)) ;
#102673=CARTESIAN_POINT('',(44.5997399737516,253.9,22.4421173342227)) ;
#102674=CARTESIAN_POINT('Ctrl Pts',(44.4000617028502,253.75,22.4017818933262)) ;
#102675=CARTESIAN_POINT('Ctrl Pts',(44.400835880386,253.75,22.4019327189915)) ;
#102676=CARTESIAN_POINT('Ctrl Pts',(44.4016100511485,253.750003330106,22.4020836088011)) ;
#102677=CARTESIAN_POINT('Ctrl Pts',(44.4223337105147,253.750181671152,22.4061245065945)) ;
#102678=CARTESIAN_POINT('Ctrl Pts',(44.4423502667022,253.752566842488,22.4100719695998)) ;
#102679=CARTESIAN_POINT('Ctrl Pts',(44.4802873650014,253.761740190968,22.4176322943072)) ;
#102680=CARTESIAN_POINT('Ctrl Pts',(44.4984290495541,253.768377217198,22.4212858541613)) ;
#102681=CARTESIAN_POINT('Ctrl Pts',(44.5340321397943,253.78721321578,22.4285177152552)) ;
#102682=CARTESIAN_POINT('Ctrl Pts',(44.5513620820533,253.800023548159,22.4320769437325)) ;
#102683=CARTESIAN_POINT('Ctrl Pts',(44.5765243463011,253.828041657271,22.4372777090437)) ;
#102684=CARTESIAN_POINT('Ctrl Pts',(44.5855192953333,253.841958224525,22.4391496602992)) ;
#102685=CARTESIAN_POINT('Ctrl Pts',(44.5968962077347,253.870954690135,22.4415219892068)) ;
#102686=CARTESIAN_POINT('Ctrl Pts',(44.5997399737516,253.885320776746,22.4421173342227)) ;
#102687=CARTESIAN_POINT('Ctrl Pts',(44.5997399737516,253.9,22.4421173342227)) ;
#102688=CARTESIAN_POINT('Origin',(40.2,253.9,25.0213203435596)) ;
#102689=CARTESIAN_POINT('Origin',(42.621024432828,253.9,23.6943281289039)) ;
#102690=CARTESIAN_POINT('',(44.8396327882296,253.75,22.0824148057166)) ;
#102691=CARTESIAN_POINT('',(42.621024432828,253.75,23.6943281289039)) ;
#102692=CARTESIAN_POINT('',(44.9247955802669,253.9,22.2059506121228)) ;
#102693=CARTESIAN_POINT('Ctrl Pts',(44.8396327882296,253.75,22.0824148057166)) ;
#102694=CARTESIAN_POINT('Ctrl Pts',(44.8404577872253,253.75,22.0836177483836)) ;
#102695=CARTESIAN_POINT('Ctrl Pts',(44.8412828446445,253.750021261236,22.0848205571807)) ;
#102696=CARTESIAN_POINT('Ctrl Pts',(44.8421076954281,253.750063777237,22.086022849981)) ;
#102697=CARTESIAN_POINT('Ctrl Pts',(44.8527043199125,253.750609968276,22.101468365193)) ;
#102698=CARTESIAN_POINT('Ctrl Pts',(44.8631668725215,253.754658837467,22.11668241981)) ;
#102699=CARTESIAN_POINT('Ctrl Pts',(44.8729467056649,253.762001431812,22.1308806422755)) ;
#102700=CARTESIAN_POINT('Ctrl Pts',(44.8831421698776,253.769656077527,22.1456822720076)) ;
#102701=CARTESIAN_POINT('Ctrl Pts',(44.8924045364365,253.78074710398,22.1591030484338)) ;
#102702=CARTESIAN_POINT('Ctrl Pts',(44.9002038156649,253.794651469056,22.1703930883885)) ;
#102703=CARTESIAN_POINT('Ctrl Pts',(44.9080010081335,253.808552113907,22.1816801076023)) ;
#102704=CARTESIAN_POINT('Ctrl Pts',(44.9141865082534,253.824998688613,22.1906217387246)) ;
#102705=CARTESIAN_POINT('Ctrl Pts',(44.9184055076825,253.843066458683,22.1967187258681)) ;
#102706=CARTESIAN_POINT('Ctrl Pts',(44.9226239872069,253.861132002274,22.2028149616837)) ;
#102707=CARTESIAN_POINT('Ctrl Pts',(44.9247955802668,253.880472526098,22.2059506121229)) ;
#102708=CARTESIAN_POINT('Ctrl Pts',(44.9247955802668,253.9,22.2059506121229)) ;
#102709=CARTESIAN_POINT('',(42.7091922206719,253.9,23.8156806780601)) ;
#102710=CARTESIAN_POINT('Origin',(44.6495934690622,253.9,21.788501455951)) ;
#102711=CARTESIAN_POINT('',(44.4287906417638,253.75,21.5169391031533)) ;
#102712=CARTESIAN_POINT('Origin',(44.6495934690622,253.75,21.788501455951)) ;
#102713=CARTESIAN_POINT('',(44.3376178581133,253.9,21.3977698112471)) ;
#102714=CARTESIAN_POINT('Ctrl Pts',(44.4287906417615,253.75,21.5169391031502)) ;
#102715=CARTESIAN_POINT('Ctrl Pts',(44.4279015140102,253.75,21.5157827527532)) ;
#102716=CARTESIAN_POINT('Ctrl Pts',(44.4270125316307,253.750021261236,21.5146263881596)) ;
#102717=CARTESIAN_POINT('Ctrl Pts',(44.4261239761389,253.750063777237,21.5134703795409)) ;
#102718=CARTESIAN_POINT('Ctrl Pts',(44.4147089552932,253.750609968276,21.4986194640919)) ;
#102719=CARTESIAN_POINT('Ctrl Pts',(44.4034726360771,253.754658837467,21.4839675838201)) ;
#102720=CARTESIAN_POINT('Ctrl Pts',(44.3929914587243,253.762001431812,21.4702789177492)) ;
#102721=CARTESIAN_POINT('Ctrl Pts',(44.3820648440225,253.769656077527,21.4560084999418)) ;
#102722=CARTESIAN_POINT('Ctrl Pts',(44.3721631558231,253.78074710398,21.4430522178766)) ;
#102723=CARTESIAN_POINT('Ctrl Pts',(44.3638357995804,253.794651469056,21.4321458483308)) ;
#102724=CARTESIAN_POINT('Ctrl Pts',(44.3555106713887,253.808552113907,21.4212423968718)) ;
#102725=CARTESIAN_POINT('Ctrl Pts',(44.3489180994998,253.824998688613,21.4125965207017)) ;
#102726=CARTESIAN_POINT('Ctrl Pts',(44.3444232626702,253.843066458683,21.4066999411606)) ;
#102727=CARTESIAN_POINT('Ctrl Pts',(44.3399289797363,253.861132002274,21.4008040882512)) ;
#102728=CARTESIAN_POINT('Ctrl Pts',(44.3376178581132,253.880472526098,21.3977698112471)) ;
#102729=CARTESIAN_POINT('Ctrl Pts',(44.3376178581134,253.9,21.397769811247)) ;
#102730=CARTESIAN_POINT('Origin',(44.6495934690622,253.9,21.788501455951)) ;
#102731=CARTESIAN_POINT('Origin',(41.9256787897644,253.9,23.3355563159851)) ;
#102732=CARTESIAN_POINT('',(43.9892195563843,253.75,21.836306190763)) ;
#102733=CARTESIAN_POINT('',(41.9256787897644,253.75,23.3355563159851)) ;
#102734=CARTESIAN_POINT('',(44.012562251598,253.9,21.6339365333471)) ;
#102735=CARTESIAN_POINT('Ctrl Pts',(43.9892195563843,253.75,21.836306190763)) ;
#102736=CARTESIAN_POINT('Ctrl Pts',(43.9893153466677,253.75,21.8355232964791)) ;
#102737=CARTESIAN_POINT('Ctrl Pts',(43.9894110738533,253.750003330106,21.8347403888152)) ;
#102738=CARTESIAN_POINT('Ctrl Pts',(43.9919719146053,253.750181671152,21.8137823114442)) ;
#102739=CARTESIAN_POINT('Ctrl Pts',(43.9944031102216,253.752566842488,21.7935256020938)) ;
#102740=CARTESIAN_POINT('Ctrl Pts',(43.9989360222351,253.761740190968,21.7551090087292)) ;
#102741=CARTESIAN_POINT('Ctrl Pts',(44.0010673691616,253.768377217198,21.7367262293339)) ;
#102742=CARTESIAN_POINT('Ctrl Pts',(44.0051914204798,253.78721321578,21.7006309103819)) ;
#102743=CARTESIAN_POINT('Ctrl Pts',(44.007161639713,253.800023548159,21.683049293783)) ;
#102744=CARTESIAN_POINT('Ctrl Pts',(44.0099909852437,253.828041657271,21.6575114335403)) ;
#102745=CARTESIAN_POINT('Ctrl Pts',(44.0109902459184,253.841958224525,21.648378263899)) ;
#102746=CARTESIAN_POINT('Ctrl Pts',(44.0122496863275,253.870954690135,21.6368250872756)) ;
#102747=CARTESIAN_POINT('Ctrl Pts',(44.012562251598,253.885320776746,21.6339365333471)) ;
#102748=CARTESIAN_POINT('Ctrl Pts',(44.012562251598,253.9,21.633936533347)) ;
#102749=CARTESIAN_POINT('',(41.8375110019206,253.9,23.2142037668289)) ;
#102750=CARTESIAN_POINT('Origin',(40.2,253.9,25.0213203435596)) ;
#102751=CARTESIAN_POINT('',(43.3850141527966,253.75,21.2321007871753)) ;
#102752=CARTESIAN_POINT('Origin',(40.2,253.75,25.0213203435596)) ;
#102753=CARTESIAN_POINT('',(43.5873838102126,253.9,21.2087580919617)) ;
#102754=CARTESIAN_POINT('Ctrl Pts',(43.3850141527966,253.75,21.2321007871753)) ;
#102755=CARTESIAN_POINT('Ctrl Pts',(43.3857970470791,253.75,21.2320049968921)) ;
#102756=CARTESIAN_POINT('Ctrl Pts',(43.3865799547417,253.750003330105,21.2319092697067)) ;
#102757=CARTESIAN_POINT('Ctrl Pts',(43.4075380321123,253.750181671152,21.2293484289549)) ;
#102758=CARTESIAN_POINT('Ctrl Pts',(43.4277947414631,253.752566842487,21.2269172333384)) ;
#102759=CARTESIAN_POINT('Ctrl Pts',(43.4662113348294,253.761740190968,21.2223843213247)) ;
#102760=CARTESIAN_POINT('Ctrl Pts',(43.4845941142251,253.768377217197,21.2202529743981)) ;
#102761=CARTESIAN_POINT('Ctrl Pts',(43.5206894331778,253.78721321578,21.2161289230798)) ;
#102762=CARTESIAN_POINT('Ctrl Pts',(43.5382710497766,253.800023548159,21.2141587038466)) ;
#102763=CARTESIAN_POINT('Ctrl Pts',(43.5638089100192,253.828041657271,21.211329358316)) ;
#102764=CARTESIAN_POINT('Ctrl Pts',(43.5729420796606,253.841958224525,21.2103300976412)) ;
#102765=CARTESIAN_POINT('Ctrl Pts',(43.5844952562841,253.870954690135,21.2090706572321)) ;
#102766=CARTESIAN_POINT('Ctrl Pts',(43.5873838102126,253.885320776746,21.2087580919617)) ;
#102767=CARTESIAN_POINT('Ctrl Pts',(43.5873838102126,253.9,21.2087580919617)) ;
#102768=CARTESIAN_POINT('Origin',(40.2,253.9,25.0213203435596)) ;
#102769=CARTESIAN_POINT('Origin',(42.0924679172189,253.9,23.0111380571975)) ;
#102770=CARTESIAN_POINT('',(43.7043812404062,253.75,20.792529701796)) ;
#102771=CARTESIAN_POINT('',(42.0924679172189,253.75,23.0111380571975)) ;
#102772=CARTESIAN_POINT('',(43.8235505323125,253.9,20.8837024854464)) ;
#102773=CARTESIAN_POINT('Ctrl Pts',(43.7043812404062,253.75,20.792529701796)) ;
#102774=CARTESIAN_POINT('Ctrl Pts',(43.7055375908043,253.75,20.7934188295481)) ;
#102775=CARTESIAN_POINT('Ctrl Pts',(43.7066939553987,253.750021261236,20.7943078119284)) ;
#102776=CARTESIAN_POINT('Ctrl Pts',(43.7078499640185,253.750063777237,20.7951963674209)) ;
#102777=CARTESIAN_POINT('Ctrl Pts',(43.7227008794692,253.750609968276,20.8066113882653)) ;
#102778=CARTESIAN_POINT('Ctrl Pts',(43.7373527597391,253.754658837467,20.8178477074831)) ;
#102779=CARTESIAN_POINT('Ctrl Pts',(43.7510414258101,253.762001431812,20.8283288848357)) ;
#102780=CARTESIAN_POINT('Ctrl Pts',(43.7653118436178,253.769656077527,20.8392554995374)) ;
#102781=CARTESIAN_POINT('Ctrl Pts',(43.778268125683,253.78074710398,20.8491571877367)) ;
#102782=CARTESIAN_POINT('Ctrl Pts',(43.7891744952286,253.794651469056,20.8574845439794)) ;
#102783=CARTESIAN_POINT('Ctrl Pts',(43.8000779466876,253.808552113907,20.8658096721711)) ;
#102784=CARTESIAN_POINT('Ctrl Pts',(43.8087238228576,253.824998688613,20.8724022440603)) ;
#102785=CARTESIAN_POINT('Ctrl Pts',(43.8146204023986,253.843066458683,20.87689708089)) ;
#102786=CARTESIAN_POINT('Ctrl Pts',(43.820516255308,253.861132002274,20.8813913638238)) ;
#102787=CARTESIAN_POINT('Ctrl Pts',(43.8235505323122,253.880472526098,20.8837024854468)) ;
#102788=CARTESIAN_POINT('Ctrl Pts',(43.8235505323123,253.9,20.8837024854466)) ;
#102789=CARTESIAN_POINT('',(42.2138204663752,253.9,23.0993058450414)) ;
#102790=CARTESIAN_POINT('Origin',(43.4328188876086,253.9,20.5717268744974)) ;
#102791=CARTESIAN_POINT('',(43.1389055378431,253.75,20.38168755533)) ;
#102792=CARTESIAN_POINT('Origin',(43.4328188876086,253.75,20.5717268744974)) ;
#102793=CARTESIAN_POINT('',(43.0153697314369,253.9,20.2965247632928)) ;
#102794=CARTESIAN_POINT('Ctrl Pts',(43.1389055378404,253.75,20.381687555328)) ;
#102795=CARTESIAN_POINT('Ctrl Pts',(43.137702595174,253.75,20.3808625563329)) ;
#102796=CARTESIAN_POINT('Ctrl Pts',(43.1364997863777,253.750021261236,20.3800374989153)) ;
#102797=CARTESIAN_POINT('Ctrl Pts',(43.1352974935784,253.750063777237,20.3792126481319)) ;
#102798=CARTESIAN_POINT('Ctrl Pts',(43.1198519783686,253.750609968276,20.3686160236418)) ;
#102799=CARTESIAN_POINT('Ctrl Pts',(43.1046379237494,253.754658837467,20.3581534710382)) ;
#102800=CARTESIAN_POINT('Ctrl Pts',(43.0904397012842,253.762001431812,20.3483736378948)) ;
#102801=CARTESIAN_POINT('Ctrl Pts',(43.075638071552,253.769656077527,20.3381781736819)) ;
#102802=CARTESIAN_POINT('Ctrl Pts',(43.0622172951261,253.78074710398,20.3289158071227)) ;
#102803=CARTESIAN_POINT('Ctrl Pts',(43.0509272551714,253.794651469056,20.3211165278944)) ;
#102804=CARTESIAN_POINT('Ctrl Pts',(43.0396402359575,253.808552113907,20.3133193354259)) ;
#102805=CARTESIAN_POINT('Ctrl Pts',(43.0306986048352,253.824998688613,20.3071338353061)) ;
#102806=CARTESIAN_POINT('Ctrl Pts',(43.0246016176917,253.843066458683,20.3029148358772)) ;
#102807=CARTESIAN_POINT('Ctrl Pts',(43.0185053818759,253.861132002274,20.2986963563528)) ;
#102808=CARTESIAN_POINT('Ctrl Pts',(43.0153697314369,253.880472526098,20.2965247632927)) ;
#102809=CARTESIAN_POINT('Ctrl Pts',(43.0153697314369,253.9,20.2965247632927)) ;
#102810=CARTESIAN_POINT('Origin',(43.4328188876086,253.9,20.5717268744974)) ;
#102811=CARTESIAN_POINT('Origin',(41.3202883250113,253.9,22.8847994073294)) ;
#102812=CARTESIAN_POINT('',(42.8195384502335,253.75,20.8212586407095)) ;
#102813=CARTESIAN_POINT('',(41.3202883250113,253.75,22.8847994073294)) ;
#102814=CARTESIAN_POINT('',(42.7792030093369,253.9,20.6215803698081)) ;
#102815=CARTESIAN_POINT('Ctrl Pts',(42.8195384502335,253.75,20.8212586407095)) ;
#102816=CARTESIAN_POINT('Ctrl Pts',(42.8193876245682,253.75,20.8204844631737)) ;
#102817=CARTESIAN_POINT('Ctrl Pts',(42.8192367347586,253.750003330106,20.8197102924112)) ;
#102818=CARTESIAN_POINT('Ctrl Pts',(42.8151958369649,253.750181671152,20.7989866330446)) ;
#102819=CARTESIAN_POINT('Ctrl Pts',(42.8112483739597,253.752566842488,20.7789700768574)) ;
#102820=CARTESIAN_POINT('Ctrl Pts',(42.8036880492523,253.761740190968,20.7410329785579)) ;
#102821=CARTESIAN_POINT('Ctrl Pts',(42.8000344893984,253.768377217198,20.7228912940054)) ;
#102822=CARTESIAN_POINT('Ctrl Pts',(42.7928026283045,253.78721321578,20.6872882037656)) ;
#102823=CARTESIAN_POINT('Ctrl Pts',(42.7892433998272,253.800023548159,20.6699582615064)) ;
#102824=CARTESIAN_POINT('Ctrl Pts',(42.7840426345159,253.828041657271,20.6447959972585)) ;
#102825=CARTESIAN_POINT('Ctrl Pts',(42.7821706832604,253.841958224525,20.6358010482263)) ;
#102826=CARTESIAN_POINT('Ctrl Pts',(42.7797983543528,253.870954690135,20.6244241358249)) ;
#102827=CARTESIAN_POINT('Ctrl Pts',(42.7792030093369,253.885320776746,20.6215803698081)) ;
#102828=CARTESIAN_POINT('Ctrl Pts',(42.7792030093369,253.9,20.6215803698081)) ;
#102829=CARTESIAN_POINT('',(41.1989357758551,253.9,22.7966316194855)) ;
#102830=CARTESIAN_POINT('Origin',(40.2,253.9,25.0213203435596)) ;
#102831=CARTESIAN_POINT('',(42.0581952261689,253.75,20.4333348922484)) ;
#102832=CARTESIAN_POINT('Origin',(40.2,253.75,25.0213203435596)) ;
#102833=CARTESIAN_POINT('',(42.2434469180392,253.9,20.3485990065702)) ;
#102834=CARTESIAN_POINT('Ctrl Pts',(42.0581952261685,253.75,20.4333348922483)) ;
#102835=CARTESIAN_POINT('Ctrl Pts',(42.0589102020531,253.75,20.4330018626366)) ;
#102836=CARTESIAN_POINT('Ctrl Pts',(42.0596252101622,253.750003330106,20.4326688888998)) ;
#102837=CARTESIAN_POINT('Ctrl Pts',(42.0787661829037,253.750181671152,20.4237569825383)) ;
#102838=CARTESIAN_POINT('Ctrl Pts',(42.0972801775669,253.752566842488,20.4151851106656)) ;
#102839=CARTESIAN_POINT('Ctrl Pts',(42.132415782174,253.761740190968,20.3990026749418)) ;
#102840=CARTESIAN_POINT('Ctrl Pts',(42.1492402218842,253.768377217198,20.3912950523219)) ;
#102841=CARTESIAN_POINT('Ctrl Pts',(42.1822945082381,253.78721321578,20.3762187794687)) ;
#102842=CARTESIAN_POINT('Ctrl Pts',(42.1984067880458,253.800023548159,20.3689119713107)) ;
#102843=CARTESIAN_POINT('Ctrl Pts',(42.2218204205899,253.828041657271,20.3583294709921)) ;
#102844=CARTESIAN_POINT('Ctrl Pts',(42.2301977925614,253.841958224525,20.3545568129842)) ;
#102845=CARTESIAN_POINT('Ctrl Pts',(42.2407963279832,253.870954690135,20.3497888860605)) ;
#102846=CARTESIAN_POINT('Ctrl Pts',(42.2434469180392,253.885320776746,20.3485990065702)) ;
#102847=CARTESIAN_POINT('Ctrl Pts',(42.2434469180392,253.9,20.3485990065702)) ;
#102848=CARTESIAN_POINT('Origin',(40.2,253.9,25.0213203435596)) ;
#102849=CARTESIAN_POINT('Origin',(41.3786634562732,253.9,22.5247186334439)) ;
#102850=CARTESIAN_POINT('',(42.3676071114944,253.9,19.9664732232009)) ;
#102851=CARTESIAN_POINT('',(41.5213219337175,253.9,22.5710711826001)) ;
#102852=CARTESIAN_POINT('',(42.2260964403123,253.75,19.9165880896075)) ;
#102853=CARTESIAN_POINT('',(41.3786634562732,253.75,22.5247186334439)) ;
#102854=CARTESIAN_POINT('Ctrl Pts',(42.2260964403123,253.75,19.9165880896075)) ;
#102855=CARTESIAN_POINT('Ctrl Pts',(42.2274709504793,253.75,19.9170763684256)) ;
#102856=CARTESIAN_POINT('Ctrl Pts',(42.2288454292246,253.750021261236,19.9175645046006)) ;
#102857=CARTESIAN_POINT('Ctrl Pts',(42.2302194375034,253.750063777237,19.9180523447822)) ;
#102858=CARTESIAN_POINT('Ctrl Pts',(42.2478709328509,253.750609968276,19.9243194894782)) ;
#102859=CARTESIAN_POINT('Ctrl Pts',(42.2652779126467,253.754658837467,19.9304781840933)) ;
#102860=CARTESIAN_POINT('Ctrl Pts',(42.2815354696358,253.762001431812,19.9362163456661)) ;
#102861=CARTESIAN_POINT('Ctrl Pts',(42.298483953116,253.769656077527,19.9421983721592)) ;
#102862=CARTESIAN_POINT('Ctrl Pts',(42.3138658995279,253.78074710398,19.947611725901)) ;
#102863=CARTESIAN_POINT('Ctrl Pts',(42.3268117679507,253.794651469056,19.9521612587826)) ;
#102864=CARTESIAN_POINT('Ctrl Pts',(42.3397541726024,253.808552113907,19.9567095744001)) ;
#102865=CARTESIAN_POINT('Ctrl Pts',(42.3500141062233,253.824998688613,19.9603077601869)) ;
#102866=CARTESIAN_POINT('Ctrl Pts',(42.3570110675869,253.843066458683,19.9627604607566)) ;
#102867=CARTESIAN_POINT('Ctrl Pts',(42.3640071667196,253.861132002274,19.9652128590817)) ;
#102868=CARTESIAN_POINT('Ctrl Pts',(42.3676071114944,253.880472526098,19.9664732232006)) ;
#102869=CARTESIAN_POINT('Ctrl Pts',(42.3676071114945,253.9,19.9664732232005)) ;
#102870=CARTESIAN_POINT('Origin',(41.8995934690622,253.9,19.7905095039363)) ;
#102871=CARTESIAN_POINT('',(41.4175335996131,253.9,19.6577756263215)) ;
#102872=CARTESIAN_POINT('Origin',(41.8995934690622,253.9,19.7905095039363)) ;
#102873=CARTESIAN_POINT('',(41.5613398833193,253.75,19.7005955910415)) ;
#102874=CARTESIAN_POINT('Origin',(41.8995934690622,253.75,19.7905095039363)) ;
#102875=CARTESIAN_POINT('Ctrl Pts',(41.5613398833094,253.75,19.7005955910383)) ;
#102876=CARTESIAN_POINT('Ctrl Pts',(41.5599408781403,253.75,19.7001827000958)) ;
#102877=CARTESIAN_POINT('Ctrl Pts',(41.5585419822356,253.750021261236,19.699769712222)) ;
#102878=CARTESIAN_POINT('Ctrl Pts',(41.5571436409267,253.750063777237,19.6993567614174)) ;
#102879=CARTESIAN_POINT('Ctrl Pts',(41.5391795459882,253.750609968276,19.694051699333)) ;
#102880=CARTESIAN_POINT('Ctrl Pts',(41.521477013645,253.754658837467,19.6888026219303)) ;
#102881=CARTESIAN_POINT('Ctrl Pts',(41.5049515670061,253.762001431812,19.683888939923)) ;
#102882=CARTESIAN_POINT('Ctrl Pts',(41.4877238088899,253.769656077527,19.6787664323788)) ;
#102883=CARTESIAN_POINT('Ctrl Pts',(41.4720976633411,253.78074710398,19.6741046463012)) ;
#102884=CARTESIAN_POINT('Ctrl Pts',(41.4589500874475,253.794651469056,19.6701759051819)) ;
#102885=CARTESIAN_POINT('Ctrl Pts',(41.4458060292935,253.808552113907,19.6662482152289)) ;
#102886=CARTESIAN_POINT('Ctrl Pts',(41.4353906080927,253.824998688613,19.6631285710069)) ;
#102887=CARTESIAN_POINT('Ctrl Pts',(41.4282882862173,253.843066458683,19.6610001367495)) ;
#102888=CARTESIAN_POINT('Ctrl Pts',(41.4211868395564,253.861132002274,19.6588719647777)) ;
#102889=CARTESIAN_POINT('Ctrl Pts',(41.4175335996131,253.880472526098,19.6577756263216)) ;
#102890=CARTESIAN_POINT('Ctrl Pts',(41.4175335996131,253.9,19.6577756263216)) ;
#102891=CARTESIAN_POINT('Origin',(40.6052362334984,253.9,22.6431800539285)) ;
#102892=CARTESIAN_POINT('',(41.2933734061579,253.9,20.0399014096908)) ;
#102893=CARTESIAN_POINT('',(40.4625777560541,253.9,22.5968275047722)) ;
#102894=CARTESIAN_POINT('',(41.3934386691762,253.75,20.2173423936815)) ;
#102895=CARTESIAN_POINT('',(40.6052362334984,253.75,22.6431800539285)) ;
#102896=CARTESIAN_POINT('Ctrl Pts',(41.3934386691762,253.75,20.2173423936815)) ;
#102897=CARTESIAN_POINT('Ctrl Pts',(41.3930559914292,253.75,20.2166527147851)) ;
#102898=CARTESIAN_POINT('Ctrl Pts',(41.3926732547703,253.750003330106,20.2159630621521)) ;
#102899=CARTESIAN_POINT('Ctrl Pts',(41.3824261696622,253.750181671152,20.197502396961)) ;
#102900=CARTESIAN_POINT('Ctrl Pts',(41.3724864532176,253.752566842488,20.1796853539185)) ;
#102901=CARTESIAN_POINT('Ctrl Pts',(41.3535729490475,253.761740190968,20.1459412981892)) ;
#102902=CARTESIAN_POINT('Ctrl Pts',(41.3444921183073,253.768377217198,20.1298165429637)) ;
#102903=CARTESIAN_POINT('Ctrl Pts',(41.3266122497526,253.78721321578,20.0981907599697)) ;
#102904=CARTESIAN_POINT('Ctrl Pts',(41.3178719756466,253.800023548159,20.0828088675435)) ;
#102905=CARTESIAN_POINT('Ctrl Pts',(41.3051501866381,253.828041657271,20.0604852570307)) ;
#102906=CARTESIAN_POINT('Ctrl Pts',(41.3005902630839,253.841958224525,20.0525090168905)) ;
#102907=CARTESIAN_POINT('Ctrl Pts',(41.294818384942,253.870954690135,20.0424220201646)) ;
#102908=CARTESIAN_POINT('Ctrl Pts',(41.2933734061579,253.885320776746,20.0399014096908)) ;
#102909=CARTESIAN_POINT('Ctrl Pts',(41.2933734061579,253.9,20.0399014096908)) ;
#102910=CARTESIAN_POINT('Origin',(40.2,253.9,25.0213203435596)) ;
#102911=CARTESIAN_POINT('',(40.6994832039963,253.9,19.9458384424072)) ;
#102912=CARTESIAN_POINT('Origin',(40.2,253.9,25.0213203435596)) ;
#102913=CARTESIAN_POINT('',(40.5494832039963,253.75,20.0836729796702)) ;
#102914=CARTESIAN_POINT('Origin',(40.2,253.75,25.0213203435596)) ;
#102915=CARTESIAN_POINT('Ctrl Pts',(40.5494832039963,253.75,20.0836729796702)) ;
#102916=CARTESIAN_POINT('Ctrl Pts',(40.5500602746619,253.75,20.0831353099878)) ;
#102917=CARTESIAN_POINT('Ctrl Pts',(40.5506373932401,253.750003330106,20.0825976834882)) ;
#102918=CARTESIAN_POINT('Ctrl Pts',(40.5660876095772,253.750181671152,20.0682070710039)) ;
#102919=CARTESIAN_POINT('Ctrl Pts',(40.5810466107612,253.752566842488,20.0543335974184)) ;
#102920=CARTESIAN_POINT('Ctrl Pts',(40.6094619088267,253.761740190969,20.0280856875433)) ;
#102921=CARTESIAN_POINT('Ctrl Pts',(40.6230811154698,253.768377217198,20.0155562650348)) ;
#102922=CARTESIAN_POINT('Ctrl Pts',(40.6498587853742,253.78721321578,19.9910035412764)) ;
#102923=CARTESIAN_POINT('Ctrl Pts',(40.6629245461823,253.800023548159,19.9790753854858)) ;
#102924=CARTESIAN_POINT('Ctrl Pts',(40.681922061542,253.828041657271,19.9617756192428)) ;
#102925=CARTESIAN_POINT('Ctrl Pts',(40.6887236003065,253.841958224525,19.9555988579533)) ;
#102926=CARTESIAN_POINT('Ctrl Pts',(40.6973300360353,253.870954690135,19.9477891624225)) ;
#102927=CARTESIAN_POINT('Ctrl Pts',(40.6994832039963,253.885320776746,19.9458384424072)) ;
#102928=CARTESIAN_POINT('Ctrl Pts',(40.6994832039963,253.9,19.9458384424072)) ;
#102929=CARTESIAN_POINT('Origin',(40.5494832039963,253.9,22.2826839799233)) ;
#102930=CARTESIAN_POINT('',(40.6994832039963,253.9,19.5440476162869)) ;
#102931=CARTESIAN_POINT('',(40.6994832039963,253.9,22.2826839799233)) ;
#102932=CARTESIAN_POINT('',(40.5494832039963,253.75,19.5403332371978)) ;
#102933=CARTESIAN_POINT('',(40.5494832039963,253.75,22.2826839799233)) ;
#102934=CARTESIAN_POINT('Ctrl Pts',(40.5494832039963,253.75,19.5403332371978)) ;
#102935=CARTESIAN_POINT('Ctrl Pts',(40.5509413273001,253.75,19.5403728709491)) ;
#102936=CARTESIAN_POINT('Ctrl Pts',(40.5523993766411,253.750021261236,19.5404123787478)) ;
#102937=CARTESIAN_POINT('Ctrl Pts',(40.5538568870747,253.750063777237,19.5404517504229)) ;
#102938=CARTESIAN_POINT('Ctrl Pts',(40.5725811109644,253.750609968276,19.5409575471863)) ;
#102939=CARTESIAN_POINT('Ctrl Pts',(40.5910392738275,253.754658837467,19.5414357612545)) ;
#102940=CARTESIAN_POINT('Ctrl Pts',(40.6082743187835,253.762001431812,19.5418692158132)) ;
#102941=CARTESIAN_POINT('Ctrl Pts',(40.626241832286,253.769656077527,19.5423210916659)) ;
#102942=CARTESIAN_POINT('Ctrl Pts',(40.642543750957,253.78074710398,19.5427162141691)) ;
#102943=CARTESIAN_POINT('Ctrl Pts',(40.6562618864565,253.794651469056,19.5430425837128)) ;
#102944=CARTESIAN_POINT('Ctrl Pts',(40.6699763515586,253.808552113907,19.5433688659336)) ;
#102945=CARTESIAN_POINT('Ctrl Pts',(40.6808460288425,253.824998688613,19.5436204501224)) ;
#102946=CARTESIAN_POINT('Ctrl Pts',(40.6882584606999,253.843066458683,19.5437909270114)) ;
#102947=CARTESIAN_POINT('Ctrl Pts',(40.695669979128,253.861132002274,19.5439613828926)) ;
#102948=CARTESIAN_POINT('Ctrl Pts',(40.6994832039963,253.880472526098,19.5440476162869)) ;
#102949=CARTESIAN_POINT('Ctrl Pts',(40.6994832039963,253.9,19.5440476162869)) ;
#102950=CARTESIAN_POINT('Origin',(40.2,253.9,19.5213203435596)) ;
#102951=CARTESIAN_POINT('',(39.7005167960037,253.9,19.5440476162869)) ;
#102952=CARTESIAN_POINT('Origin',(40.2,253.9,19.5213203435596)) ;
#102953=CARTESIAN_POINT('',(39.8505167960037,253.75,19.5403332371979)) ;
#102954=CARTESIAN_POINT('Origin',(40.2,253.75,19.5213203435596)) ;
#102955=CARTESIAN_POINT('Ctrl Pts',(39.8505167960037,253.75,19.5403332371979)) ;
#102956=CARTESIAN_POINT('Ctrl Pts',(39.8490586726999,253.75,19.5403728709491)) ;
#102957=CARTESIAN_POINT('Ctrl Pts',(39.8476006233589,253.750021261236,19.5404123787479)) ;
#102958=CARTESIAN_POINT('Ctrl Pts',(39.8461431129253,253.750063777237,19.540451750423)) ;
#102959=CARTESIAN_POINT('Ctrl Pts',(39.8274188890355,253.750609968276,19.5409575471857)) ;
#102960=CARTESIAN_POINT('Ctrl Pts',(39.8089607261725,253.754658837467,19.5414357612546)) ;
#102961=CARTESIAN_POINT('Ctrl Pts',(39.7917256812165,253.762001431812,19.5418692158132)) ;
#102962=CARTESIAN_POINT('Ctrl Pts',(39.773758167714,253.769656077527,19.5423210916658)) ;
#102963=CARTESIAN_POINT('Ctrl Pts',(39.757456249043,253.78074710398,19.5427162141691)) ;
#102964=CARTESIAN_POINT('Ctrl Pts',(39.7437381135436,253.794651469056,19.5430425837128)) ;
#102965=CARTESIAN_POINT('Ctrl Pts',(39.7300236484415,253.808552113907,19.5433688659337)) ;
#102966=CARTESIAN_POINT('Ctrl Pts',(39.7191539711575,253.824998688613,19.5436204501225)) ;
#102967=CARTESIAN_POINT('Ctrl Pts',(39.7117415393002,253.843066458683,19.5437909270115)) ;
#102968=CARTESIAN_POINT('Ctrl Pts',(39.704330020872,253.861132002274,19.5439613828928)) ;
#102969=CARTESIAN_POINT('Ctrl Pts',(39.7005167960037,253.880472526098,19.5440476162869)) ;
#102970=CARTESIAN_POINT('Ctrl Pts',(39.7005167960037,253.9,19.5440476162869)) ;
#102971=CARTESIAN_POINT('Origin',(39.8505167960037,253.9,22.6343496415544)) ;
#102972=CARTESIAN_POINT('',(39.7005167960037,253.9,19.9458384424072)) ;
#102973=CARTESIAN_POINT('',(39.7005167960037,253.9,22.6343496415544)) ;
#102974=CARTESIAN_POINT('',(39.8505167960037,253.75,20.0836729796702)) ;
#102975=CARTESIAN_POINT('',(39.8505167960037,253.75,22.6343496415544)) ;
#102976=CARTESIAN_POINT('Ctrl Pts',(39.8505167960037,253.75,20.0836729796702)) ;
#102977=CARTESIAN_POINT('Ctrl Pts',(39.8499397253381,253.75,20.0831353099878)) ;
#102978=CARTESIAN_POINT('Ctrl Pts',(39.8493626067599,253.750003330106,20.0825976834882)) ;
#102979=CARTESIAN_POINT('Ctrl Pts',(39.833912390423,253.750181671152,20.0682070710039)) ;
#102980=CARTESIAN_POINT('Ctrl Pts',(39.8189533892388,253.752566842488,20.0543335974184)) ;
#102981=CARTESIAN_POINT('Ctrl Pts',(39.7905380911733,253.761740190969,20.0280856875433)) ;
#102982=CARTESIAN_POINT('Ctrl Pts',(39.7769188845303,253.768377217198,20.0155562650348)) ;
#102983=CARTESIAN_POINT('Ctrl Pts',(39.7501412146258,253.78721321578,19.9910035412764)) ;
#102984=CARTESIAN_POINT('Ctrl Pts',(39.7370754538178,253.800023548159,19.9790753854858)) ;
#102985=CARTESIAN_POINT('Ctrl Pts',(39.718077938458,253.828041657271,19.9617756192428)) ;
#102986=CARTESIAN_POINT('Ctrl Pts',(39.7112763996935,253.841958224525,19.9555988579533)) ;
#102987=CARTESIAN_POINT('Ctrl Pts',(39.7026699639648,253.870954690135,19.9477891624225)) ;
#102988=CARTESIAN_POINT('Ctrl Pts',(39.7005167960037,253.885320776746,19.9458384424072)) ;
#102989=CARTESIAN_POINT('Ctrl Pts',(39.7005167960037,253.9,19.9458384424072)) ;
#102990=CARTESIAN_POINT('Origin',(40.2,253.9,25.0213203435596)) ;
#102991=CARTESIAN_POINT('',(39.1066265938421,253.9,20.0399014096908)) ;
#102992=CARTESIAN_POINT('Origin',(40.2,253.9,25.0213203435596)) ;
#102993=CARTESIAN_POINT('',(39.0065613308239,253.75,20.2173423936815)) ;
#102994=CARTESIAN_POINT('Origin',(40.2,253.75,25.0213203435596)) ;
#102995=CARTESIAN_POINT('Ctrl Pts',(39.0065613308239,253.75,20.2173423936815)) ;
#102996=CARTESIAN_POINT('Ctrl Pts',(39.0069440085716,253.75,20.2166527147839)) ;
#102997=CARTESIAN_POINT('Ctrl Pts',(39.0073267452311,253.750003330106,20.2159630621497)) ;
#102998=CARTESIAN_POINT('Ctrl Pts',(39.0175738303395,253.750181671152,20.197502396958)) ;
#102999=CARTESIAN_POINT('Ctrl Pts',(39.0275135467838,253.752566842488,20.1796853539161)) ;
#103000=CARTESIAN_POINT('Ctrl Pts',(39.0464270509533,253.761740190969,20.1459412981879)) ;
#103001=CARTESIAN_POINT('Ctrl Pts',(39.0555078816931,253.768377217198,20.1298165429631)) ;
#103002=CARTESIAN_POINT('Ctrl Pts',(39.0733877502474,253.78721321578,20.0981907599697)) ;
#103003=CARTESIAN_POINT('Ctrl Pts',(39.0821280243534,253.800023548159,20.0828088675435)) ;
#103004=CARTESIAN_POINT('Ctrl Pts',(39.0948498133619,253.828041657271,20.0604852570307)) ;
#103005=CARTESIAN_POINT('Ctrl Pts',(39.0994097369161,253.841958224525,20.0525090168905)) ;
#103006=CARTESIAN_POINT('Ctrl Pts',(39.1051816150581,253.870954690135,20.0424220201645)) ;
#103007=CARTESIAN_POINT('Ctrl Pts',(39.1066265938421,253.885320776746,20.0399014096908)) ;
#103008=CARTESIAN_POINT('Ctrl Pts',(39.1066265938421,253.9,20.0399014096908)) ;
#103009=CARTESIAN_POINT('Origin',(39.6860931007195,253.9,22.3087261348769)) ;
#103010=CARTESIAN_POINT('',(38.982466400387,253.9,19.6577756263215)) ;
#103011=CARTESIAN_POINT('',(39.8287515781638,253.9,22.2623735857207)) ;
#103012=CARTESIAN_POINT('',(38.8386601166806,253.75,19.7005955910409)) ;
#103013=CARTESIAN_POINT('',(39.6860931007195,253.75,22.3087261348769)) ;
#103014=CARTESIAN_POINT('Ctrl Pts',(38.8386601166806,253.75,19.7005955910409)) ;
#103015=CARTESIAN_POINT('Ctrl Pts',(38.840059121853,253.75,19.7001827000975)) ;
#103016=CARTESIAN_POINT('Ctrl Pts',(38.841458017761,253.750021261236,19.6997697122226)) ;
#103017=CARTESIAN_POINT('Ctrl Pts',(38.8428563590732,253.750063777237,19.6993567614171)) ;
#103018=CARTESIAN_POINT('Ctrl Pts',(38.8608204540116,253.750609968276,19.6940516993336)) ;
#103019=CARTESIAN_POINT('Ctrl Pts',(38.8785229863551,253.754658837467,19.6888026219308)) ;
#103020=CARTESIAN_POINT('Ctrl Pts',(38.8950484329941,253.762001431812,19.6838889399233)) ;
#103021=CARTESIAN_POINT('Ctrl Pts',(38.9122761911102,253.769656077527,19.6787664323789)) ;
#103022=CARTESIAN_POINT('Ctrl Pts',(38.9279023366589,253.78074710398,19.6741046463011)) ;
#103023=CARTESIAN_POINT('Ctrl Pts',(38.9410499125525,253.794651469056,19.6701759051817)) ;
#103024=CARTESIAN_POINT('Ctrl Pts',(38.9541939707065,253.808552113907,19.6662482152286)) ;
#103025=CARTESIAN_POINT('Ctrl Pts',(38.9646093919074,253.824998688613,19.6631285710068)) ;
#103026=CARTESIAN_POINT('Ctrl Pts',(38.9717117137827,253.843066458683,19.6610001367494)) ;
#103027=CARTESIAN_POINT('Ctrl Pts',(38.9788131604436,253.861132002274,19.6588719647776)) ;
#103028=CARTESIAN_POINT('Ctrl Pts',(38.9824664003869,253.880472526098,19.6577756263214)) ;
#103029=CARTESIAN_POINT('Ctrl Pts',(38.9824664003869,253.9,19.6577756263214)) ;
#103030=CARTESIAN_POINT('Origin',(38.5004065309378,253.9,19.7905095039363)) ;
#103031=CARTESIAN_POINT('',(38.0323928885057,253.9,19.9664732232009)) ;
#103032=CARTESIAN_POINT('Origin',(38.5004065309378,253.9,19.7905095039363)) ;
#103033=CARTESIAN_POINT('',(38.173903559688,253.75,19.9165880896082)) ;
#103034=CARTESIAN_POINT('Origin',(38.5004065309378,253.75,19.7905095039363)) ;
#103035=CARTESIAN_POINT('Ctrl Pts',(38.1739035596861,253.75,19.9165880896088)) ;
#103036=CARTESIAN_POINT('Ctrl Pts',(38.1725290495197,253.75,19.9170763684267)) ;
#103037=CARTESIAN_POINT('Ctrl Pts',(38.1711545707748,253.750021261236,19.917564504601)) ;
#103038=CARTESIAN_POINT('Ctrl Pts',(38.1697805624967,253.750063777237,19.9180523447824)) ;
#103039=CARTESIAN_POINT('Ctrl Pts',(38.1521290671492,253.750609968276,19.9243194894788)) ;
#103040=CARTESIAN_POINT('Ctrl Pts',(38.1347220873535,253.754658837467,19.9304781840937)) ;
#103041=CARTESIAN_POINT('Ctrl Pts',(38.1184645303644,253.762001431812,19.9362163456665)) ;
#103042=CARTESIAN_POINT('Ctrl Pts',(38.1015160468842,253.769656077527,19.9421983721597)) ;
#103043=CARTESIAN_POINT('Ctrl Pts',(38.0861341004723,253.78074710398,19.9476117259015)) ;
#103044=CARTESIAN_POINT('Ctrl Pts',(38.0731882320495,253.794651469056,19.952161258783)) ;
#103045=CARTESIAN_POINT('Ctrl Pts',(38.0602458273978,253.808552113907,19.9567095744005)) ;
#103046=CARTESIAN_POINT('Ctrl Pts',(38.0499858937768,253.824998688613,19.960307760187)) ;
#103047=CARTESIAN_POINT('Ctrl Pts',(38.0429889324131,253.843066458683,19.9627604607567)) ;
#103048=CARTESIAN_POINT('Ctrl Pts',(38.0359928332805,253.861132002274,19.9652128590818)) ;
#103049=CARTESIAN_POINT('Ctrl Pts',(38.0323928885057,253.880472526098,19.966473223201)) ;
#103050=CARTESIAN_POINT('Ctrl Pts',(38.0323928885057,253.9,19.9664732232009)) ;
#103051=CARTESIAN_POINT('Origin',(39.1300072095089,253.9,22.8591725524954)) ;
#103052=CARTESIAN_POINT('',(38.1565530819608,253.9,20.3485990065702)) ;
#103053=CARTESIAN_POINT('',(38.9873487320647,253.9,22.9055251016516)) ;
#103054=CARTESIAN_POINT('',(38.3418047738312,253.75,20.4333348922484)) ;
#103055=CARTESIAN_POINT('',(39.1300072095089,253.75,22.8591725524954)) ;
#103056=CARTESIAN_POINT('Ctrl Pts',(38.3418047738312,253.75,20.4333348922484)) ;
#103057=CARTESIAN_POINT('Ctrl Pts',(38.3410897979451,253.75,20.4330018626361)) ;
#103058=CARTESIAN_POINT('Ctrl Pts',(38.3403747898355,253.750003330106,20.4326688888987)) ;
#103059=CARTESIAN_POINT('Ctrl Pts',(38.3212338170932,253.750181671152,20.4237569825369)) ;
#103060=CARTESIAN_POINT('Ctrl Pts',(38.3027198224307,253.752566842488,20.4151851106646)) ;
#103061=CARTESIAN_POINT('Ctrl Pts',(38.2675842178248,253.761740190969,20.3990026749412)) ;
#103062=CARTESIAN_POINT('Ctrl Pts',(38.2507597781153,253.768377217198,20.3912950523217)) ;
#103063=CARTESIAN_POINT('Ctrl Pts',(38.2177054917619,253.78721321578,20.3762187794687)) ;
#103064=CARTESIAN_POINT('Ctrl Pts',(38.2015932119542,253.800023548159,20.3689119713107)) ;
#103065=CARTESIAN_POINT('Ctrl Pts',(38.1781795794102,253.828041657271,20.3583294709921)) ;
#103066=CARTESIAN_POINT('Ctrl Pts',(38.1698022074386,253.841958224525,20.3545568129842)) ;
#103067=CARTESIAN_POINT('Ctrl Pts',(38.1592036720168,253.870954690135,20.3497888860605)) ;
#103068=CARTESIAN_POINT('Ctrl Pts',(38.1565530819608,253.885320776746,20.3485990065702)) ;
#103069=CARTESIAN_POINT('Ctrl Pts',(38.1565530819608,253.9,20.3485990065702)) ;
#103070=CARTESIAN_POINT('Origin',(40.2,253.9,25.0213203435596)) ;
#103071=CARTESIAN_POINT('',(37.6207969906631,253.9,20.6215803698081)) ;
#103072=CARTESIAN_POINT('Origin',(40.2,253.9,25.0213203435596)) ;
#103073=CARTESIAN_POINT('',(37.5804615497666,253.75,20.8212586407095)) ;
#103074=CARTESIAN_POINT('Origin',(40.2,253.75,25.0213203435596)) ;
#103075=CARTESIAN_POINT('Ctrl Pts',(37.5804615497666,253.75,20.8212586407095)) ;
#103076=CARTESIAN_POINT('Ctrl Pts',(37.5806123754316,253.75,20.8204844631751)) ;
#103077=CARTESIAN_POINT('Ctrl Pts',(37.5807632652409,253.750003330105,20.8197102924139)) ;
#103078=CARTESIAN_POINT('Ctrl Pts',(37.5848041630341,253.750181671152,20.7989866330484)) ;
#103079=CARTESIAN_POINT('Ctrl Pts',(37.5887516260398,253.752566842487,20.7789700768601)) ;
#103080=CARTESIAN_POINT('Ctrl Pts',(37.5963119507474,253.761740190968,20.7410329785595)) ;
#103081=CARTESIAN_POINT('Ctrl Pts',(37.5999655106015,253.768377217197,20.7228912940061)) ;
#103082=CARTESIAN_POINT('Ctrl Pts',(37.6071973716955,253.78721321578,20.6872882037654)) ;
#103083=CARTESIAN_POINT('Ctrl Pts',(37.6107566001728,253.800023548159,20.6699582615064)) ;
#103084=CARTESIAN_POINT('Ctrl Pts',(37.615957365484,253.828041657271,20.6447959972585)) ;
#103085=CARTESIAN_POINT('Ctrl Pts',(37.6178293167396,253.841958224525,20.6358010482263)) ;
#103086=CARTESIAN_POINT('Ctrl Pts',(37.6202016456472,253.870954690135,20.6244241358249)) ;
#103087=CARTESIAN_POINT('Ctrl Pts',(37.6207969906631,253.885320776746,20.6215803698081)) ;
#103088=CARTESIAN_POINT('Ctrl Pts',(37.6207969906631,253.9,20.6215803698081)) ;
#103089=CARTESIAN_POINT('Origin',(38.8730077853443,253.9,22.6002959107317)) ;
#103090=CARTESIAN_POINT('',(37.3846302685632,253.9,20.2965247632928)) ;
#103091=CARTESIAN_POINT('',(38.9943603345005,253.9,22.5121281228878)) ;
#103092=CARTESIAN_POINT('',(37.2610944621568,253.75,20.3816875553298)) ;
#103093=CARTESIAN_POINT('',(38.8730077853443,253.75,22.6002959107317)) ;
#103094=CARTESIAN_POINT('Ctrl Pts',(37.2610944621568,253.75,20.3816875553298)) ;
#103095=CARTESIAN_POINT('Ctrl Pts',(37.2622974048239,253.75,20.3808625563341)) ;
#103096=CARTESIAN_POINT('Ctrl Pts',(37.263500213621,253.750021261236,20.3800374989151)) ;
#103097=CARTESIAN_POINT('Ctrl Pts',(37.2647025064213,253.750063777237,20.3792126481315)) ;
#103098=CARTESIAN_POINT('Ctrl Pts',(37.280148021633,253.750609968276,20.3686160236467)) ;
#103099=CARTESIAN_POINT('Ctrl Pts',(37.2953620762501,253.754658837467,20.3581534710378)) ;
#103100=CARTESIAN_POINT('Ctrl Pts',(37.3095602987156,253.762001431812,20.3483736378944)) ;
#103101=CARTESIAN_POINT('Ctrl Pts',(37.3243619284479,253.769656077527,20.3381781736817)) ;
#103102=CARTESIAN_POINT('Ctrl Pts',(37.3377827048739,253.78074710398,20.3289158071227)) ;
#103103=CARTESIAN_POINT('Ctrl Pts',(37.3490727448286,253.794651469056,20.3211165278944)) ;
#103104=CARTESIAN_POINT('Ctrl Pts',(37.3603597640425,253.808552113907,20.3133193354259)) ;
#103105=CARTESIAN_POINT('Ctrl Pts',(37.3693013951648,253.824998688613,20.307133835306)) ;
#103106=CARTESIAN_POINT('Ctrl Pts',(37.3753983823083,253.843066458683,20.302914835877)) ;
#103107=CARTESIAN_POINT('Ctrl Pts',(37.3814946181239,253.861132002274,20.2986963563525)) ;
#103108=CARTESIAN_POINT('Ctrl Pts',(37.3846302685631,253.880472526098,20.2965247632926)) ;
#103109=CARTESIAN_POINT('Ctrl Pts',(37.384630268563,253.9,20.2965247632926)) ;
#103110=CARTESIAN_POINT('Origin',(36.9671811123914,253.9,20.5717268744974)) ;
#103111=CARTESIAN_POINT('',(36.5764494676875,253.9,20.8837024854464)) ;
#103112=CARTESIAN_POINT('Origin',(36.9671811123914,253.9,20.5717268744974)) ;
#103113=CARTESIAN_POINT('',(36.6956187595939,253.75,20.7925297017961)) ;
#103114=CARTESIAN_POINT('Origin',(36.9671811123914,253.75,20.5717268744974)) ;
#103115=CARTESIAN_POINT('Ctrl Pts',(36.69561875959,253.75,20.7925297017989)) ;
#103116=CARTESIAN_POINT('Ctrl Pts',(36.6944624091931,253.75,20.7934188295502)) ;
#103117=CARTESIAN_POINT('Ctrl Pts',(36.6933060446003,253.750021261236,20.7943078119297)) ;
#103118=CARTESIAN_POINT('Ctrl Pts',(36.6921500359814,253.750063777237,20.7951963674211)) ;
#103119=CARTESIAN_POINT('Ctrl Pts',(36.677299120528,253.750609968276,20.8066113882631)) ;
#103120=CARTESIAN_POINT('Ctrl Pts',(36.662647240261,253.754658837467,20.8178477074835)) ;
#103121=CARTESIAN_POINT('Ctrl Pts',(36.64895857419,253.762001431812,20.8283288848358)) ;
#103122=CARTESIAN_POINT('Ctrl Pts',(36.6346881563821,253.769656077527,20.8392554995373)) ;
#103123=CARTESIAN_POINT('Ctrl Pts',(36.6217318743169,253.78074710398,20.8491571877365)) ;
#103124=CARTESIAN_POINT('Ctrl Pts',(36.6108255047712,253.794651469056,20.8574845439793)) ;
#103125=CARTESIAN_POINT('Ctrl Pts',(36.5999220533123,253.808552113907,20.865809672171)) ;
#103126=CARTESIAN_POINT('Ctrl Pts',(36.5912761771423,253.824998688613,20.8724022440601)) ;
#103127=CARTESIAN_POINT('Ctrl Pts',(36.5853795976012,253.843066458683,20.8768970808898)) ;
#103128=CARTESIAN_POINT('Ctrl Pts',(36.5794837446919,253.861132002274,20.8813913638237)) ;
#103129=CARTESIAN_POINT('Ctrl Pts',(36.5764494676877,253.880472526098,20.8837024854467)) ;
#103130=CARTESIAN_POINT('Ctrl Pts',(36.5764494676876,253.9,20.8837024854466)) ;
#103131=CARTESIAN_POINT('Origin',(38.5142359724255,253.9,23.2956415537952)) ;
#103132=CARTESIAN_POINT('',(36.8126161897874,253.9,21.2087580919617)) ;
#103133=CARTESIAN_POINT('',(38.3928834232693,253.9,23.3838093416391)) ;
#103134=CARTESIAN_POINT('',(37.0149858472034,253.75,21.2321007871753)) ;
#103135=CARTESIAN_POINT('',(38.5142359724255,253.75,23.2956415537952)) ;
#103136=CARTESIAN_POINT('Ctrl Pts',(37.0149858472034,253.75,21.2321007871753)) ;
#103137=CARTESIAN_POINT('Ctrl Pts',(37.0142029529195,253.75,21.2320049968919)) ;
#103138=CARTESIAN_POINT('Ctrl Pts',(37.0134200452556,253.750003330106,21.2319092697064)) ;
#103139=CARTESIAN_POINT('Ctrl Pts',(36.9924619678835,253.750181671152,21.2293484289546)) ;
#103140=CARTESIAN_POINT('Ctrl Pts',(36.972205258534,253.752566842488,21.226917233338)) ;
#103141=CARTESIAN_POINT('Ctrl Pts',(36.9337886651694,253.761740190968,21.2223843213245)) ;
#103142=CARTESIAN_POINT('Ctrl Pts',(36.9154058857743,253.768377217198,21.220252974398)) ;
#103143=CARTESIAN_POINT('Ctrl Pts',(36.8793105668223,253.78721321578,21.2161289230799)) ;
#103144=CARTESIAN_POINT('Ctrl Pts',(36.8617289502234,253.800023548159,21.2141587038466)) ;
#103145=CARTESIAN_POINT('Ctrl Pts',(36.8361910899809,253.828041657271,21.211329358316)) ;
#103146=CARTESIAN_POINT('Ctrl Pts',(36.8270579203394,253.841958224525,21.2103300976413)) ;
#103147=CARTESIAN_POINT('Ctrl Pts',(36.815504743716,253.870954690135,21.2090706572321)) ;
#103148=CARTESIAN_POINT('Ctrl Pts',(36.8126161897874,253.885320776746,21.2087580919617)) ;
#103149=CARTESIAN_POINT('Ctrl Pts',(36.8126161897874,253.9,21.2087580919617)) ;
#103150=CARTESIAN_POINT('Origin',(40.2,253.9,25.0213203435596)) ;
#103151=CARTESIAN_POINT('',(36.3874377484021,253.9,21.633936533347)) ;
#103152=CARTESIAN_POINT('Origin',(40.2,253.9,25.0213203435596)) ;
#103153=CARTESIAN_POINT('',(36.4107804436157,253.75,21.836306190763)) ;
#103154=CARTESIAN_POINT('Origin',(40.2,253.75,25.0213203435596)) ;
#103155=CARTESIAN_POINT('Ctrl Pts',(36.4107804436157,253.75,21.836306190763)) ;
#103156=CARTESIAN_POINT('Ctrl Pts',(36.410684653332,253.75,21.835523296477)) ;
#103157=CARTESIAN_POINT('Ctrl Pts',(36.410588926147,253.750003330105,21.8347403888173)) ;
#103158=CARTESIAN_POINT('Ctrl Pts',(36.4080280853953,253.750181671152,21.8137823114414)) ;
#103159=CARTESIAN_POINT('Ctrl Pts',(36.4055968897783,253.752566842488,21.7935256020932)) ;
#103160=CARTESIAN_POINT('Ctrl Pts',(36.4010639777649,253.761740190968,21.7551090087289)) ;
#103161=CARTESIAN_POINT('Ctrl Pts',(36.3989326308384,253.768377217198,21.7367262293338)) ;
#103162=CARTESIAN_POINT('Ctrl Pts',(36.3948085795202,253.78721321578,21.7006309103819)) ;
#103163=CARTESIAN_POINT('Ctrl Pts',(36.392838360287,253.800023548159,21.683049293783)) ;
#103164=CARTESIAN_POINT('Ctrl Pts',(36.3900090147564,253.828041657271,21.6575114335404)) ;
#103165=CARTESIAN_POINT('Ctrl Pts',(36.3890097540816,253.841958224525,21.648378263899)) ;
#103166=CARTESIAN_POINT('Ctrl Pts',(36.3877503136725,253.870954690135,21.6368250872756)) ;
#103167=CARTESIAN_POINT('Ctrl Pts',(36.3874377484021,253.885320776746,21.633936533347)) ;
#103168=CARTESIAN_POINT('Ctrl Pts',(36.3874377484021,253.9,21.633936533347)) ;
#103169=CARTESIAN_POINT('Origin',(38.1898177136379,253.9,23.1288524263407)) ;
#103170=CARTESIAN_POINT('',(36.0623821418868,253.9,21.3977698112471)) ;
#103171=CARTESIAN_POINT('',(38.2779855014818,253.9,23.0074998771845)) ;
#103172=CARTESIAN_POINT('',(35.9712093582363,253.75,21.5169391031534)) ;
#103173=CARTESIAN_POINT('',(38.1898177136379,253.75,23.1288524263407)) ;
#103174=CARTESIAN_POINT('Ctrl Pts',(35.9712093582363,253.75,21.5169391031534)) ;
#103175=CARTESIAN_POINT('Ctrl Pts',(35.9720984859888,253.75,21.5157827527548)) ;
#103176=CARTESIAN_POINT('Ctrl Pts',(35.9729874683704,253.750021261236,21.5146263881627)) ;
#103177=CARTESIAN_POINT('Ctrl Pts',(35.9738760238622,253.750063777237,21.5134703795415)) ;
#103178=CARTESIAN_POINT('Ctrl Pts',(35.9852910446951,253.750609968276,21.4986194640776)) ;
#103179=CARTESIAN_POINT('Ctrl Pts',(35.9965273639257,253.754658837467,21.4839675838214)) ;
#103180=CARTESIAN_POINT('Ctrl Pts',(36.0070085412772,253.762001431812,21.4702789177503)) ;
#103181=CARTESIAN_POINT('Ctrl Pts',(36.017935155978,253.769656077527,21.4560084999421)) ;
#103182=CARTESIAN_POINT('Ctrl Pts',(36.0278368441765,253.78074710398,21.4430522178762)) ;
#103183=CARTESIAN_POINT('Ctrl Pts',(36.0361642004193,253.794651469056,21.4321458483306)) ;
#103184=CARTESIAN_POINT('Ctrl Pts',(36.0444893286111,253.808552113907,21.4212423968717)) ;
#103185=CARTESIAN_POINT('Ctrl Pts',(36.0510819005004,253.824998688613,21.4125965207018)) ;
#103186=CARTESIAN_POINT('Ctrl Pts',(36.0555767373303,253.843066458683,21.4066999411609)) ;
#103187=CARTESIAN_POINT('Ctrl Pts',(36.0600710202644,253.861132002274,21.4008040882518)) ;
#103188=CARTESIAN_POINT('Ctrl Pts',(36.0623821418865,253.880472526098,21.3977698112469)) ;
#103189=CARTESIAN_POINT('Ctrl Pts',(36.0623821418867,253.9,21.3977698112471)) ;
#103190=CARTESIAN_POINT('Origin',(35.7504065309378,253.9,21.788501455951)) ;
#103191=CARTESIAN_POINT('',(35.4752044197332,253.9,22.2059506121228)) ;
#103192=CARTESIAN_POINT('Origin',(35.7504065309378,253.9,21.788501455951)) ;
#103193=CARTESIAN_POINT('',(35.5603672117704,253.75,22.0824148057165)) ;
#103194=CARTESIAN_POINT('Origin',(35.7504065309378,253.75,21.788501455951)) ;
#103195=CARTESIAN_POINT('Ctrl Pts',(35.5603672117688,253.75,22.0824148057187)) ;
#103196=CARTESIAN_POINT('Ctrl Pts',(35.5595422127734,253.75,22.0836177483853)) ;
#103197=CARTESIAN_POINT('Ctrl Pts',(35.5587171553563,253.750021261236,22.084820557182)) ;
#103198=CARTESIAN_POINT('Ctrl Pts',(35.5578923045725,253.750063777237,22.0860228499814)) ;
#103199=CARTESIAN_POINT('Ctrl Pts',(35.5472956800797,253.750609968276,22.1014683651895)) ;
#103200=CARTESIAN_POINT('Ctrl Pts',(35.5368331274791,253.754658837467,22.1166824198107)) ;
#103201=CARTESIAN_POINT('Ctrl Pts',(35.5270532943355,253.762001431812,22.1308806422758)) ;
#103202=CARTESIAN_POINT('Ctrl Pts',(35.5168578301224,253.769656077527,22.1456822720078)) ;
#103203=CARTESIAN_POINT('Ctrl Pts',(35.5075954635634,253.78074710398,22.1591030484337)) ;
#103204=CARTESIAN_POINT('Ctrl Pts',(35.4997961843351,253.794651469056,22.1703930883885)) ;
#103205=CARTESIAN_POINT('Ctrl Pts',(35.4919989918666,253.808552113907,22.1816801076023)) ;
#103206=CARTESIAN_POINT('Ctrl Pts',(35.4858134917463,253.824998688613,22.1906217387244)) ;
#103207=CARTESIAN_POINT('Ctrl Pts',(35.4815944923174,253.843066458683,22.1967187258679)) ;
#103208=CARTESIAN_POINT('Ctrl Pts',(35.4773760127931,253.861132002274,22.2028149616837)) ;
#103209=CARTESIAN_POINT('Ctrl Pts',(35.4752044197329,253.880472526098,22.2059506121226)) ;
#103210=CARTESIAN_POINT('Ctrl Pts',(35.475204419733,253.9,22.2059506121227)) ;
#103211=CARTESIAN_POINT('Origin',(38.0634790637697,253.9,23.9010320185483)) ;
#103212=CARTESIAN_POINT('',(35.8002600262485,253.9,22.4421173342227)) ;
#103213=CARTESIAN_POINT('',(37.9753112759259,253.9,24.0223845677046)) ;
#103214=CARTESIAN_POINT('',(35.9999382971499,253.75,22.4017818933262)) ;
#103215=CARTESIAN_POINT('',(38.0634790637697,253.75,23.9010320185483)) ;
#103216=CARTESIAN_POINT('Ctrl Pts',(35.9999382971499,253.75,22.4017818933262)) ;
#103217=CARTESIAN_POINT('Ctrl Pts',(35.999164119612,253.75,22.4019327189919)) ;
#103218=CARTESIAN_POINT('Ctrl Pts',(35.9983899488536,253.750003330105,22.4020836088006)) ;
#103219=CARTESIAN_POINT('Ctrl Pts',(35.9776662894844,253.750181671152,22.4061245065949)) ;
#103220=CARTESIAN_POINT('Ctrl Pts',(35.9576497332976,253.752566842488,22.4100719696)) ;
#103221=CARTESIAN_POINT('Ctrl Pts',(35.9197126349982,253.761740190968,22.4176322943074)) ;
#103222=CARTESIAN_POINT('Ctrl Pts',(35.9015709504457,253.768377217198,22.4212858541613)) ;
#103223=CARTESIAN_POINT('Ctrl Pts',(35.8659678602058,253.78721321578,22.4285177152552)) ;
#103224=CARTESIAN_POINT('Ctrl Pts',(35.8486379179467,253.800023548159,22.4320769437325)) ;
#103225=CARTESIAN_POINT('Ctrl Pts',(35.823475653699,253.828041657271,22.4372777090437)) ;
#103226=CARTESIAN_POINT('Ctrl Pts',(35.8144807046667,253.841958224525,22.4391496602992)) ;
#103227=CARTESIAN_POINT('Ctrl Pts',(35.8031037922653,253.870954690135,22.4415219892068)) ;
#103228=CARTESIAN_POINT('Ctrl Pts',(35.8002600262485,253.885320776746,22.4421173342227)) ;
#103229=CARTESIAN_POINT('Ctrl Pts',(35.8002600262485,253.9,22.4421173342227)) ;
#103230=CARTESIAN_POINT('Origin',(40.2,253.9,25.0213203435596)) ;
#103231=CARTESIAN_POINT('',(35.5272786630106,253.9,22.9778734255204)) ;
#103232=CARTESIAN_POINT('Origin',(40.2,253.9,25.0213203435596)) ;
#103233=CARTESIAN_POINT('',(35.6120145486888,253.75,23.1631251173908)) ;
#103234=CARTESIAN_POINT('Origin',(40.2,253.75,25.0213203435596)) ;
#103235=CARTESIAN_POINT('Ctrl Pts',(35.6120145486888,253.75,23.1631251173908)) ;
#103236=CARTESIAN_POINT('Ctrl Pts',(35.611681519077,253.75,23.162410141506)) ;
#103237=CARTESIAN_POINT('Ctrl Pts',(35.6113485453403,253.750003330106,23.1616951333977)) ;
#103238=CARTESIAN_POINT('Ctrl Pts',(35.6024366389787,253.750181671152,23.1425541606558)) ;
#103239=CARTESIAN_POINT('Ctrl Pts',(35.593864767106,253.752566842488,23.1240401659928)) ;
#103240=CARTESIAN_POINT('Ctrl Pts',(35.5776823313821,253.761740190968,23.0889045613856)) ;
#103241=CARTESIAN_POINT('Ctrl Pts',(35.5699747087623,253.768377217198,23.0720801216755)) ;
#103242=CARTESIAN_POINT('Ctrl Pts',(35.5548984359091,253.78721321578,23.0390258353216)) ;
#103243=CARTESIAN_POINT('Ctrl Pts',(35.5475916277511,253.800023548159,23.0229135555139)) ;
#103244=CARTESIAN_POINT('Ctrl Pts',(35.5370091274324,253.828041657271,22.9994999229698)) ;
#103245=CARTESIAN_POINT('Ctrl Pts',(35.5332364694246,253.841958224525,22.9911225509982)) ;
#103246=CARTESIAN_POINT('Ctrl Pts',(35.5284685425009,253.870954690135,22.9805240155764)) ;
#103247=CARTESIAN_POINT('Ctrl Pts',(35.5272786630106,253.885320776746,22.9778734255204)) ;
#103248=CARTESIAN_POINT('Ctrl Pts',(35.5272786630106,253.9,22.9778734255204)) ;
#103249=CARTESIAN_POINT('Origin',(37.7033982898842,253.9,23.8426568872864)) ;
#103250=CARTESIAN_POINT('',(35.1451528796413,253.9,22.8537132320653)) ;
#103251=CARTESIAN_POINT('',(37.7497508390405,253.9,23.6999984098422)) ;
#103252=CARTESIAN_POINT('',(35.0952677460482,253.75,22.9952239032475)) ;
#103253=CARTESIAN_POINT('',(37.7033982898842,253.75,23.8426568872864)) ;
#103254=CARTESIAN_POINT('Ctrl Pts',(35.0952677460482,253.75,22.9952239032474)) ;
#103255=CARTESIAN_POINT('Ctrl Pts',(35.0957560248663,253.75,22.9938493930805)) ;
#103256=CARTESIAN_POINT('Ctrl Pts',(35.0962441610409,253.750021261236,22.9924749143349)) ;
#103257=CARTESIAN_POINT('Ctrl Pts',(35.0967320012226,253.750063777237,22.9911009060562)) ;
#103258=CARTESIAN_POINT('Ctrl Pts',(35.1029991459191,253.750609968276,22.9734494107094)) ;
#103259=CARTESIAN_POINT('Ctrl Pts',(35.1091578405339,253.754658837467,22.9560424309131)) ;
#103260=CARTESIAN_POINT('Ctrl Pts',(35.1148960021067,253.762001431812,22.9397848739239)) ;
#103261=CARTESIAN_POINT('Ctrl Pts',(35.1208780285998,253.769656077527,22.9228363904437)) ;
#103262=CARTESIAN_POINT('Ctrl Pts',(35.1262913823416,253.78074710398,22.9074544440318)) ;
#103263=CARTESIAN_POINT('Ctrl Pts',(35.1308409152232,253.794651469056,22.894508575609)) ;
#103264=CARTESIAN_POINT('Ctrl Pts',(35.1353892308407,253.808552113907,22.8815661709573)) ;
#103265=CARTESIAN_POINT('Ctrl Pts',(35.1389874166273,253.824998688613,22.8713062373364)) ;
#103266=CARTESIAN_POINT('Ctrl Pts',(35.141440117197,253.843066458683,22.8643092759727)) ;
#103267=CARTESIAN_POINT('Ctrl Pts',(35.1438925155221,253.861132002274,22.8573131768401)) ;
#103268=CARTESIAN_POINT('Ctrl Pts',(35.1451528796412,253.880472526098,22.8537132320653)) ;
#103269=CARTESIAN_POINT('Ctrl Pts',(35.1451528796412,253.9,22.8537132320653)) ;
#103270=CARTESIAN_POINT('Origin',(34.9691891603767,253.9,23.3217268744974)) ;
#103271=CARTESIAN_POINT('',(34.8364552827619,253.9,23.8037867439466)) ;
#103272=CARTESIAN_POINT('Origin',(34.9691891603767,253.9,23.3217268744974)) ;
#103273=CARTESIAN_POINT('',(34.8792752474816,253.75,23.6599804602403)) ;
#103274=CARTESIAN_POINT('Origin',(34.9691891603767,253.75,23.3217268744974)) ;
#103275=CARTESIAN_POINT('Ctrl Pts',(34.8792752474796,253.75,23.6599804602464)) ;
#103276=CARTESIAN_POINT('Ctrl Pts',(34.8788623565368,253.75,23.6613794654168)) ;
#103277=CARTESIAN_POINT('Ctrl Pts',(34.8784493686624,253.750021261236,23.6627783613227)) ;
#103278=CARTESIAN_POINT('Ctrl Pts',(34.8780364178575,253.750063777237,23.6641767026329)) ;
#103279=CARTESIAN_POINT('Ctrl Pts',(34.8727313557742,253.750609968276,23.6821407975714)) ;
#103280=CARTESIAN_POINT('Ctrl Pts',(34.8674822783712,253.754658837467,23.6998433299148)) ;
#103281=CARTESIAN_POINT('Ctrl Pts',(34.8625685963638,253.762001431812,23.7163687765538)) ;
#103282=CARTESIAN_POINT('Ctrl Pts',(34.8574460888193,253.769656077527,23.7335965346698)) ;
#103283=CARTESIAN_POINT('Ctrl Pts',(34.8527843027414,253.78074710398,23.7492226802185)) ;
#103284=CARTESIAN_POINT('Ctrl Pts',(34.8488555616221,253.794651469056,23.7623702561121)) ;
#103285=CARTESIAN_POINT('Ctrl Pts',(34.844927871669,253.808552113907,23.7755143142662)) ;
#103286=CARTESIAN_POINT('Ctrl Pts',(34.8418082274473,253.824998688613,23.785929735467)) ;
#103287=CARTESIAN_POINT('Ctrl Pts',(34.8396797931899,253.843066458683,23.7930320573424)) ;
#103288=CARTESIAN_POINT('Ctrl Pts',(34.837551621218,253.861132002274,23.8001335040032)) ;
#103289=CARTESIAN_POINT('Ctrl Pts',(34.8364552827618,253.880472526098,23.8037867439466)) ;
#103290=CARTESIAN_POINT('Ctrl Pts',(34.8364552827619,253.9,23.8037867439466)) ;
#103291=CARTESIAN_POINT('Origin',(37.8218597103689,253.9,24.6160841100613)) ;
#103292=CARTESIAN_POINT('',(35.2185810661312,253.9,23.9279469374017)) ;
#103293=CARTESIAN_POINT('',(37.7755071612126,253.9,24.7587425875056)) ;
#103294=CARTESIAN_POINT('',(35.3960220501219,253.75,23.8278816743835)) ;
#103295=CARTESIAN_POINT('',(37.8218597103689,253.75,24.6160841100613)) ;
#103296=CARTESIAN_POINT('Ctrl Pts',(35.3960220501219,253.75,23.8278816743835)) ;
#103297=CARTESIAN_POINT('Ctrl Pts',(35.3953323712255,253.75,23.8282643521305)) ;
#103298=CARTESIAN_POINT('Ctrl Pts',(35.3946427185925,253.750003330106,23.8286470887893)) ;
#103299=CARTESIAN_POINT('Ctrl Pts',(35.3761820534012,253.750181671152,23.8388941738976)) ;
#103300=CARTESIAN_POINT('Ctrl Pts',(35.3583650103588,253.752566842488,23.8488338903421)) ;
#103301=CARTESIAN_POINT('Ctrl Pts',(35.3246209546295,253.761740190968,23.8677473945122)) ;
#103302=CARTESIAN_POINT('Ctrl Pts',(35.3084961994041,253.768377217198,23.8768282252524)) ;
#103303=CARTESIAN_POINT('Ctrl Pts',(35.27687041641,253.78721321578,23.8947080938071)) ;
#103304=CARTESIAN_POINT('Ctrl Pts',(35.2614885239839,253.800023548159,23.903448367913)) ;
#103305=CARTESIAN_POINT('Ctrl Pts',(35.2391649134711,253.828041657271,23.9161701569215)) ;
#103306=CARTESIAN_POINT('Ctrl Pts',(35.2311886733309,253.841958224525,23.9207300804757)) ;
#103307=CARTESIAN_POINT('Ctrl Pts',(35.2211016766049,253.870954690135,23.9265019586177)) ;
#103308=CARTESIAN_POINT('Ctrl Pts',(35.2185810661312,253.885320776746,23.9279469374017)) ;
#103309=CARTESIAN_POINT('Ctrl Pts',(35.2185810661312,253.9,23.9279469374017)) ;
#103310=CARTESIAN_POINT('Origin',(40.2,253.9,25.0213203435596)) ;
#103311=CARTESIAN_POINT('',(35.1245180988476,253.9,24.5218371395634)) ;
#103312=CARTESIAN_POINT('Origin',(40.2,253.9,25.0213203435596)) ;
#103313=CARTESIAN_POINT('',(35.2623526361106,253.75,24.6718371395634)) ;
#103314=CARTESIAN_POINT('Origin',(40.2,253.75,25.0213203435596)) ;
#103315=CARTESIAN_POINT('Ctrl Pts',(35.2623526361106,253.75,24.6718371395634)) ;
#103316=CARTESIAN_POINT('Ctrl Pts',(35.2618149664292,253.75,24.6712600688988)) ;
#103317=CARTESIAN_POINT('Ctrl Pts',(35.2612773399305,253.750003330106,24.6706829503216)) ;
#103318=CARTESIAN_POINT('Ctrl Pts',(35.2468867274465,253.750181671152,24.655232733985)) ;
#103319=CARTESIAN_POINT('Ctrl Pts',(35.2330132538605,253.752566842488,24.6402737328005)) ;
#103320=CARTESIAN_POINT('Ctrl Pts',(35.2067653439847,253.761740190968,24.6118584347341)) ;
#103321=CARTESIAN_POINT('Ctrl Pts',(35.1942359214757,253.768377217198,24.5982392280904)) ;
#103322=CARTESIAN_POINT('Ctrl Pts',(35.1696831977168,253.78721321578,24.5714615581854)) ;
#103323=CARTESIAN_POINT('Ctrl Pts',(35.1577550419262,253.800023548159,24.5583957973774)) ;
#103324=CARTESIAN_POINT('Ctrl Pts',(35.1404552756832,253.828041657271,24.5393982820177)) ;
#103325=CARTESIAN_POINT('Ctrl Pts',(35.1342785143937,253.841958224525,24.5325967432531)) ;
#103326=CARTESIAN_POINT('Ctrl Pts',(35.1264688188629,253.870954690135,24.5239903075244)) ;
#103327=CARTESIAN_POINT('Ctrl Pts',(35.1245180988476,253.885320776746,24.5218371395634)) ;
#103328=CARTESIAN_POINT('Ctrl Pts',(35.1245180988476,253.9,24.5218371395634)) ;
#103329=CARTESIAN_POINT('Origin',(37.4613636363637,253.9,24.6718371395634)) ;
#103330=CARTESIAN_POINT('',(34.7227272727273,253.9,24.5218371395634)) ;
#103331=CARTESIAN_POINT('',(37.4613636363637,253.9,24.5218371395634)) ;
#103332=CARTESIAN_POINT('',(34.7190128936382,253.75,24.6718371395634)) ;
#103333=CARTESIAN_POINT('',(37.4613636363637,253.75,24.6718371395634)) ;
#103334=CARTESIAN_POINT('Ctrl Pts',(34.7190128936382,253.75,24.6718371395634)) ;
#103335=CARTESIAN_POINT('Ctrl Pts',(34.7190525273894,253.75,24.6703790162596)) ;
#103336=CARTESIAN_POINT('Ctrl Pts',(34.7190920351881,253.750021261236,24.6689209669185)) ;
#103337=CARTESIAN_POINT('Ctrl Pts',(34.7191314068632,253.750063777237,24.6674634564849)) ;
#103338=CARTESIAN_POINT('Ctrl Pts',(34.7196372036259,253.750609968276,24.6487392325953)) ;
#103339=CARTESIAN_POINT('Ctrl Pts',(34.720115417695,253.754658837467,24.6302810697322)) ;
#103340=CARTESIAN_POINT('Ctrl Pts',(34.7205488722535,253.762001431812,24.6130460247761)) ;
#103341=CARTESIAN_POINT('Ctrl Pts',(34.7210007481061,253.769656077527,24.5950785112738)) ;
#103342=CARTESIAN_POINT('Ctrl Pts',(34.7213958706093,253.78074710398,24.5787765926027)) ;
#103343=CARTESIAN_POINT('Ctrl Pts',(34.7217222401528,253.794651469056,24.5650584571033)) ;
#103344=CARTESIAN_POINT('Ctrl Pts',(34.7220485223735,253.808552113907,24.5513439920011)) ;
#103345=CARTESIAN_POINT('Ctrl Pts',(34.7223001065627,253.824998688613,24.5404743147171)) ;
#103346=CARTESIAN_POINT('Ctrl Pts',(34.7224705834518,253.843066458683,24.5330618828598)) ;
#103347=CARTESIAN_POINT('Ctrl Pts',(34.7226410393332,253.861132002274,24.5256503644317)) ;
#103348=CARTESIAN_POINT('Ctrl Pts',(34.7227272727271,253.880472526098,24.5218371395634)) ;
#103349=CARTESIAN_POINT('Ctrl Pts',(34.7227272727271,253.9,24.5218371395634)) ;
#103350=CARTESIAN_POINT('Origin',(34.7,253.9,25.0213203435596)) ;
#103351=CARTESIAN_POINT('',(34.7227272727273,253.9,25.5208035475559)) ;
#103352=CARTESIAN_POINT('Origin',(34.7,253.9,25.0213203435596)) ;
#103353=CARTESIAN_POINT('',(34.7190128936384,253.75,25.3708035475559)) ;
#103354=CARTESIAN_POINT('Origin',(34.7,253.75,25.0213203435596)) ;
#103355=CARTESIAN_POINT('Ctrl Pts',(34.7190128936384,253.75,25.3708035475559)) ;
#103356=CARTESIAN_POINT('Ctrl Pts',(34.7190525273896,253.75,25.3722616708596)) ;
#103357=CARTESIAN_POINT('Ctrl Pts',(34.7190920351885,253.750021261236,25.3737197202007)) ;
#103358=CARTESIAN_POINT('Ctrl Pts',(34.7191314068636,253.750063777237,25.3751772306343)) ;
#103359=CARTESIAN_POINT('Ctrl Pts',(34.7196372036263,253.750609968276,25.3939014545242)) ;
#103360=CARTESIAN_POINT('Ctrl Pts',(34.7201154176943,253.754658837467,25.4123596173871)) ;
#103361=CARTESIAN_POINT('Ctrl Pts',(34.720548872253,253.762001431812,25.4295946623432)) ;
#103362=CARTESIAN_POINT('Ctrl Pts',(34.7210007481058,253.769656077527,25.4475621758457)) ;
#103363=CARTESIAN_POINT('Ctrl Pts',(34.7213958706092,253.78074710398,25.4638640945166)) ;
#103364=CARTESIAN_POINT('Ctrl Pts',(34.7217222401529,253.794651469056,25.4775822300161)) ;
#103365=CARTESIAN_POINT('Ctrl Pts',(34.7220485223737,253.808552113907,25.4912966951182)) ;
#103366=CARTESIAN_POINT('Ctrl Pts',(34.7223001065631,253.824998688613,25.5021663724021)) ;
#103367=CARTESIAN_POINT('Ctrl Pts',(34.7224705834521,253.843066458683,25.5095788042595)) ;
#103368=CARTESIAN_POINT('Ctrl Pts',(34.7226410393334,253.861132002274,25.5169903226876)) ;
#103369=CARTESIAN_POINT('Ctrl Pts',(34.7227272727275,253.880472526098,25.5208035475559)) ;
#103370=CARTESIAN_POINT('Ctrl Pts',(34.7227272727275,253.9,25.5208035475559)) ;
#103371=CARTESIAN_POINT('Origin',(37.8130292979948,253.9,25.3708035475559)) ;
#103372=CARTESIAN_POINT('',(35.1245180988476,253.9,25.5208035475559)) ;
#103373=CARTESIAN_POINT('',(37.8130292979948,253.9,25.5208035475559)) ;
#103374=CARTESIAN_POINT('',(35.2623526361106,253.75,25.3708035475559)) ;
#103375=CARTESIAN_POINT('',(37.8130292979948,253.75,25.3708035475559)) ;
#103376=CARTESIAN_POINT('Ctrl Pts',(35.2623526361106,253.75,25.3708035475559)) ;
#103377=CARTESIAN_POINT('Ctrl Pts',(35.2618149664292,253.75,25.3713806182205)) ;
#103378=CARTESIAN_POINT('Ctrl Pts',(35.2612773399305,253.750003330106,25.3719577367977)) ;
#103379=CARTESIAN_POINT('Ctrl Pts',(35.2468867274466,253.750181671152,25.3874079531342)) ;
#103380=CARTESIAN_POINT('Ctrl Pts',(35.2330132538606,253.752566842488,25.4023669543188)) ;
#103381=CARTESIAN_POINT('Ctrl Pts',(35.2067653439847,253.761740190968,25.4307822523853)) ;
#103382=CARTESIAN_POINT('Ctrl Pts',(35.1942359214756,253.768377217198,25.4444014590289)) ;
#103383=CARTESIAN_POINT('Ctrl Pts',(35.1696831977168,253.78721321578,25.4711791289339)) ;
#103384=CARTESIAN_POINT('Ctrl Pts',(35.1577550419262,253.800023548159,25.4842448897419)) ;
#103385=CARTESIAN_POINT('Ctrl Pts',(35.1404552756832,253.828041657271,25.5032424051016)) ;
#103386=CARTESIAN_POINT('Ctrl Pts',(35.1342785143937,253.841958224525,25.5100439438662)) ;
#103387=CARTESIAN_POINT('Ctrl Pts',(35.1264688188629,253.870954690135,25.5186503795949)) ;
#103388=CARTESIAN_POINT('Ctrl Pts',(35.1245180988476,253.885320776746,25.5208035475559)) ;
#103389=CARTESIAN_POINT('Ctrl Pts',(35.1245180988476,253.9,25.5208035475559)) ;
#103390=CARTESIAN_POINT('Origin',(40.2,253.9,25.0213203435596)) ;
#103391=CARTESIAN_POINT('',(35.2185810661312,253.9,26.1146937497175)) ;
#103392=CARTESIAN_POINT('Origin',(40.2,253.9,25.0213203435596)) ;
#103393=CARTESIAN_POINT('',(35.3960220501219,253.75,26.2147590127358)) ;
#103394=CARTESIAN_POINT('Origin',(40.2,253.75,25.0213203435596)) ;
#103395=CARTESIAN_POINT('Ctrl Pts',(35.3960220501219,253.75,26.2147590127358)) ;
#103396=CARTESIAN_POINT('Ctrl Pts',(35.3953323712267,253.75,26.2143763349894)) ;
#103397=CARTESIAN_POINT('Ctrl Pts',(35.3946427185949,253.750003330105,26.2139935983313)) ;
#103398=CARTESIAN_POINT('Ctrl Pts',(35.3761820534042,253.750181671152,26.2037465132234)) ;
#103399=CARTESIAN_POINT('Ctrl Pts',(35.3583650103612,253.752566842487,26.1938067967784)) ;
#103400=CARTESIAN_POINT('Ctrl Pts',(35.3246209546306,253.761740190968,26.1748932926076)) ;
#103401=CARTESIAN_POINT('Ctrl Pts',(35.3084961994046,253.768377217198,26.1658124618672)) ;
#103402=CARTESIAN_POINT('Ctrl Pts',(35.2768704164101,253.78721321578,26.1479325933122)) ;
#103403=CARTESIAN_POINT('Ctrl Pts',(35.2614885239839,253.800023548159,26.1391923192062)) ;
#103404=CARTESIAN_POINT('Ctrl Pts',(35.2391649134711,253.828041657271,26.1264705301977)) ;
#103405=CARTESIAN_POINT('Ctrl Pts',(35.2311886733309,253.841958224525,26.1219106066435)) ;
#103406=CARTESIAN_POINT('Ctrl Pts',(35.2211016766049,253.870954690135,26.1161387285016)) ;
#103407=CARTESIAN_POINT('Ctrl Pts',(35.2185810661312,253.885320776746,26.1146937497175)) ;
#103408=CARTESIAN_POINT('Ctrl Pts',(35.2185810661312,253.9,26.1146937497175)) ;
#103409=CARTESIAN_POINT('Origin',(37.4874057913173,253.9,25.5352272428401)) ;
#103410=CARTESIAN_POINT('',(34.8364552827619,253.9,26.2388539431727)) ;
#103411=CARTESIAN_POINT('',(37.4410532421611,253.9,25.3925687653958)) ;
#103412=CARTESIAN_POINT('',(34.8792752474813,253.75,26.3826602268791)) ;
#103413=CARTESIAN_POINT('',(37.4874057913173,253.75,25.5352272428401)) ;
#103414=CARTESIAN_POINT('Ctrl Pts',(34.8792752474813,253.75,26.3826602268791)) ;
#103415=CARTESIAN_POINT('Ctrl Pts',(34.8788623565379,253.75,26.3812612217066)) ;
#103416=CARTESIAN_POINT('Ctrl Pts',(34.8784493686629,253.750021261236,26.3798623257986)) ;
#103417=CARTESIAN_POINT('Ctrl Pts',(34.8780364178574,253.750063777237,26.3784639844864)) ;
#103418=CARTESIAN_POINT('Ctrl Pts',(34.872731355774,253.750609968276,26.3604998895479)) ;
#103419=CARTESIAN_POINT('Ctrl Pts',(34.8674822783721,253.754658837467,26.3427973572042)) ;
#103420=CARTESIAN_POINT('Ctrl Pts',(34.8625685963644,253.762001431812,26.3262719105654)) ;
#103421=CARTESIAN_POINT('Ctrl Pts',(34.8574460888198,253.769656077527,26.3090441524495)) ;
#103422=CARTESIAN_POINT('Ctrl Pts',(34.8527843027409,253.78074710398,26.2934180069009)) ;
#103423=CARTESIAN_POINT('Ctrl Pts',(34.8488555616216,253.794651469056,26.2802704310073)) ;
#103424=CARTESIAN_POINT('Ctrl Pts',(34.8449278716686,253.808552113907,26.2671263728532)) ;
#103425=CARTESIAN_POINT('Ctrl Pts',(34.8418082274471,253.824998688613,26.2567109516523)) ;
#103426=CARTESIAN_POINT('Ctrl Pts',(34.8396797931898,253.843066458683,26.2496086297769)) ;
#103427=CARTESIAN_POINT('Ctrl Pts',(34.8375516212181,253.861132002274,26.242507183116)) ;
#103428=CARTESIAN_POINT('Ctrl Pts',(34.8364552827617,253.880472526098,26.2388539431727)) ;
#103429=CARTESIAN_POINT('Ctrl Pts',(34.8364552827617,253.9,26.2388539431727)) ;
#103430=CARTESIAN_POINT('Origin',(34.9691891603767,253.9,26.7209138126218)) ;
#103431=CARTESIAN_POINT('',(35.1451528796413,253.9,27.188927455054)) ;
#103432=CARTESIAN_POINT('Origin',(34.9691891603767,253.9,26.7209138126218)) ;
#103433=CARTESIAN_POINT('',(35.0952677460484,253.75,27.0474167838717)) ;
#103434=CARTESIAN_POINT('Origin',(34.9691891603767,253.75,26.7209138126218)) ;
#103435=CARTESIAN_POINT('Ctrl Pts',(35.0952677460487,253.75,27.0474167838725)) ;
#103436=CARTESIAN_POINT('Ctrl Pts',(35.0957560248667,253.75,27.0487912940392)) ;
#103437=CARTESIAN_POINT('Ctrl Pts',(35.0962441610412,253.750021261236,27.0501657727845)) ;
#103438=CARTESIAN_POINT('Ctrl Pts',(35.0967320012228,253.750063777237,27.051539781063)) ;
#103439=CARTESIAN_POINT('Ctrl Pts',(35.1029991459191,253.750609968276,27.0691912764102)) ;
#103440=CARTESIAN_POINT('Ctrl Pts',(35.1091578405316,253.754658837467,27.086598256207)) ;
#103441=CARTESIAN_POINT('Ctrl Pts',(35.114896002105,253.762001431812,27.1028558131961)) ;
#103442=CARTESIAN_POINT('Ctrl Pts',(35.1208780285987,253.769656077527,27.1198042966762)) ;
#103443=CARTESIAN_POINT('Ctrl Pts',(35.1262913823415,253.78074710398,27.1351862430875)) ;
#103444=CARTESIAN_POINT('Ctrl Pts',(35.1308409152232,253.794651469056,27.1481321115102)) ;
#103445=CARTESIAN_POINT('Ctrl Pts',(35.1353892308407,253.808552113907,27.1610745161619)) ;
#103446=CARTESIAN_POINT('Ctrl Pts',(35.1389874166275,253.824998688613,27.1713344497828)) ;
#103447=CARTESIAN_POINT('Ctrl Pts',(35.1414401171972,253.843066458683,27.1783314111465)) ;
#103448=CARTESIAN_POINT('Ctrl Pts',(35.1438925155223,253.861132002274,27.1853275102791)) ;
#103449=CARTESIAN_POINT('Ctrl Pts',(35.1451528796413,253.880472526098,27.1889274550539)) ;
#103450=CARTESIAN_POINT('Ctrl Pts',(35.1451528796413,253.9,27.1889274550539)) ;
#103451=CARTESIAN_POINT('Origin',(38.0378522089358,253.9,26.0913131340507)) ;
#103452=CARTESIAN_POINT('',(35.5272786630106,253.9,27.0647672615988)) ;
#103453=CARTESIAN_POINT('',(38.084204758092,253.9,26.233971611495)) ;
#103454=CARTESIAN_POINT('',(35.6120145486888,253.75,26.8795155697285)) ;
#103455=CARTESIAN_POINT('',(38.0378522089358,253.75,26.0913131340507)) ;
#103456=CARTESIAN_POINT('Ctrl Pts',(35.6120145486888,253.75,26.8795155697285)) ;
#103457=CARTESIAN_POINT('Ctrl Pts',(35.611681519077,253.75,26.8802305456133)) ;
#103458=CARTESIAN_POINT('Ctrl Pts',(35.6113485453403,253.750003330106,26.8809455537216)) ;
#103459=CARTESIAN_POINT('Ctrl Pts',(35.6024366389788,253.750181671152,26.9000865264633)) ;
#103460=CARTESIAN_POINT('Ctrl Pts',(35.5938647671061,253.752566842488,26.9186005211265)) ;
#103461=CARTESIAN_POINT('Ctrl Pts',(35.5776823313821,253.761740190968,26.9537361257337)) ;
#103462=CARTESIAN_POINT('Ctrl Pts',(35.5699747087622,253.768377217198,26.9705605654438)) ;
#103463=CARTESIAN_POINT('Ctrl Pts',(35.554898435909,253.78721321578,27.0036148517979)) ;
#103464=CARTESIAN_POINT('Ctrl Pts',(35.5475916277511,253.800023548159,27.0197271316055)) ;
#103465=CARTESIAN_POINT('Ctrl Pts',(35.5370091274324,253.828041657271,27.0431407641495)) ;
#103466=CARTESIAN_POINT('Ctrl Pts',(35.5332364694245,253.841958224525,27.0515181361211)) ;
#103467=CARTESIAN_POINT('Ctrl Pts',(35.5284685425009,253.870954690135,27.0621166715429)) ;
#103468=CARTESIAN_POINT('Ctrl Pts',(35.5272786630106,253.885320776746,27.0647672615988)) ;
#103469=CARTESIAN_POINT('Ctrl Pts',(35.5272786630106,253.9,27.0647672615988)) ;
#103470=CARTESIAN_POINT('Origin',(40.2,253.9,25.0213203435596)) ;
#103471=CARTESIAN_POINT('',(35.8002600262484,253.9,27.6005233528965)) ;
#103472=CARTESIAN_POINT('Origin',(40.2,253.9,25.0213203435596)) ;
#103473=CARTESIAN_POINT('',(35.9999382971499,253.75,27.6408587937931)) ;
#103474=CARTESIAN_POINT('Origin',(40.2,253.75,25.0213203435596)) ;
#103475=CARTESIAN_POINT('Ctrl Pts',(35.9999382971499,253.75,27.6408587937931)) ;
#103476=CARTESIAN_POINT('Ctrl Pts',(35.999164119612,253.75,27.6407079681274)) ;
#103477=CARTESIAN_POINT('Ctrl Pts',(35.9983899488536,253.750003330105,27.6405570783186)) ;
#103478=CARTESIAN_POINT('Ctrl Pts',(35.9776662894844,253.750181671152,27.6365161805243)) ;
#103479=CARTESIAN_POINT('Ctrl Pts',(35.9576497332976,253.752566842488,27.6325687175194)) ;
#103480=CARTESIAN_POINT('Ctrl Pts',(35.9197126349983,253.761740190968,27.6250083928119)) ;
#103481=CARTESIAN_POINT('Ctrl Pts',(35.9015709504458,253.768377217198,27.621354832958)) ;
#103482=CARTESIAN_POINT('Ctrl Pts',(35.8659678602057,253.78721321578,27.6141229718641)) ;
#103483=CARTESIAN_POINT('Ctrl Pts',(35.8486379179467,253.800023548159,27.6105637433868)) ;
#103484=CARTESIAN_POINT('Ctrl Pts',(35.823475653699,253.828041657271,27.6053629780756)) ;
#103485=CARTESIAN_POINT('Ctrl Pts',(35.8144807046667,253.841958224525,27.6034910268201)) ;
#103486=CARTESIAN_POINT('Ctrl Pts',(35.8031037922653,253.870954690135,27.6011186979124)) ;
#103487=CARTESIAN_POINT('Ctrl Pts',(35.8002600262485,253.885320776746,27.6005233528965)) ;
#103488=CARTESIAN_POINT('Ctrl Pts',(35.8002600262485,253.9,27.6005233528965)) ;
#103489=CARTESIAN_POINT('Origin',(37.7789755671721,253.9,26.3483125582154)) ;
#103490=CARTESIAN_POINT('',(35.4752044197332,253.9,27.8366900749965)) ;
#103491=CARTESIAN_POINT('',(37.6908077793282,253.9,26.2269600090591)) ;
#103492=CARTESIAN_POINT('',(35.5603672117706,253.75,27.9602258814026)) ;
#103493=CARTESIAN_POINT('',(37.7789755671721,253.75,26.3483125582154)) ;
#103494=CARTESIAN_POINT('Ctrl Pts',(35.5603672117706,253.75,27.9602258814026)) ;
#103495=CARTESIAN_POINT('Ctrl Pts',(35.5595422127747,253.75,27.9590229387353)) ;
#103496=CARTESIAN_POINT('Ctrl Pts',(35.5587171553567,253.750021261236,27.957820129938)) ;
#103497=CARTESIAN_POINT('Ctrl Pts',(35.5578923045725,253.750063777237,27.9566178371378)) ;
#103498=CARTESIAN_POINT('Ctrl Pts',(35.5472956800808,253.750609968276,27.9411723219294)) ;
#103499=CARTESIAN_POINT('Ctrl Pts',(35.5368331274772,253.754658837467,27.92595826731)) ;
#103500=CARTESIAN_POINT('Ctrl Pts',(35.527053294334,253.762001431812,27.9117600448446)) ;
#103501=CARTESIAN_POINT('Ctrl Pts',(35.5168578301213,253.769656077527,27.8969584151122)) ;
#103502=CARTESIAN_POINT('Ctrl Pts',(35.5075954635632,253.78074710398,27.8835376386856)) ;
#103503=CARTESIAN_POINT('Ctrl Pts',(35.499796184335,253.794651469056,27.8722475987309)) ;
#103504=CARTESIAN_POINT('Ctrl Pts',(35.4919989918665,253.808552113907,27.860960579517)) ;
#103505=CARTESIAN_POINT('Ctrl Pts',(35.4858134917465,253.824998688613,27.8520189483947)) ;
#103506=CARTESIAN_POINT('Ctrl Pts',(35.4815944923177,253.843066458683,27.8459219612512)) ;
#103507=CARTESIAN_POINT('Ctrl Pts',(35.4773760127934,253.861132002274,27.8398257254355)) ;
#103508=CARTESIAN_POINT('Ctrl Pts',(35.4752044197331,253.880472526098,27.8366900749965)) ;
#103509=CARTESIAN_POINT('Ctrl Pts',(35.4752044197332,253.9,27.8366900749965)) ;
#103510=CARTESIAN_POINT('Origin',(35.7504065309378,253.9,28.2541392311682)) ;
#103511=CARTESIAN_POINT('',(36.0623821418868,253.9,28.6448708758722)) ;
#103512=CARTESIAN_POINT('Origin',(35.7504065309378,253.9,28.2541392311682)) ;
#103513=CARTESIAN_POINT('',(35.9712093582363,253.75,28.5257015839659)) ;
#103514=CARTESIAN_POINT('Origin',(35.7504065309378,253.75,28.2541392311682)) ;
#103515=CARTESIAN_POINT('Ctrl Pts',(35.9712093582364,253.75,28.5257015839658)) ;
#103516=CARTESIAN_POINT('Ctrl Pts',(35.9720984859886,253.75,28.5268579343639)) ;
#103517=CARTESIAN_POINT('Ctrl Pts',(35.9729874683689,253.750021261236,28.5280142989583)) ;
#103518=CARTESIAN_POINT('Ctrl Pts',(35.9738760238612,253.750063777237,28.5291703075783)) ;
#103519=CARTESIAN_POINT('Ctrl Pts',(35.9852910447033,253.750609968276,28.5440212230314)) ;
#103520=CARTESIAN_POINT('Ctrl Pts',(35.9965273639227,253.754658837467,28.5586731032995)) ;
#103521=CARTESIAN_POINT('Ctrl Pts',(36.0070085412753,253.762001431812,28.5723617693703)) ;
#103522=CARTESIAN_POINT('Ctrl Pts',(36.017935155977,253.769656077527,28.5866321871779)) ;
#103523=CARTESIAN_POINT('Ctrl Pts',(36.0278368441769,253.78074710398,28.5995884692427)) ;
#103524=CARTESIAN_POINT('Ctrl Pts',(36.0361642004197,253.794651469056,28.6104948387884)) ;
#103525=CARTESIAN_POINT('Ctrl Pts',(36.0444893286114,253.808552113907,28.6213982902473)) ;
#103526=CARTESIAN_POINT('Ctrl Pts',(36.0510819005004,253.824998688613,28.6300441664174)) ;
#103527=CARTESIAN_POINT('Ctrl Pts',(36.0555767373301,253.843066458683,28.6359407459584)) ;
#103528=CARTESIAN_POINT('Ctrl Pts',(36.0600710202639,253.861132002274,28.6418365988678)) ;
#103529=CARTESIAN_POINT('Ctrl Pts',(36.0623821418869,253.880472526098,28.6448708758721)) ;
#103530=CARTESIAN_POINT('Ctrl Pts',(36.0623821418868,253.9,28.6448708758721)) ;
#103531=CARTESIAN_POINT('Origin',(38.4743212102356,253.9,26.7070843711341)) ;
#103532=CARTESIAN_POINT('',(36.387437748402,253.9,28.4087041537722)) ;
#103533=CARTESIAN_POINT('',(38.5624889980795,253.9,26.8284369202904)) ;
#103534=CARTESIAN_POINT('',(36.4107804436157,253.75,28.2063344963562)) ;
#103535=CARTESIAN_POINT('',(38.4743212102356,253.75,26.7070843711341)) ;
#103536=CARTESIAN_POINT('Ctrl Pts',(36.4107804436157,253.75,28.2063344963562)) ;
#103537=CARTESIAN_POINT('Ctrl Pts',(36.4106846533323,253.75,28.2071173906402)) ;
#103538=CARTESIAN_POINT('Ctrl Pts',(36.4105889261468,253.750003330106,28.2079002983041)) ;
#103539=CARTESIAN_POINT('Ctrl Pts',(36.408028085395,253.750181671152,28.228858375676)) ;
#103540=CARTESIAN_POINT('Ctrl Pts',(36.4055968897784,253.752566842488,28.2491150850256)) ;
#103541=CARTESIAN_POINT('Ctrl Pts',(36.4010639777649,253.761740190968,28.2875316783901)) ;
#103542=CARTESIAN_POINT('Ctrl Pts',(36.3989326308384,253.768377217198,28.3059144577853)) ;
#103543=CARTESIAN_POINT('Ctrl Pts',(36.3948085795202,253.78721321578,28.3420097767375)) ;
#103544=CARTESIAN_POINT('Ctrl Pts',(36.3928383602869,253.800023548159,28.3595913933363)) ;
#103545=CARTESIAN_POINT('Ctrl Pts',(36.3900090147564,253.828041657271,28.3851292535788)) ;
#103546=CARTESIAN_POINT('Ctrl Pts',(36.3890097540816,253.841958224525,28.3942624232202)) ;
#103547=CARTESIAN_POINT('Ctrl Pts',(36.3877503136725,253.870954690135,28.4058155998437)) ;
#103548=CARTESIAN_POINT('Ctrl Pts',(36.387437748402,253.885320776746,28.4087041537722)) ;
#103549=CARTESIAN_POINT('Ctrl Pts',(36.387437748402,253.9,28.4087041537722)) ;
#103550=CARTESIAN_POINT('Origin',(40.2,253.9,25.0213203435596)) ;
#103551=CARTESIAN_POINT('',(36.8126161897874,253.9,28.8338825951576)) ;
#103552=CARTESIAN_POINT('Origin',(40.2,253.9,25.0213203435596)) ;
#103553=CARTESIAN_POINT('',(37.0149858472034,253.75,28.8105398999439)) ;
#103554=CARTESIAN_POINT('Origin',(40.2,253.75,25.0213203435596)) ;
#103555=CARTESIAN_POINT('Ctrl Pts',(37.0149858472034,253.75,28.8105398999439)) ;
#103556=CARTESIAN_POINT('Ctrl Pts',(37.0142029529195,253.75,28.8106356902274)) ;
#103557=CARTESIAN_POINT('Ctrl Pts',(37.0134200452556,253.750003330106,28.8107314174129)) ;
#103558=CARTESIAN_POINT('Ctrl Pts',(36.9924619678827,253.750181671152,28.8132922581644)) ;
#103559=CARTESIAN_POINT('Ctrl Pts',(36.9722052585338,253.752566842488,28.8157234537813)) ;
#103560=CARTESIAN_POINT('Ctrl Pts',(36.9337886651694,253.761740190968,28.8202563657947)) ;
#103561=CARTESIAN_POINT('Ctrl Pts',(36.9154058857743,253.768377217198,28.8223877127213)) ;
#103562=CARTESIAN_POINT('Ctrl Pts',(36.8793105668222,253.78721321578,28.8265117640394)) ;
#103563=CARTESIAN_POINT('Ctrl Pts',(36.8617289502234,253.800023548159,28.8284819832727)) ;
#103564=CARTESIAN_POINT('Ctrl Pts',(36.8361910899809,253.828041657271,28.8313113288033)) ;
#103565=CARTESIAN_POINT('Ctrl Pts',(36.8270579203394,253.841958224525,28.832310589478)) ;
#103566=CARTESIAN_POINT('Ctrl Pts',(36.815504743716,253.870954690135,28.8335700298872)) ;
#103567=CARTESIAN_POINT('Ctrl Pts',(36.8126161897874,253.885320776746,28.8338825951576)) ;
#103568=CARTESIAN_POINT('Ctrl Pts',(36.8126161897874,253.9,28.8338825951576)) ;
#103569=CARTESIAN_POINT('Origin',(38.3075320827811,253.9,27.0315026299217)) ;
#103570=CARTESIAN_POINT('',(36.5764494676875,253.9,29.1589382016729)) ;
#103571=CARTESIAN_POINT('',(38.1861795336248,253.9,26.9433348420779)) ;
#103572=CARTESIAN_POINT('',(36.6956187595936,253.75,29.2501109853235)) ;
#103573=CARTESIAN_POINT('',(38.3075320827811,253.75,27.0315026299217)) ;
#103574=CARTESIAN_POINT('Ctrl Pts',(36.6956187595936,253.75,29.2501109853235)) ;
#103575=CARTESIAN_POINT('Ctrl Pts',(36.6944624091953,253.75,29.2492218575712)) ;
#103576=CARTESIAN_POINT('Ctrl Pts',(36.693306044602,253.750021261236,29.2483328751903)) ;
#103577=CARTESIAN_POINT('Ctrl Pts',(36.6921500359814,253.750063777237,29.2474443196982)) ;
#103578=CARTESIAN_POINT('Ctrl Pts',(36.6772991205231,253.750609968276,29.2360292988605)) ;
#103579=CARTESIAN_POINT('Ctrl Pts',(36.6626472402606,253.754658837467,29.2247929796359)) ;
#103580=CARTESIAN_POINT('Ctrl Pts',(36.6489585741898,253.762001431812,29.2143118022838)) ;
#103581=CARTESIAN_POINT('Ctrl Pts',(36.6346881563818,253.769656077527,29.2033851875823)) ;
#103582=CARTESIAN_POINT('Ctrl Pts',(36.6217318743171,253.78074710398,29.1934834993824)) ;
#103583=CARTESIAN_POINT('Ctrl Pts',(36.6108255047715,253.794651469056,29.1851561431397)) ;
#103584=CARTESIAN_POINT('Ctrl Pts',(36.5999220533126,253.808552113907,29.176831014948)) ;
#103585=CARTESIAN_POINT('Ctrl Pts',(36.5912761771423,253.824998688613,29.1702384430592)) ;
#103586=CARTESIAN_POINT('Ctrl Pts',(36.5853795976013,253.843066458683,29.1657436062294)) ;
#103587=CARTESIAN_POINT('Ctrl Pts',(36.579483744692,253.861132002274,29.1612493232954)) ;
#103588=CARTESIAN_POINT('Ctrl Pts',(36.5764494676874,253.880472526098,29.1589382016731)) ;
#103589=CARTESIAN_POINT('Ctrl Pts',(36.5764494676874,253.9,29.158938201673)) ;
#103590=CARTESIAN_POINT('Origin',(36.9671811123914,253.9,29.4709138126218)) ;
#103591=CARTESIAN_POINT('',(37.3846302685632,253.9,29.7461159238265)) ;
#103592=CARTESIAN_POINT('Origin',(36.9671811123914,253.9,29.4709138126218)) ;
#103593=CARTESIAN_POINT('',(37.2610944621571,253.75,29.6609531317891)) ;
#103594=CARTESIAN_POINT('Origin',(36.9671811123914,253.75,29.4709138126218)) ;
#103595=CARTESIAN_POINT('Ctrl Pts',(37.2610944621618,253.75,29.6609531317925)) ;
#103596=CARTESIAN_POINT('Ctrl Pts',(37.2622974048275,253.75,29.6617781307873)) ;
#103597=CARTESIAN_POINT('Ctrl Pts',(37.2635002136233,253.750021261236,29.6626031882038)) ;
#103598=CARTESIAN_POINT('Ctrl Pts',(37.2647025064218,253.750063777237,29.663428038987)) ;
#103599=CARTESIAN_POINT('Ctrl Pts',(37.2801480216301,253.750609968276,29.6740246634796)) ;
#103600=CARTESIAN_POINT('Ctrl Pts',(37.2953620762498,253.754658837467,29.6844872160823)) ;
#103601=CARTESIAN_POINT('Ctrl Pts',(37.3095602987151,253.762001431812,29.6942670492256)) ;
#103602=CARTESIAN_POINT('Ctrl Pts',(37.3243619284475,253.769656077527,29.7044625134383)) ;
#103603=CARTESIAN_POINT('Ctrl Pts',(37.337782704874,253.78074710398,29.7137248799965)) ;
#103604=CARTESIAN_POINT('Ctrl Pts',(37.3490727448287,253.794651469056,29.7215241592247)) ;
#103605=CARTESIAN_POINT('Ctrl Pts',(37.3603597640426,253.808552113907,29.7293213516932)) ;
#103606=CARTESIAN_POINT('Ctrl Pts',(37.3693013951648,253.824998688613,29.7355068518133)) ;
#103607=CARTESIAN_POINT('Ctrl Pts',(37.3753983823083,253.843066458683,29.7397258512422)) ;
#103608=CARTESIAN_POINT('Ctrl Pts',(37.3814946181241,253.861132002274,29.7439443307665)) ;
#103609=CARTESIAN_POINT('Ctrl Pts',(37.3846302685631,253.880472526098,29.7461159238265)) ;
#103610=CARTESIAN_POINT('Ctrl Pts',(37.3846302685632,253.9,29.7461159238264)) ;
#103611=CARTESIAN_POINT('Origin',(39.0797116749887,253.9,27.1578412797899)) ;
#103612=CARTESIAN_POINT('',(39.201064224145,253.9,27.2460090676338)) ;
#103613=CARTESIAN_POINT('',(39.0797116749887,253.75,27.1578412797899)) ;
#103614=CARTESIAN_POINT('Origin',(42.3676071114944,258.25,19.9664732232009)) ;
#103615=CARTESIAN_POINT('',(42.3676071114944,258.1,19.9664732232009)) ;
#103616=CARTESIAN_POINT('',(42.3676071114944,258.25,19.9664732232009)) ;
#103617=CARTESIAN_POINT('',(42.2434469180392,258.1,20.3485990065702)) ;
#103618=CARTESIAN_POINT('',(41.5213219337175,258.1,22.5710711826001)) ;
#103619=CARTESIAN_POINT('',(42.2434469180392,258.25,20.3485990065702)) ;
#103620=CARTESIAN_POINT('Origin',(41.8995934690622,258.25,19.7905095039363)) ;
#103621=CARTESIAN_POINT('',(41.4175335996131,258.1,19.6577756263215)) ;
#103622=CARTESIAN_POINT('',(41.4175335996131,258.25,19.6577756263215)) ;
#103623=CARTESIAN_POINT('Origin',(41.8995934690622,258.1,19.7905095039363)) ;
#103624=CARTESIAN_POINT('Origin',(41.2001922680488,258.25,20.3266834644245)) ;
#103625=CARTESIAN_POINT('',(41.2933734061579,258.1,20.0399014096908)) ;
#103626=CARTESIAN_POINT('',(41.2933734061579,258.25,20.0399014096908)) ;
#103627=CARTESIAN_POINT('',(40.4625777560541,258.1,22.5968275047722)) ;
#103628=CARTESIAN_POINT('Origin',(40.2,258.25,25.0213203435596)) ;
#103629=CARTESIAN_POINT('',(40.6994832039963,258.1,19.9458384424072)) ;
#103630=CARTESIAN_POINT('',(40.6994832039963,258.25,19.9458384424072)) ;
#103631=CARTESIAN_POINT('Origin',(40.2,258.1,25.0213203435596)) ;
#103632=CARTESIAN_POINT('Origin',(40.6994832039963,258.25,19.5440476162869)) ;
#103633=CARTESIAN_POINT('',(40.6994832039963,258.1,19.5440476162869)) ;
#103634=CARTESIAN_POINT('',(40.6994832039963,258.25,19.5440476162869)) ;
#103635=CARTESIAN_POINT('',(40.6994832039963,258.1,22.2826839799233)) ;
#103636=CARTESIAN_POINT('Origin',(40.2,258.25,19.5213203435596)) ;
#103637=CARTESIAN_POINT('',(39.7005167960037,258.1,19.5440476162869)) ;
#103638=CARTESIAN_POINT('',(39.7005167960037,258.25,19.5440476162869)) ;
#103639=CARTESIAN_POINT('Origin',(40.2,258.1,19.5213203435596)) ;
#103640=CARTESIAN_POINT('Origin',(39.7005167960037,258.25,20.2473789395491)) ;
#103641=CARTESIAN_POINT('',(39.7005167960037,258.1,19.9458384424072)) ;
#103642=CARTESIAN_POINT('',(39.7005167960037,258.25,19.9458384424072)) ;
#103643=CARTESIAN_POINT('',(39.7005167960037,258.1,22.6343496415544)) ;
#103644=CARTESIAN_POINT('Origin',(40.2,258.25,25.0213203435596)) ;
#103645=CARTESIAN_POINT('',(39.1066265938421,258.1,20.0399014096908)) ;
#103646=CARTESIAN_POINT('',(39.1066265938421,258.25,20.0399014096908)) ;
#103647=CARTESIAN_POINT('Origin',(40.2,258.1,25.0213203435596)) ;
#103648=CARTESIAN_POINT('Origin',(38.982466400387,258.25,19.6577756263215)) ;
#103649=CARTESIAN_POINT('',(38.982466400387,258.1,19.6577756263215)) ;
#103650=CARTESIAN_POINT('',(38.982466400387,258.25,19.6577756263215)) ;
#103651=CARTESIAN_POINT('',(39.8287515781638,258.1,22.2623735857207)) ;
#103652=CARTESIAN_POINT('Origin',(38.5004065309378,258.25,19.7905095039363)) ;
#103653=CARTESIAN_POINT('',(38.0323928885057,258.1,19.9664732232009)) ;
#103654=CARTESIAN_POINT('',(38.0323928885057,258.25,19.9664732232009)) ;
#103655=CARTESIAN_POINT('Origin',(38.5004065309378,258.1,19.7905095039363)) ;
#103656=CARTESIAN_POINT('Origin',(38.2497342200699,258.25,20.6353810613039)) ;
#103657=CARTESIAN_POINT('',(38.1565530819608,258.1,20.3485990065702)) ;
#103658=CARTESIAN_POINT('',(38.1565530819608,258.25,20.3485990065702)) ;
#103659=CARTESIAN_POINT('',(38.9873487320647,258.1,22.9055251016516)) ;
#103660=CARTESIAN_POINT('Origin',(40.2,258.25,25.0213203435596)) ;
#103661=CARTESIAN_POINT('',(37.6207969906631,258.1,20.6215803698081)) ;
#103662=CARTESIAN_POINT('',(37.6207969906631,258.25,20.6215803698081)) ;
#103663=CARTESIAN_POINT('Origin',(40.2,258.1,25.0213203435596)) ;
#103664=CARTESIAN_POINT('Origin',(37.3846302685632,258.25,20.2965247632928)) ;
#103665=CARTESIAN_POINT('',(37.3846302685632,258.1,20.2965247632928)) ;
#103666=CARTESIAN_POINT('',(37.3846302685632,258.25,20.2965247632928)) ;
#103667=CARTESIAN_POINT('',(38.9943603345005,258.1,22.5121281228878)) ;
#103668=CARTESIAN_POINT('Origin',(36.9671811123914,258.25,20.5717268744974)) ;
#103669=CARTESIAN_POINT('',(36.5764494676875,258.1,20.8837024854464)) ;
#103670=CARTESIAN_POINT('',(36.5764494676875,258.25,20.8837024854464)) ;
#103671=CARTESIAN_POINT('Origin',(36.9671811123914,258.1,20.5717268744974)) ;
#103672=CARTESIAN_POINT('Origin',(36.9898572469764,258.25,21.4527094786418)) ;
#103673=CARTESIAN_POINT('',(36.8126161897874,258.1,21.2087580919617)) ;
#103674=CARTESIAN_POINT('',(36.8126161897874,258.25,21.2087580919617)) ;
#103675=CARTESIAN_POINT('',(38.3928834232693,258.1,23.3838093416391)) ;
#103676=CARTESIAN_POINT('Origin',(40.2,258.25,25.0213203435596)) ;
#103677=CARTESIAN_POINT('',(36.3874377484021,258.1,21.633936533347)) ;
#103678=CARTESIAN_POINT('',(36.3874377484021,258.25,21.633936533347)) ;
#103679=CARTESIAN_POINT('Origin',(40.2,258.1,25.0213203435596)) ;
#103680=CARTESIAN_POINT('Origin',(36.0623821418868,258.25,21.3977698112471)) ;
#103681=CARTESIAN_POINT('',(36.0623821418868,258.1,21.3977698112471)) ;
#103682=CARTESIAN_POINT('',(36.0623821418868,258.25,21.3977698112471)) ;
#103683=CARTESIAN_POINT('',(38.2779855014818,258.1,23.0074998771845)) ;
#103684=CARTESIAN_POINT('Origin',(35.7504065309378,258.25,21.788501455951)) ;
#103685=CARTESIAN_POINT('',(35.4752044197332,258.1,22.2059506121228)) ;
#103686=CARTESIAN_POINT('',(35.4752044197332,258.25,22.2059506121228)) ;
#103687=CARTESIAN_POINT('Origin',(35.7504065309378,258.1,21.788501455951)) ;
#103688=CARTESIAN_POINT('Origin',(36.0442114129285,258.25,22.6193583914117)) ;
#103689=CARTESIAN_POINT('',(35.8002600262485,258.1,22.4421173342227)) ;
#103690=CARTESIAN_POINT('',(35.8002600262485,258.25,22.4421173342227)) ;
#103691=CARTESIAN_POINT('',(37.9753112759259,258.1,24.0223845677046)) ;
#103692=CARTESIAN_POINT('Origin',(40.2,258.25,25.0213203435596)) ;
#103693=CARTESIAN_POINT('',(35.5272786630106,258.1,22.9778734255204)) ;
#103694=CARTESIAN_POINT('',(35.5272786630106,258.25,22.9778734255204)) ;
#103695=CARTESIAN_POINT('Origin',(40.2,258.1,25.0213203435596)) ;
#103696=CARTESIAN_POINT('Origin',(35.1451528796413,258.25,22.8537132320653)) ;
#103697=CARTESIAN_POINT('',(35.1451528796413,258.1,22.8537132320653)) ;
#103698=CARTESIAN_POINT('',(35.1451528796413,258.25,22.8537132320653)) ;
#103699=CARTESIAN_POINT('',(37.7497508390405,258.1,23.6999984098422)) ;
#103700=CARTESIAN_POINT('Origin',(34.9691891603767,258.25,23.3217268744974)) ;
#103701=CARTESIAN_POINT('',(34.8364552827619,258.1,23.8037867439466)) ;
#103702=CARTESIAN_POINT('',(34.8364552827619,258.25,23.8037867439466)) ;
#103703=CARTESIAN_POINT('Origin',(34.9691891603767,258.1,23.3217268744974)) ;
#103704=CARTESIAN_POINT('Origin',(35.5053631208649,258.25,24.0211280755108)) ;
#103705=CARTESIAN_POINT('',(35.2185810661312,258.1,23.9279469374017)) ;
#103706=CARTESIAN_POINT('',(35.2185810661312,258.25,23.9279469374017)) ;
#103707=CARTESIAN_POINT('',(37.7755071612126,258.1,24.7587425875056)) ;
#103708=CARTESIAN_POINT('Origin',(40.2,258.25,25.0213203435596)) ;
#103709=CARTESIAN_POINT('',(35.1245180988476,258.1,24.5218371395634)) ;
#103710=CARTESIAN_POINT('',(35.1245180988476,258.25,24.5218371395634)) ;
#103711=CARTESIAN_POINT('Origin',(40.2,258.1,25.0213203435596)) ;
#103712=CARTESIAN_POINT('Origin',(34.7227272727273,258.25,24.5218371395634)) ;
#103713=CARTESIAN_POINT('',(34.7227272727273,258.1,24.5218371395634)) ;
#103714=CARTESIAN_POINT('',(34.7227272727273,258.25,24.5218371395634)) ;
#103715=CARTESIAN_POINT('',(37.4613636363637,258.1,24.5218371395634)) ;
#103716=CARTESIAN_POINT('Origin',(34.7,258.25,25.0213203435596)) ;
#103717=CARTESIAN_POINT('',(34.7227272727273,258.1,25.5208035475559)) ;
#103718=CARTESIAN_POINT('',(34.7227272727273,258.25,25.5208035475559)) ;
#103719=CARTESIAN_POINT('Origin',(34.7,258.1,25.0213203435596)) ;
#103720=CARTESIAN_POINT('Origin',(35.4260585959895,258.25,25.5208035475559)) ;
#103721=CARTESIAN_POINT('',(35.1245180988476,258.1,25.5208035475559)) ;
#103722=CARTESIAN_POINT('',(35.1245180988476,258.25,25.5208035475559)) ;
#103723=CARTESIAN_POINT('',(37.8130292979948,258.1,25.5208035475559)) ;
#103724=CARTESIAN_POINT('Origin',(40.2,258.25,25.0213203435596)) ;
#103725=CARTESIAN_POINT('',(35.2185810661312,258.1,26.1146937497175)) ;
#103726=CARTESIAN_POINT('',(35.2185810661312,258.25,26.1146937497175)) ;
#103727=CARTESIAN_POINT('Origin',(40.2,258.1,25.0213203435596)) ;
#103728=CARTESIAN_POINT('Origin',(34.8364552827619,258.25,26.2388539431727)) ;
#103729=CARTESIAN_POINT('',(34.8364552827619,258.1,26.2388539431727)) ;
#103730=CARTESIAN_POINT('',(34.8364552827619,258.25,26.2388539431727)) ;
#103731=CARTESIAN_POINT('',(37.4410532421611,258.1,25.3925687653958)) ;
#103732=CARTESIAN_POINT('Origin',(34.9691891603767,258.25,26.7209138126218)) ;
#103733=CARTESIAN_POINT('',(35.1451528796413,258.1,27.188927455054)) ;
#103734=CARTESIAN_POINT('',(35.1451528796413,258.25,27.188927455054)) ;
#103735=CARTESIAN_POINT('Origin',(34.9691891603767,258.1,26.7209138126218)) ;
#103736=CARTESIAN_POINT('Origin',(35.8140607177443,258.25,26.9715861234897)) ;
#103737=CARTESIAN_POINT('',(35.5272786630106,258.1,27.0647672615988)) ;
#103738=CARTESIAN_POINT('',(35.5272786630106,258.25,27.0647672615988)) ;
#103739=CARTESIAN_POINT('',(38.084204758092,258.1,26.233971611495)) ;
#103740=CARTESIAN_POINT('Origin',(40.2,258.25,25.0213203435596)) ;
#103741=CARTESIAN_POINT('',(35.8002600262484,258.1,27.6005233528965)) ;
#103742=CARTESIAN_POINT('',(35.8002600262484,258.25,27.6005233528965)) ;
#103743=CARTESIAN_POINT('Origin',(40.2,258.1,25.0213203435596)) ;
#103744=CARTESIAN_POINT('Origin',(35.4752044197332,258.25,27.8366900749965)) ;
#103745=CARTESIAN_POINT('',(35.4752044197332,258.1,27.8366900749965)) ;
#103746=CARTESIAN_POINT('',(35.4752044197332,258.25,27.8366900749965)) ;
#103747=CARTESIAN_POINT('',(37.6908077793282,258.1,26.2269600090591)) ;
#103748=CARTESIAN_POINT('Origin',(35.7504065309378,258.25,28.2541392311682)) ;
#103749=CARTESIAN_POINT('',(36.0623821418868,258.1,28.6448708758722)) ;
#103750=CARTESIAN_POINT('',(36.0623821418868,258.25,28.6448708758722)) ;
#103751=CARTESIAN_POINT('Origin',(35.7504065309378,258.1,28.2541392311682)) ;
#103752=CARTESIAN_POINT('Origin',(36.6313891350821,258.25,28.2314630965833)) ;
#103753=CARTESIAN_POINT('',(36.387437748402,258.1,28.4087041537722)) ;
#103754=CARTESIAN_POINT('',(36.387437748402,258.25,28.4087041537722)) ;
#103755=CARTESIAN_POINT('',(38.5624889980795,258.1,26.8284369202904)) ;
#103756=CARTESIAN_POINT('Origin',(40.2,258.25,25.0213203435596)) ;
#103757=CARTESIAN_POINT('',(36.8126161897874,258.1,28.8338825951576)) ;
#103758=CARTESIAN_POINT('',(36.8126161897874,258.25,28.8338825951576)) ;
#103759=CARTESIAN_POINT('Origin',(40.2,258.1,25.0213203435596)) ;
#103760=CARTESIAN_POINT('Origin',(36.5764494676875,258.25,29.1589382016729)) ;
#103761=CARTESIAN_POINT('',(36.5764494676875,258.1,29.1589382016729)) ;
#103762=CARTESIAN_POINT('',(36.5764494676875,258.25,29.1589382016729)) ;
#103763=CARTESIAN_POINT('',(38.1861795336248,258.1,26.9433348420779)) ;
#103764=CARTESIAN_POINT('Origin',(36.9671811123914,258.25,29.4709138126218)) ;
#103765=CARTESIAN_POINT('',(37.3846302685632,258.1,29.7461159238265)) ;
#103766=CARTESIAN_POINT('',(37.3846302685632,258.25,29.7461159238265)) ;
#103767=CARTESIAN_POINT('Origin',(36.9671811123914,258.1,29.4709138126218)) ;
#103768=CARTESIAN_POINT('Origin',(37.7980380478521,258.25,29.1771089306311)) ;
#103769=CARTESIAN_POINT('',(37.6207969906631,258.1,29.4210603173112)) ;
#103770=CARTESIAN_POINT('',(37.6207969906631,258.25,29.4210603173112)) ;
#103771=CARTESIAN_POINT('',(39.201064224145,258.1,27.2460090676338)) ;
#103772=CARTESIAN_POINT('Origin',(40.2,258.25,25.0213203435596)) ;
#103773=CARTESIAN_POINT('',(38.1565530819608,258.1,29.694041680549)) ;
#103774=CARTESIAN_POINT('',(38.1565530819608,258.25,29.694041680549)) ;
#103775=CARTESIAN_POINT('Origin',(40.2,258.1,25.0213203435596)) ;
#103776=CARTESIAN_POINT('Origin',(40.2,253.75,25.0213203435596)) ;
#103777=CARTESIAN_POINT('Origin',(40.2,253.75,25.0213203435596)) ;
#103778=CARTESIAN_POINT('Origin',(40.2,253.75,25.0213203435596)) ;
#103779=CARTESIAN_POINT('Origin',(40.2,253.75,25.0213203435596)) ;
#103780=CARTESIAN_POINT('Origin',(40.2,253.75,25.0213203435596)) ;
#103781=CARTESIAN_POINT('Origin',(40.2,253.75,25.0213203435596)) ;
#103782=CARTESIAN_POINT('Origin',(40.2,253.75,25.0213203435596)) ;
#103783=CARTESIAN_POINT('Origin',(40.2,253.75,25.0213203435596)) ;
#103784=CARTESIAN_POINT('Origin',(40.2,253.75,25.0213203435596)) ;
#103785=CARTESIAN_POINT('Origin',(40.2,253.75,25.0213203435596)) ;
#103786=CARTESIAN_POINT('Origin',(40.2,253.75,25.0213203435596)) ;
#103787=CARTESIAN_POINT('Origin',(40.2,253.75,25.0213203435596)) ;
#103788=CARTESIAN_POINT('Origin',(40.2,253.75,25.0213203435596)) ;
#103789=CARTESIAN_POINT('Origin',(40.2,253.75,25.0213203435596)) ;
#103790=CARTESIAN_POINT('Origin',(40.2,253.75,25.0213203435596)) ;
#103791=CARTESIAN_POINT('Origin',(40.2,253.75,25.0213203435596)) ;
#103792=CARTESIAN_POINT('Origin',(40.2,253.75,25.0213203435596)) ;
#103793=CARTESIAN_POINT('Origin',(40.2,253.75,25.0213203435596)) ;
#103794=CARTESIAN_POINT('Origin',(40.2,253.75,25.0213203435596)) ;
#103795=CARTESIAN_POINT('Origin',(40.2,253.75,25.0213203435596)) ;
#103796=CARTESIAN_POINT('Origin',(40.2,253.75,25.0213203435596)) ;
#103797=CARTESIAN_POINT('Origin',(40.2,253.75,25.0213203435596)) ;
#103798=CARTESIAN_POINT('Origin',(40.2,253.75,25.0213203435596)) ;
#103799=CARTESIAN_POINT('Origin',(40.2,253.75,25.0213203435596)) ;
#103800=CARTESIAN_POINT('Origin',(40.2,253.75,25.0213203435596)) ;
#103801=CARTESIAN_POINT('Origin',(40.2,253.75,25.0213203435596)) ;
#103802=CARTESIAN_POINT('Origin',(40.2,253.75,25.0213203435596)) ;
#103803=CARTESIAN_POINT('Origin',(40.2,253.75,25.0213203435596)) ;
#103804=CARTESIAN_POINT('Origin',(40.2,253.75,25.0213203435596)) ;
#103805=CARTESIAN_POINT('Origin',(40.2,253.75,25.0213203435596)) ;
#103806=CARTESIAN_POINT('Origin',(40.2,253.75,25.0213203435596)) ;
#103807=CARTESIAN_POINT('Origin',(40.2,253.75,25.0213203435596)) ;
#103808=CARTESIAN_POINT('Origin',(40.2,253.75,25.0213203435596)) ;
#103809=CARTESIAN_POINT('Origin',(40.2,253.75,25.0213203435596)) ;
#103810=CARTESIAN_POINT('Origin',(40.2,253.75,25.0213203435596)) ;
#103811=CARTESIAN_POINT('Origin',(40.2,253.75,25.0213203435596)) ;
#103812=CARTESIAN_POINT('Origin',(40.2,253.75,25.0213203435596)) ;
#103813=CARTESIAN_POINT('',(40.2,253.75,29.9713203435596)) ;
#103814=CARTESIAN_POINT('Origin',(40.2,253.75,25.0213203435596)) ;
#103815=CARTESIAN_POINT('Origin',(40.2,253.75,25.0213203435596)) ;
#103816=CARTESIAN_POINT('Origin',(40.2,253.6,25.0213203435596)) ;
#103817=CARTESIAN_POINT('Origin',(40.2,253.6,29.9713203435596)) ;
#103818=CARTESIAN_POINT('Origin',(40.2,253.75,25.0213203435596)) ;
#103819=CARTESIAN_POINT('Origin',(40.2,253.75,25.0213203435596)) ;
#103820=CARTESIAN_POINT('Origin',(40.2,258.4,25.0213203435596)) ;
#103821=CARTESIAN_POINT('',(40.2,258.25,20.0713203435596)) ;
#103822=CARTESIAN_POINT('Origin',(40.2,258.4,20.0713203435596)) ;
#103823=CARTESIAN_POINT('',(39.8505167960037,258.25,20.0836729796702)) ;
#103824=CARTESIAN_POINT('Origin',(40.2,258.25,25.0213203435596)) ;
#103825=CARTESIAN_POINT('',(39.0065613308239,258.25,20.2173423936815)) ;
#103826=CARTESIAN_POINT('Origin',(40.2,258.25,25.0213203435596)) ;
#103827=CARTESIAN_POINT('',(38.3418047738312,258.25,20.4333348922484)) ;
#103828=CARTESIAN_POINT('Origin',(40.2,258.25,25.0213203435596)) ;
#103829=CARTESIAN_POINT('',(37.5804615497666,258.25,20.8212586407095)) ;
#103830=CARTESIAN_POINT('Origin',(40.2,258.25,25.0213203435596)) ;
#103831=CARTESIAN_POINT('',(37.0149858472034,258.25,21.2321007871753)) ;
#103832=CARTESIAN_POINT('Origin',(40.2,258.25,25.0213203435596)) ;
#103833=CARTESIAN_POINT('',(36.4107804436157,258.25,21.836306190763)) ;
#103834=CARTESIAN_POINT('Origin',(40.2,258.25,25.0213203435596)) ;
#103835=CARTESIAN_POINT('',(35.9999382971499,258.25,22.4017818933262)) ;
#103836=CARTESIAN_POINT('Origin',(40.2,258.25,25.0213203435596)) ;
#103837=CARTESIAN_POINT('',(35.6120145486888,258.25,23.1631251173908)) ;
#103838=CARTESIAN_POINT('Origin',(40.2,258.25,25.0213203435596)) ;
#103839=CARTESIAN_POINT('',(35.3960220501219,258.25,23.8278816743835)) ;
#103840=CARTESIAN_POINT('Origin',(40.2,258.25,25.0213203435596)) ;
#103841=CARTESIAN_POINT('',(35.2623526361106,258.25,24.6718371395634)) ;
#103842=CARTESIAN_POINT('Origin',(40.2,258.25,25.0213203435596)) ;
#103843=CARTESIAN_POINT('',(35.2623526361106,258.25,25.3708035475559)) ;
#103844=CARTESIAN_POINT('Origin',(40.2,258.25,25.0213203435596)) ;
#103845=CARTESIAN_POINT('',(35.3960220501219,258.25,26.2147590127358)) ;
#103846=CARTESIAN_POINT('Origin',(40.2,258.25,25.0213203435596)) ;
#103847=CARTESIAN_POINT('',(35.6120145486888,258.25,26.8795155697285)) ;
#103848=CARTESIAN_POINT('Origin',(40.2,258.25,25.0213203435596)) ;
#103849=CARTESIAN_POINT('',(35.9999382971499,258.25,27.6408587937931)) ;
#103850=CARTESIAN_POINT('Origin',(40.2,258.25,25.0213203435596)) ;
#103851=CARTESIAN_POINT('',(36.4107804436157,258.25,28.2063344963562)) ;
#103852=CARTESIAN_POINT('Origin',(40.2,258.25,25.0213203435596)) ;
#103853=CARTESIAN_POINT('',(37.0149858472034,258.25,28.8105398999439)) ;
#103854=CARTESIAN_POINT('Origin',(40.2,258.25,25.0213203435596)) ;
#103855=CARTESIAN_POINT('',(37.5804615497666,258.25,29.2213820464098)) ;
#103856=CARTESIAN_POINT('Origin',(40.2,258.25,25.0213203435596)) ;
#103857=CARTESIAN_POINT('',(38.3418047738312,258.25,29.6093057948708)) ;
#103858=CARTESIAN_POINT('Origin',(40.2,258.25,25.0213203435596)) ;
#103859=CARTESIAN_POINT('',(39.0065613308239,258.25,29.8252982934377)) ;
#103860=CARTESIAN_POINT('Origin',(40.2,258.25,25.0213203435596)) ;
#103861=CARTESIAN_POINT('',(39.8505167960038,258.25,29.9589677074491)) ;
#103862=CARTESIAN_POINT('Origin',(40.2,258.25,25.0213203435596)) ;
#103863=CARTESIAN_POINT('',(40.5494832039963,258.25,29.9589677074491)) ;
#103864=CARTESIAN_POINT('Origin',(40.2,258.25,25.0213203435596)) ;
#103865=CARTESIAN_POINT('',(41.3934386691762,258.25,29.8252982934377)) ;
#103866=CARTESIAN_POINT('Origin',(40.2,258.25,25.0213203435596)) ;
#103867=CARTESIAN_POINT('',(42.0581952261689,258.25,29.6093057948708)) ;
#103868=CARTESIAN_POINT('Origin',(40.2,258.25,25.0213203435596)) ;
#103869=CARTESIAN_POINT('',(42.8195384502335,258.25,29.2213820464098)) ;
#103870=CARTESIAN_POINT('Origin',(40.2,258.25,25.0213203435596)) ;
#103871=CARTESIAN_POINT('',(43.3850141527966,258.25,28.8105398999439)) ;
#103872=CARTESIAN_POINT('Origin',(40.2,258.25,25.0213203435596)) ;
#103873=CARTESIAN_POINT('',(43.9892195563843,258.25,28.2063344963563)) ;
#103874=CARTESIAN_POINT('Origin',(40.2,258.25,25.0213203435596)) ;
#103875=CARTESIAN_POINT('',(44.4000617028502,258.25,27.6408587937931)) ;
#103876=CARTESIAN_POINT('Origin',(40.2,258.25,25.0213203435596)) ;
#103877=CARTESIAN_POINT('',(44.7879854513112,258.25,26.8795155697285)) ;
#103878=CARTESIAN_POINT('Origin',(40.2,258.25,25.0213203435596)) ;
#103879=CARTESIAN_POINT('',(45.0039779498781,258.25,26.2147590127358)) ;
#103880=CARTESIAN_POINT('Origin',(40.2,258.25,25.0213203435596)) ;
#103881=CARTESIAN_POINT('',(45.1376473638895,258.25,25.3708035475559)) ;
#103882=CARTESIAN_POINT('Origin',(40.2,258.25,25.0213203435596)) ;
#103883=CARTESIAN_POINT('',(45.1376473638895,258.25,24.6718371395634)) ;
#103884=CARTESIAN_POINT('Origin',(40.2,258.25,25.0213203435596)) ;
#103885=CARTESIAN_POINT('',(45.0039779498781,258.25,23.8278816743835)) ;
#103886=CARTESIAN_POINT('Origin',(40.2,258.25,25.0213203435596)) ;
#103887=CARTESIAN_POINT('',(44.7879854513112,258.25,23.1631251173908)) ;
#103888=CARTESIAN_POINT('Origin',(40.2,258.25,25.0213203435596)) ;
#103889=CARTESIAN_POINT('',(44.4000617028502,258.25,22.4017818933262)) ;
#103890=CARTESIAN_POINT('Origin',(40.2,258.25,25.0213203435596)) ;
#103891=CARTESIAN_POINT('',(43.9892195563843,258.25,21.836306190763)) ;
#103892=CARTESIAN_POINT('Origin',(40.2,258.25,25.0213203435596)) ;
#103893=CARTESIAN_POINT('',(43.3850141527966,258.25,21.2321007871753)) ;
#103894=CARTESIAN_POINT('Origin',(40.2,258.25,25.0213203435596)) ;
#103895=CARTESIAN_POINT('',(42.8195384502335,258.25,20.8212586407095)) ;
#103896=CARTESIAN_POINT('Origin',(40.2,258.25,25.0213203435596)) ;
#103897=CARTESIAN_POINT('',(42.0581952261685,258.25,20.4333348922483)) ;
#103898=CARTESIAN_POINT('Origin',(40.2,258.25,25.0213203435596)) ;
#103899=CARTESIAN_POINT('',(41.3934386691762,258.25,20.2173423936815)) ;
#103900=CARTESIAN_POINT('Origin',(40.2,258.25,25.0213203435596)) ;
#103901=CARTESIAN_POINT('',(40.5494832039963,258.25,20.0836729796702)) ;
#103902=CARTESIAN_POINT('Origin',(40.2,258.25,25.0213203435596)) ;
#103903=CARTESIAN_POINT('Origin',(40.2,258.25,25.0213203435596)) ;
#103904=CARTESIAN_POINT('Origin',(40.2,258.25,25.0213203435596)) ;
#103905=CARTESIAN_POINT('',(42.2260964403124,258.25,19.9165880896072)) ;
#103906=CARTESIAN_POINT('',(41.3786634562732,258.25,22.5247186334439)) ;
#103907=CARTESIAN_POINT('',(41.5613398833194,258.25,19.700595591041)) ;
#103908=CARTESIAN_POINT('Origin',(41.8995934690622,258.25,19.7905095039363)) ;
#103909=CARTESIAN_POINT('',(40.6052362334984,258.25,22.6431800539285)) ;
#103910=CARTESIAN_POINT('Origin',(40.2,258.25,25.0213203435596)) ;
#103911=CARTESIAN_POINT('',(43.7043812404059,258.25,20.7925297017964)) ;
#103912=CARTESIAN_POINT('',(42.0924679172189,258.25,23.0111380571975)) ;
#103913=CARTESIAN_POINT('',(43.1389055378432,258.25,20.3816875553299)) ;
#103914=CARTESIAN_POINT('Origin',(43.4328188876086,258.25,20.5717268744974)) ;
#103915=CARTESIAN_POINT('',(41.3202883250113,258.25,22.8847994073294)) ;
#103916=CARTESIAN_POINT('Origin',(40.2,258.25,25.0213203435596)) ;
#103917=CARTESIAN_POINT('',(44.8396327882295,258.25,22.0824148057166)) ;
#103918=CARTESIAN_POINT('',(42.621024432828,258.25,23.6943281289039)) ;
#103919=CARTESIAN_POINT('',(44.428790641764,258.25,21.5169391031532)) ;
#103920=CARTESIAN_POINT('Origin',(44.6495934690622,258.25,21.788501455951)) ;
#103921=CARTESIAN_POINT('',(41.9256787897644,258.25,23.3355563159851)) ;
#103922=CARTESIAN_POINT('Origin',(40.2,258.25,25.0213203435596)) ;
#103923=CARTESIAN_POINT('',(45.5207247525196,258.25,23.6599804602399)) ;
#103924=CARTESIAN_POINT('',(42.9125942086827,258.25,24.5074134442792)) ;
#103925=CARTESIAN_POINT('',(45.3047322539521,258.25,22.9952239032473)) ;
#103926=CARTESIAN_POINT('Origin',(45.4308108396234,258.25,23.3217268744974)) ;
#103927=CARTESIAN_POINT('',(42.3621477910643,258.25,23.9513275530686)) ;
#103928=CARTESIAN_POINT('Origin',(40.2,258.25,25.0213203435596)) ;
#103929=CARTESIAN_POINT('',(45.6809871063617,258.25,25.3708035475559)) ;
#103930=CARTESIAN_POINT('',(42.9386363636364,258.25,25.3708035475559)) ;
#103931=CARTESIAN_POINT('',(45.6809871063617,258.25,24.6718371395634)) ;
#103932=CARTESIAN_POINT('Origin',(45.7,258.25,25.0213203435596)) ;
#103933=CARTESIAN_POINT('',(42.5869707020053,258.25,24.6718371395634)) ;
#103934=CARTESIAN_POINT('Origin',(40.2,258.25,25.0213203435596)) ;
#103935=CARTESIAN_POINT('',(45.3047322539528,258.25,27.0474167838721)) ;
#103936=CARTESIAN_POINT('',(42.6966017101158,258.25,26.1999837998328)) ;
#103937=CARTESIAN_POINT('',(45.5207247525189,258.25,26.3826602268791)) ;
#103938=CARTESIAN_POINT('Origin',(45.4308108396234,258.25,26.7209138126218)) ;
#103939=CARTESIAN_POINT('',(42.5781402896312,258.25,25.426556577058)) ;
#103940=CARTESIAN_POINT('Origin',(40.2,258.25,25.0213203435596)) ;
#103941=CARTESIAN_POINT('',(44.4287906417642,258.25,28.5257015839662)) ;
#103942=CARTESIAN_POINT('',(42.2101822863621,258.25,26.9137882607786)) ;
#103943=CARTESIAN_POINT('',(44.8396327882299,258.25,27.9602258814029)) ;
#103944=CARTESIAN_POINT('Origin',(44.6495934690622,258.25,28.2541392311682)) ;
#103945=CARTESIAN_POINT('',(42.3365209362303,258.25,26.1416086685709)) ;
#103946=CARTESIAN_POINT('Origin',(40.2,258.25,25.0213203435596)) ;
#103947=CARTESIAN_POINT('',(43.1389055378432,258.25,29.6609531317894)) ;
#103948=CARTESIAN_POINT('',(41.5269922146558,258.25,27.4423447763876)) ;
#103949=CARTESIAN_POINT('',(43.7043812404062,258.25,29.2501109853232)) ;
#103950=CARTESIAN_POINT('Origin',(43.4328188876086,258.25,29.4709138126218)) ;
#103951=CARTESIAN_POINT('',(41.8857640275745,258.25,26.746999133324)) ;
#103952=CARTESIAN_POINT('Origin',(40.2,258.25,25.0213203435596)) ;
#103953=CARTESIAN_POINT('',(41.5613398833195,258.25,30.3420450960785)) ;
#103954=CARTESIAN_POINT('',(40.7139068992805,258.25,27.7339145522423)) ;
#103955=CARTESIAN_POINT('',(42.2260964403121,258.25,30.1260525975113)) ;
#103956=CARTESIAN_POINT('Origin',(41.8995934690622,258.25,30.252131183183)) ;
#103957=CARTESIAN_POINT('',(41.2699927904911,258.25,27.1834681346239)) ;
#103958=CARTESIAN_POINT('Origin',(40.2,258.25,25.0213203435596)) ;
#103959=CARTESIAN_POINT('',(39.8505167960037,258.25,30.5023074499212)) ;
#103960=CARTESIAN_POINT('',(39.8505167960037,258.25,27.759956707196)) ;
#103961=CARTESIAN_POINT('',(40.5494832039963,258.25,30.5023074499214)) ;
#103962=CARTESIAN_POINT('Origin',(40.2,258.25,30.5213203435596)) ;
#103963=CARTESIAN_POINT('',(40.5494832039963,258.25,27.4082910455649)) ;
#103964=CARTESIAN_POINT('Origin',(40.2,258.25,25.0213203435596)) ;
#103965=CARTESIAN_POINT('',(38.1739035596877,258.25,30.1260525975118)) ;
#103966=CARTESIAN_POINT('',(39.0213365437268,258.25,27.5179220536754)) ;
#103967=CARTESIAN_POINT('',(38.8386601166806,258.25,30.3420450960783)) ;
#103968=CARTESIAN_POINT('Origin',(38.5004065309378,258.25,30.252131183183)) ;
#103969=CARTESIAN_POINT('',(39.7947637665017,258.25,27.3994606331908)) ;
#103970=CARTESIAN_POINT('Origin',(40.2,258.25,25.0213203435596)) ;
#103971=CARTESIAN_POINT('',(36.6956187595938,258.25,29.2501109853234)) ;
#103972=CARTESIAN_POINT('',(38.3075320827811,258.25,27.0315026299217)) ;
#103973=CARTESIAN_POINT('',(37.2610944621569,258.25,29.6609531317893)) ;
#103974=CARTESIAN_POINT('Origin',(36.9671811123914,258.25,29.4709138126218)) ;
#103975=CARTESIAN_POINT('',(39.0797116749887,258.25,27.1578412797899)) ;
#103976=CARTESIAN_POINT('Origin',(40.2,258.25,25.0213203435596)) ;
#103977=CARTESIAN_POINT('',(35.5603672117705,258.25,27.9602258814026)) ;
#103978=CARTESIAN_POINT('',(37.7789755671721,258.25,26.3483125582154)) ;
#103979=CARTESIAN_POINT('',(35.9712093582364,258.25,28.5257015839658)) ;
#103980=CARTESIAN_POINT('Origin',(35.7504065309378,258.25,28.2541392311682)) ;
#103981=CARTESIAN_POINT('',(38.4743212102356,258.25,26.7070843711341)) ;
#103982=CARTESIAN_POINT('Origin',(40.2,258.25,25.0213203435596)) ;
#103983=CARTESIAN_POINT('',(34.8792752474809,258.25,26.3826602268792)) ;
#103984=CARTESIAN_POINT('',(37.4874057913173,258.25,25.5352272428401)) ;
#103985=CARTESIAN_POINT('',(35.0952677460484,258.25,27.0474167838717)) ;
#103986=CARTESIAN_POINT('Origin',(34.9691891603767,258.25,26.7209138126218)) ;
#103987=CARTESIAN_POINT('',(38.0378522089358,258.25,26.0913131340507)) ;
#103988=CARTESIAN_POINT('Origin',(40.2,258.25,25.0213203435596)) ;
#103989=CARTESIAN_POINT('',(34.7190128936382,258.25,24.6718371395634)) ;
#103990=CARTESIAN_POINT('',(37.4613636363637,258.25,24.6718371395634)) ;
#103991=CARTESIAN_POINT('',(34.7190128936385,258.25,25.3708035475559)) ;
#103992=CARTESIAN_POINT('Origin',(34.7,258.25,25.0213203435596)) ;
#103993=CARTESIAN_POINT('',(37.8130292979948,258.25,25.3708035475559)) ;
#103994=CARTESIAN_POINT('Origin',(40.2,258.25,25.0213203435596)) ;
#103995=CARTESIAN_POINT('',(35.0952677460478,258.25,22.9952239032473)) ;
#103996=CARTESIAN_POINT('',(37.7033982898842,258.25,23.8426568872864)) ;
#103997=CARTESIAN_POINT('',(34.8792752474813,258.25,23.6599804602402)) ;
#103998=CARTESIAN_POINT('Origin',(34.9691891603767,258.25,23.3217268744974)) ;
#103999=CARTESIAN_POINT('',(37.8218597103689,258.25,24.6160841100613)) ;
#104000=CARTESIAN_POINT('Origin',(40.2,258.25,25.0213203435596)) ;
#104001=CARTESIAN_POINT('',(35.9712093582363,258.25,21.5169391031534)) ;
#104002=CARTESIAN_POINT('',(38.1898177136379,258.25,23.1288524263407)) ;
#104003=CARTESIAN_POINT('',(35.5603672117703,258.25,22.0824148057165)) ;
#104004=CARTESIAN_POINT('Origin',(35.7504065309378,258.25,21.788501455951)) ;
#104005=CARTESIAN_POINT('',(38.0634790637697,258.25,23.9010320185483)) ;
#104006=CARTESIAN_POINT('Origin',(40.2,258.25,25.0213203435596)) ;
#104007=CARTESIAN_POINT('',(37.261094462157,258.25,20.3816875553301)) ;
#104008=CARTESIAN_POINT('',(38.8730077853443,258.25,22.6002959107317)) ;
#104009=CARTESIAN_POINT('',(36.6956187595937,258.25,20.7925297017959)) ;
#104010=CARTESIAN_POINT('Origin',(36.9671811123914,258.25,20.5717268744974)) ;
#104011=CARTESIAN_POINT('',(38.5142359724255,258.25,23.2956415537952)) ;
#104012=CARTESIAN_POINT('Origin',(40.2,258.25,25.0213203435596)) ;
#104013=CARTESIAN_POINT('',(38.8386601166805,258.25,19.7005955910407)) ;
#104014=CARTESIAN_POINT('',(39.6860931007195,258.25,22.3087261348769)) ;
#104015=CARTESIAN_POINT('',(38.1739035596879,258.25,19.9165880896081)) ;
#104016=CARTESIAN_POINT('Origin',(38.5004065309378,258.25,19.7905095039363)) ;
#104017=CARTESIAN_POINT('',(39.1300072095089,258.25,22.8591725524954)) ;
#104018=CARTESIAN_POINT('Origin',(40.2,258.25,25.0213203435596)) ;
#104019=CARTESIAN_POINT('',(40.5494832039963,258.25,19.5403332371977)) ;
#104020=CARTESIAN_POINT('',(40.5494832039963,258.25,22.2826839799233)) ;
#104021=CARTESIAN_POINT('',(39.8505167960037,258.25,19.5403332371979)) ;
#104022=CARTESIAN_POINT('Origin',(40.2,258.25,19.5213203435596)) ;
#104023=CARTESIAN_POINT('',(39.8505167960037,258.25,22.6343496415544)) ;
#104024=CARTESIAN_POINT('Origin',(40.2,258.1,25.0213203435596)) ;
#104025=CARTESIAN_POINT('',(39.1066265938421,258.1,30.0027392774284)) ;
#104026=CARTESIAN_POINT('Ctrl Pts',(39.0065613308239,258.25,29.8252982934377)) ;
#104027=CARTESIAN_POINT('Ctrl Pts',(39.0069440085726,258.25,29.8259879723372)) ;
#104028=CARTESIAN_POINT('Ctrl Pts',(39.00732674523,258.249996669895,29.8266776249678)) ;
#104029=CARTESIAN_POINT('Ctrl Pts',(39.0175738303397,258.249818328848,29.8451382901616)) ;
#104030=CARTESIAN_POINT('Ctrl Pts',(39.0275135467839,258.247433157512,29.8629553332033)) ;
#104031=CARTESIAN_POINT('Ctrl Pts',(39.0464270509533,258.238259809031,29.8966993889314)) ;
#104032=CARTESIAN_POINT('Ctrl Pts',(39.0555078816931,258.231622782802,29.9128241441561)) ;
#104033=CARTESIAN_POINT('Ctrl Pts',(39.0733877502474,258.21278678422,29.9444499271496)) ;
#104034=CARTESIAN_POINT('Ctrl Pts',(39.0821280243534,258.199976451841,29.9598318195758)) ;
#104035=CARTESIAN_POINT('Ctrl Pts',(39.0948498133619,258.171958342729,29.9821554300886)) ;
#104036=CARTESIAN_POINT('Ctrl Pts',(39.0994097369161,258.158041775475,29.9901316702287)) ;
#104037=CARTESIAN_POINT('Ctrl Pts',(39.1051816150581,258.129045309865,30.0002186669547)) ;
#104038=CARTESIAN_POINT('Ctrl Pts',(39.1066265938421,258.114679223254,30.0027392774284)) ;
#104039=CARTESIAN_POINT('Ctrl Pts',(39.1066265938421,258.1,30.0027392774284)) ;
#104040=CARTESIAN_POINT('',(39.7005167960037,258.1,30.096802244712)) ;
#104041=CARTESIAN_POINT('Origin',(40.2,258.1,25.0213203435596)) ;
#104042=CARTESIAN_POINT('Ctrl Pts',(39.8505167960038,258.25,29.9589677074491)) ;
#104043=CARTESIAN_POINT('Ctrl Pts',(39.8499397253402,258.25,29.9595053771295)) ;
#104044=CARTESIAN_POINT('Ctrl Pts',(39.849362606764,258.249996669894,29.9600430036272)) ;
#104045=CARTESIAN_POINT('Ctrl Pts',(39.833912390428,258.249818328848,29.9744336161106)) ;
#104046=CARTESIAN_POINT('Ctrl Pts',(39.8189533892428,258.247433157513,29.9883070896971)) ;
#104047=CARTESIAN_POINT('Ctrl Pts',(39.7905380911752,258.238259809032,30.0145549995742)) ;
#104048=CARTESIAN_POINT('Ctrl Pts',(39.7769188845312,258.231622782802,30.0270844220836)) ;
#104049=CARTESIAN_POINT('Ctrl Pts',(39.7501412146258,258.21278678422,30.0516371458428)) ;
#104050=CARTESIAN_POINT('Ctrl Pts',(39.7370754538178,258.199976451841,30.0635653016335)) ;
#104051=CARTESIAN_POINT('Ctrl Pts',(39.7180779384581,258.171958342729,30.0808650678764)) ;
#104052=CARTESIAN_POINT('Ctrl Pts',(39.7112763996935,258.158041775475,30.087041829166)) ;
#104053=CARTESIAN_POINT('Ctrl Pts',(39.7026699639648,258.129045309865,30.0948515246967)) ;
#104054=CARTESIAN_POINT('Ctrl Pts',(39.7005167960037,258.114679223254,30.096802244712)) ;
#104055=CARTESIAN_POINT('Ctrl Pts',(39.7005167960037,258.1,30.096802244712)) ;
#104056=CARTESIAN_POINT('Origin',(39.7947637665017,258.1,27.3994606331908)) ;
#104057=CARTESIAN_POINT('',(38.982466400387,258.1,30.3848650607978)) ;
#104058=CARTESIAN_POINT('Ctrl Pts',(38.8386601166806,258.25,30.3420450960783)) ;
#104059=CARTESIAN_POINT('Ctrl Pts',(38.840059121853,258.25,30.3424579870217)) ;
#104060=CARTESIAN_POINT('Ctrl Pts',(38.8414580177611,258.249978738764,30.3428709748965)) ;
#104061=CARTESIAN_POINT('Ctrl Pts',(38.8428563590733,258.249936222763,30.343283925702)) ;
#104062=CARTESIAN_POINT('Ctrl Pts',(38.860820454012,258.249390031724,30.3485889877858)) ;
#104063=CARTESIAN_POINT('Ctrl Pts',(38.8785229863556,258.245341162533,30.3538380651872)) ;
#104064=CARTESIAN_POINT('Ctrl Pts',(38.8950484329944,258.237998568189,30.3587517471949)) ;
#104065=CARTESIAN_POINT('Ctrl Pts',(38.9122761911102,258.230343922473,30.3638742547396)) ;
#104066=CARTESIAN_POINT('Ctrl Pts',(38.9279023366588,258.21925289602,30.3685360408185)) ;
#104067=CARTESIAN_POINT('Ctrl Pts',(38.9410499125524,258.205348530944,30.3724647819377)) ;
#104068=CARTESIAN_POINT('Ctrl Pts',(38.9541939707065,258.191447886093,30.3763924718908)) ;
#104069=CARTESIAN_POINT('Ctrl Pts',(38.9646093919075,258.175001311387,30.3795121161122)) ;
#104070=CARTESIAN_POINT('Ctrl Pts',(38.9717117137828,258.156933541317,30.3816405503696)) ;
#104071=CARTESIAN_POINT('Ctrl Pts',(38.9788131604437,258.138867997726,30.3837687223414)) ;
#104072=CARTESIAN_POINT('Ctrl Pts',(38.982466400387,258.119527473902,30.3848650607978)) ;
#104073=CARTESIAN_POINT('Ctrl Pts',(38.982466400387,258.1,30.3848650607978)) ;
#104074=CARTESIAN_POINT('',(39.9374222439459,258.1,27.445813182347)) ;
#104075=CARTESIAN_POINT('Origin',(39.8505167960037,258.1,27.759956707196)) ;
#104076=CARTESIAN_POINT('',(39.7005167960037,258.1,30.4985930708324)) ;
#104077=CARTESIAN_POINT('',(39.7005167960037,258.1,27.759956707196)) ;
#104078=CARTESIAN_POINT('Ctrl Pts',(39.7005167960037,258.1,30.4985930708323)) ;
#104079=CARTESIAN_POINT('Ctrl Pts',(39.7005167960037,258.119527473902,30.4985930708323)) ;
#104080=CARTESIAN_POINT('Ctrl Pts',(39.704330020872,258.138867997726,30.4986793042264)) ;
#104081=CARTESIAN_POINT('Ctrl Pts',(39.7117415393001,258.156933541317,30.4988497601077)) ;
#104082=CARTESIAN_POINT('Ctrl Pts',(39.7191539711575,258.175001311387,30.4990202369967)) ;
#104083=CARTESIAN_POINT('Ctrl Pts',(39.7300236484414,258.191447886093,30.4992718211856)) ;
#104084=CARTESIAN_POINT('Ctrl Pts',(39.7437381135435,258.205348530944,30.4995981034065)) ;
#104085=CARTESIAN_POINT('Ctrl Pts',(39.757456249043,258.21925289602,30.4999244729501)) ;
#104086=CARTESIAN_POINT('Ctrl Pts',(39.773758167714,258.230343922473,30.5003195954534)) ;
#104087=CARTESIAN_POINT('Ctrl Pts',(39.7917256812165,258.237998568189,30.5007714713061)) ;
#104088=CARTESIAN_POINT('Ctrl Pts',(39.8089607261725,258.245341162533,30.5012049258647)) ;
#104089=CARTESIAN_POINT('Ctrl Pts',(39.8274188890354,258.249390031724,30.5016831399335)) ;
#104090=CARTESIAN_POINT('Ctrl Pts',(39.8461431129254,258.249936222763,30.5021889366962)) ;
#104091=CARTESIAN_POINT('Ctrl Pts',(39.847600623359,258.249978738764,30.5022283083713)) ;
#104092=CARTESIAN_POINT('Ctrl Pts',(39.8490586727,258.25,30.50226781617)) ;
#104093=CARTESIAN_POINT('Ctrl Pts',(39.8505167960037,258.25,30.5023074499212)) ;
#104094=CARTESIAN_POINT('Origin',(39.0213365437268,258.1,27.5179220536754)) ;
#104095=CARTESIAN_POINT('Ctrl Pts',(38.3418047738311,258.25,29.6093057948708)) ;
#104096=CARTESIAN_POINT('Ctrl Pts',(38.3410897979463,258.25,29.6096388244826)) ;
#104097=CARTESIAN_POINT('Ctrl Pts',(38.3403747898381,258.249996669894,29.6099717982194)) ;
#104098=CARTESIAN_POINT('Ctrl Pts',(38.3212338170961,258.249818328848,29.6188837045809)) ;
#104099=CARTESIAN_POINT('Ctrl Pts',(38.3027198224331,258.247433157512,29.6274555764537)) ;
#104100=CARTESIAN_POINT('Ctrl Pts',(38.267584217826,258.238259809032,29.6436380121775)) ;
#104101=CARTESIAN_POINT('Ctrl Pts',(38.2507597781159,258.231622782802,29.6513456347974)) ;
#104102=CARTESIAN_POINT('Ctrl Pts',(38.2177054917619,258.21278678422,29.6664219076506)) ;
#104103=CARTESIAN_POINT('Ctrl Pts',(38.2015932119542,258.199976451841,29.6737287158086)) ;
#104104=CARTESIAN_POINT('Ctrl Pts',(38.1781795794102,258.171958342729,29.6843112161272)) ;
#104105=CARTESIAN_POINT('Ctrl Pts',(38.1698022074386,258.158041775475,29.6880838741351)) ;
#104106=CARTESIAN_POINT('Ctrl Pts',(38.1592036720168,258.129045309865,29.6928518010587)) ;
#104107=CARTESIAN_POINT('Ctrl Pts',(38.1565530819608,258.114679223254,29.694041680549)) ;
#104108=CARTESIAN_POINT('Ctrl Pts',(38.1565530819608,258.1,29.694041680549)) ;
#104109=CARTESIAN_POINT('',(38.0323928885057,258.1,30.0761674639184)) ;
#104110=CARTESIAN_POINT('',(38.8786780662825,258.1,27.4715695045192)) ;
#104111=CARTESIAN_POINT('Ctrl Pts',(38.0323928885057,258.1,30.0761674639184)) ;
#104112=CARTESIAN_POINT('Ctrl Pts',(38.0323928885057,258.119527473902,30.0761674639184)) ;
#104113=CARTESIAN_POINT('Ctrl Pts',(38.0359928332805,258.138867997726,30.0774278280375)) ;
#104114=CARTESIAN_POINT('Ctrl Pts',(38.0429889324131,258.156933541317,30.0798802263626)) ;
#104115=CARTESIAN_POINT('Ctrl Pts',(38.0499858937768,258.175001311387,30.0823329269323)) ;
#104116=CARTESIAN_POINT('Ctrl Pts',(38.0602458273977,258.191447886093,30.0859311127189)) ;
#104117=CARTESIAN_POINT('Ctrl Pts',(38.0731882320494,258.205348530944,30.0904794283364)) ;
#104118=CARTESIAN_POINT('Ctrl Pts',(38.0861341004722,258.21925289602,30.095028961218)) ;
#104119=CARTESIAN_POINT('Ctrl Pts',(38.1015160468841,258.230343922473,30.1004423149597)) ;
#104120=CARTESIAN_POINT('Ctrl Pts',(38.1184645303642,258.237998568189,30.1064243414529)) ;
#104121=CARTESIAN_POINT('Ctrl Pts',(38.1347220873534,258.245341162533,30.1121625030258)) ;
#104122=CARTESIAN_POINT('Ctrl Pts',(38.1521290671494,258.249390031724,30.1183211976404)) ;
#104123=CARTESIAN_POINT('Ctrl Pts',(38.1697805624966,258.249936222763,30.1245883423369)) ;
#104124=CARTESIAN_POINT('Ctrl Pts',(38.1711545707754,258.249978738764,30.1250761825186)) ;
#104125=CARTESIAN_POINT('Ctrl Pts',(38.1725290495207,258.25,30.1255643186937)) ;
#104126=CARTESIAN_POINT('Ctrl Pts',(38.1739035596877,258.25,30.1260525975118)) ;
#104127=CARTESIAN_POINT('Origin',(40.2,258.1,25.0213203435596)) ;
#104128=CARTESIAN_POINT('Ctrl Pts',(37.580461549766,258.25,29.2213820464094)) ;
#104129=CARTESIAN_POINT('Ctrl Pts',(37.5806123754309,258.25,29.2221562239435)) ;
#104130=CARTESIAN_POINT('Ctrl Pts',(37.5807632652409,258.249996669894,29.2229303947057)) ;
#104131=CARTESIAN_POINT('Ctrl Pts',(37.5848041630347,258.249818328848,29.2436540540717)) ;
#104132=CARTESIAN_POINT('Ctrl Pts',(37.5887516260397,258.247433157513,29.2636706102593)) ;
#104133=CARTESIAN_POINT('Ctrl Pts',(37.5963119507474,258.238259809032,29.3016077085599)) ;
#104134=CARTESIAN_POINT('Ctrl Pts',(37.5999655106015,258.231622782802,29.3197493931132)) ;
#104135=CARTESIAN_POINT('Ctrl Pts',(37.6071973716956,258.21278678422,29.3553524833539)) ;
#104136=CARTESIAN_POINT('Ctrl Pts',(37.6107566001729,258.199976451841,29.3726824256129)) ;
#104137=CARTESIAN_POINT('Ctrl Pts',(37.6159573654841,258.171958342729,29.3978446898607)) ;
#104138=CARTESIAN_POINT('Ctrl Pts',(37.6178293167396,258.158041775475,29.4068396388929)) ;
#104139=CARTESIAN_POINT('Ctrl Pts',(37.6202016456472,258.129045309865,29.4182165512943)) ;
#104140=CARTESIAN_POINT('Ctrl Pts',(37.6207969906631,258.114679223254,29.4210603173112)) ;
#104141=CARTESIAN_POINT('Ctrl Pts',(37.6207969906631,258.1,29.4210603173112)) ;
#104142=CARTESIAN_POINT('Origin',(39.0797116749887,258.1,27.1578412797899)) ;
#104143=CARTESIAN_POINT('Ctrl Pts',(37.2610944621569,258.25,29.6609531317893)) ;
#104144=CARTESIAN_POINT('Ctrl Pts',(37.2622974048242,258.25,29.6617781307852)) ;
#104145=CARTESIAN_POINT('Ctrl Pts',(37.2635002136217,258.249978738764,29.6626031882028)) ;
#104146=CARTESIAN_POINT('Ctrl Pts',(37.2647025064219,258.249936222763,29.6634280389871)) ;
#104147=CARTESIAN_POINT('Ctrl Pts',(37.2801480216302,258.249390031724,29.6740246634793)) ;
#104148=CARTESIAN_POINT('Ctrl Pts',(37.2953620762498,258.245341162533,29.6844872160823)) ;
#104149=CARTESIAN_POINT('Ctrl Pts',(37.3095602987151,258.237998568188,29.6942670492256)) ;
#104150=CARTESIAN_POINT('Ctrl Pts',(37.3243619284475,258.230343922473,29.7044625134383)) ;
#104151=CARTESIAN_POINT('Ctrl Pts',(37.337782704874,258.21925289602,29.7137248799965)) ;
#104152=CARTESIAN_POINT('Ctrl Pts',(37.3490727448287,258.205348530944,29.7215241592247)) ;
#104153=CARTESIAN_POINT('Ctrl Pts',(37.3603597640426,258.191447886093,29.7293213516932)) ;
#104154=CARTESIAN_POINT('Ctrl Pts',(37.3693013951648,258.175001311387,29.7355068518133)) ;
#104155=CARTESIAN_POINT('Ctrl Pts',(37.3753983823083,258.156933541317,29.7397258512422)) ;
#104156=CARTESIAN_POINT('Ctrl Pts',(37.3814946181241,258.138867997726,29.7439443307665)) ;
#104157=CARTESIAN_POINT('Ctrl Pts',(37.3846302685632,258.119527473902,29.7461159238265)) ;
#104158=CARTESIAN_POINT('Ctrl Pts',(37.3846302685632,258.1,29.7461159238264)) ;
#104159=CARTESIAN_POINT('Origin',(40.7139068992805,258.1,27.7339145522423)) ;
#104160=CARTESIAN_POINT('',(41.293373406158,258.1,30.0027392774284)) ;
#104161=CARTESIAN_POINT('',(41.4175335996131,258.1,30.3848650607978)) ;
#104162=CARTESIAN_POINT('',(40.5712484218362,258.1,27.7802671013986)) ;
#104163=CARTESIAN_POINT('Ctrl Pts',(41.4175335996131,258.1,30.3848650607978)) ;
#104164=CARTESIAN_POINT('Ctrl Pts',(41.4175335996131,258.119527473902,30.3848650607978)) ;
#104165=CARTESIAN_POINT('Ctrl Pts',(41.4211868395563,258.138867997726,30.3837687223413)) ;
#104166=CARTESIAN_POINT('Ctrl Pts',(41.4282882862172,258.156933541317,30.3816405503694)) ;
#104167=CARTESIAN_POINT('Ctrl Pts',(41.4353906080925,258.175001311387,30.379512116112)) ;
#104168=CARTESIAN_POINT('Ctrl Pts',(41.4458060292935,258.191447886093,30.3763924718905)) ;
#104169=CARTESIAN_POINT('Ctrl Pts',(41.4589500874475,258.205348530944,30.3724647819374)) ;
#104170=CARTESIAN_POINT('Ctrl Pts',(41.4720976633411,258.21925289602,30.3685360408181)) ;
#104171=CARTESIAN_POINT('Ctrl Pts',(41.4877238088896,258.230343922473,30.3638742547393)) ;
#104172=CARTESIAN_POINT('Ctrl Pts',(41.5049515670055,258.237998568189,30.3587517471944)) ;
#104173=CARTESIAN_POINT('Ctrl Pts',(41.5214770136443,258.245341162533,30.3538380651865)) ;
#104174=CARTESIAN_POINT('Ctrl Pts',(41.5391795459882,258.249390031724,30.3485889877863)) ;
#104175=CARTESIAN_POINT('Ctrl Pts',(41.5571436409267,258.249936222763,30.3432839257019)) ;
#104176=CARTESIAN_POINT('Ctrl Pts',(41.558541982239,258.249978738764,30.3428709748963)) ;
#104177=CARTESIAN_POINT('Ctrl Pts',(41.5599408781471,258.25,30.342457987022)) ;
#104178=CARTESIAN_POINT('Ctrl Pts',(41.5613398833195,258.25,30.3420450960785)) ;
#104179=CARTESIAN_POINT('Ctrl Pts',(41.3934386691762,258.25,29.8252982934377)) ;
#104180=CARTESIAN_POINT('Ctrl Pts',(41.3930559914292,258.25,29.8259879723341)) ;
#104181=CARTESIAN_POINT('Ctrl Pts',(41.3926732547703,258.249996669894,29.8266776249672)) ;
#104182=CARTESIAN_POINT('Ctrl Pts',(41.3824261696622,258.249818328848,29.8451382901584)) ;
#104183=CARTESIAN_POINT('Ctrl Pts',(41.3724864532176,258.247433157512,29.8629553332008)) ;
#104184=CARTESIAN_POINT('Ctrl Pts',(41.3535729490475,258.238259809032,29.8966993889301)) ;
#104185=CARTESIAN_POINT('Ctrl Pts',(41.3444921183073,258.231622782802,29.9128241441556)) ;
#104186=CARTESIAN_POINT('Ctrl Pts',(41.3266122497526,258.21278678422,29.9444499271496)) ;
#104187=CARTESIAN_POINT('Ctrl Pts',(41.3178719756467,258.199976451841,29.9598318195758)) ;
#104188=CARTESIAN_POINT('Ctrl Pts',(41.3051501866381,258.171958342729,29.9821554300886)) ;
#104189=CARTESIAN_POINT('Ctrl Pts',(41.3005902630839,258.158041775475,29.9901316702288)) ;
#104190=CARTESIAN_POINT('Ctrl Pts',(41.294818384942,258.129045309865,30.0002186669547)) ;
#104191=CARTESIAN_POINT('Ctrl Pts',(41.293373406158,258.114679223254,30.0027392774284)) ;
#104192=CARTESIAN_POINT('Ctrl Pts',(41.293373406158,258.1,30.0027392774284)) ;
#104193=CARTESIAN_POINT('Origin',(38.3075320827811,258.1,27.0315026299217)) ;
#104194=CARTESIAN_POINT('Ctrl Pts',(37.0149858472034,258.25,28.8105398999439)) ;
#104195=CARTESIAN_POINT('Ctrl Pts',(37.0142029529195,258.25,28.8106356902274)) ;
#104196=CARTESIAN_POINT('Ctrl Pts',(37.0134200452556,258.249996669894,28.8107314174129)) ;
#104197=CARTESIAN_POINT('Ctrl Pts',(36.9924619678827,258.249818328848,28.8132922581644)) ;
#104198=CARTESIAN_POINT('Ctrl Pts',(36.9722052585338,258.247433157512,28.8157234537812)) ;
#104199=CARTESIAN_POINT('Ctrl Pts',(36.9337886651692,258.238259809032,28.8202563657947)) ;
#104200=CARTESIAN_POINT('Ctrl Pts',(36.9154058857742,258.231622782802,28.8223877127213)) ;
#104201=CARTESIAN_POINT('Ctrl Pts',(36.8793105668223,258.21278678422,28.8265117640394)) ;
#104202=CARTESIAN_POINT('Ctrl Pts',(36.8617289502234,258.199976451841,28.8284819832727)) ;
#104203=CARTESIAN_POINT('Ctrl Pts',(36.8361910899808,258.171958342729,28.8313113288033)) ;
#104204=CARTESIAN_POINT('Ctrl Pts',(36.8270579203394,258.158041775475,28.832310589478)) ;
#104205=CARTESIAN_POINT('Ctrl Pts',(36.815504743716,258.129045309865,28.8335700298872)) ;
#104206=CARTESIAN_POINT('Ctrl Pts',(36.8126161897874,258.114679223254,28.8338825951576)) ;
#104207=CARTESIAN_POINT('Ctrl Pts',(36.8126161897874,258.1,28.8338825951576)) ;
#104208=CARTESIAN_POINT('Ctrl Pts',(36.5764494676875,258.1,29.1589382016729)) ;
#104209=CARTESIAN_POINT('Ctrl Pts',(36.5764494676875,258.119527473902,29.1589382016729)) ;
#104210=CARTESIAN_POINT('Ctrl Pts',(36.5794837446919,258.138867997726,29.1612493232956)) ;
#104211=CARTESIAN_POINT('Ctrl Pts',(36.5853795976012,258.156933541317,29.1657436062296)) ;
#104212=CARTESIAN_POINT('Ctrl Pts',(36.5912761771422,258.175001311387,29.1702384430593)) ;
#104213=CARTESIAN_POINT('Ctrl Pts',(36.5999220533124,258.191447886093,29.1768310149482)) ;
#104214=CARTESIAN_POINT('Ctrl Pts',(36.6108255047713,258.205348530944,29.1851561431399)) ;
#104215=CARTESIAN_POINT('Ctrl Pts',(36.6217318743169,258.21925289602,29.1934834993827)) ;
#104216=CARTESIAN_POINT('Ctrl Pts',(36.6346881563825,258.230343922473,29.2033851875816)) ;
#104217=CARTESIAN_POINT('Ctrl Pts',(36.6489585741907,258.237998568189,29.2143118022826)) ;
#104218=CARTESIAN_POINT('Ctrl Pts',(36.6626472402618,258.245341162533,29.2247929796343)) ;
#104219=CARTESIAN_POINT('Ctrl Pts',(36.6772991205231,258.249390031724,29.2360292988605)) ;
#104220=CARTESIAN_POINT('Ctrl Pts',(36.6921500359814,258.249936222763,29.2474443196982)) ;
#104221=CARTESIAN_POINT('Ctrl Pts',(36.693306044602,258.249978738764,29.2483328751903)) ;
#104222=CARTESIAN_POINT('Ctrl Pts',(36.6944624091955,258.25,29.249221857571)) ;
#104223=CARTESIAN_POINT('Ctrl Pts',(36.6956187595938,258.25,29.2501109853234)) ;
#104224=CARTESIAN_POINT('Origin',(40.2,258.1,25.0213203435596)) ;
#104225=CARTESIAN_POINT('Ctrl Pts',(36.4107804436157,258.25,28.2063344963562)) ;
#104226=CARTESIAN_POINT('Ctrl Pts',(36.4106846533323,258.25,28.2071173906402)) ;
#104227=CARTESIAN_POINT('Ctrl Pts',(36.4105889261468,258.249996669894,28.2079002983041)) ;
#104228=CARTESIAN_POINT('Ctrl Pts',(36.408028085395,258.249818328848,28.228858375676)) ;
#104229=CARTESIAN_POINT('Ctrl Pts',(36.4055968897784,258.247433157512,28.2491150850256)) ;
#104230=CARTESIAN_POINT('Ctrl Pts',(36.4010639777649,258.238259809032,28.2875316783901)) ;
#104231=CARTESIAN_POINT('Ctrl Pts',(36.3989326308384,258.231622782802,28.3059144577853)) ;
#104232=CARTESIAN_POINT('Ctrl Pts',(36.3948085795202,258.21278678422,28.3420097767375)) ;
#104233=CARTESIAN_POINT('Ctrl Pts',(36.392838360287,258.199976451841,28.3595913933363)) ;
#104234=CARTESIAN_POINT('Ctrl Pts',(36.3900090147564,258.171958342729,28.3851292535788)) ;
#104235=CARTESIAN_POINT('Ctrl Pts',(36.3890097540816,258.158041775475,28.3942624232202)) ;
#104236=CARTESIAN_POINT('Ctrl Pts',(36.3877503136725,258.129045309865,28.4058155998437)) ;
#104237=CARTESIAN_POINT('Ctrl Pts',(36.387437748402,258.114679223254,28.4087041537722)) ;
#104238=CARTESIAN_POINT('Ctrl Pts',(36.387437748402,258.1,28.4087041537722)) ;
#104239=CARTESIAN_POINT('Origin',(38.4743212102356,258.1,26.7070843711341)) ;
#104240=CARTESIAN_POINT('Ctrl Pts',(35.9712093582364,258.25,28.5257015839658)) ;
#104241=CARTESIAN_POINT('Ctrl Pts',(35.9720984859886,258.25,28.5268579343639)) ;
#104242=CARTESIAN_POINT('Ctrl Pts',(35.9729874683689,258.249978738764,28.5280142989582)) ;
#104243=CARTESIAN_POINT('Ctrl Pts',(35.9738760238612,258.249936222763,28.5291703075783)) ;
#104244=CARTESIAN_POINT('Ctrl Pts',(35.9852910447034,258.249390031724,28.5440212230315)) ;
#104245=CARTESIAN_POINT('Ctrl Pts',(35.9965273639239,258.245341162533,28.5586731032987)) ;
#104246=CARTESIAN_POINT('Ctrl Pts',(36.0070085412762,258.237998568188,28.5723617693696)) ;
#104247=CARTESIAN_POINT('Ctrl Pts',(36.0179351559777,258.230343922473,28.5866321871773)) ;
#104248=CARTESIAN_POINT('Ctrl Pts',(36.0278368441767,258.21925289602,28.5995884692428)) ;
#104249=CARTESIAN_POINT('Ctrl Pts',(36.0361642004195,258.205348530944,28.6104948387885)) ;
#104250=CARTESIAN_POINT('Ctrl Pts',(36.0444893286112,258.191447886093,28.6213982902474)) ;
#104251=CARTESIAN_POINT('Ctrl Pts',(36.0510819005005,258.175001311387,28.6300441664173)) ;
#104252=CARTESIAN_POINT('Ctrl Pts',(36.0555767373301,258.156933541317,28.6359407459584)) ;
#104253=CARTESIAN_POINT('Ctrl Pts',(36.0600710202639,258.138867997726,28.6418365988678)) ;
#104254=CARTESIAN_POINT('Ctrl Pts',(36.0623821418869,258.119527473902,28.6448708758721)) ;
#104255=CARTESIAN_POINT('Ctrl Pts',(36.0623821418868,258.1,28.6448708758721)) ;
#104256=CARTESIAN_POINT('Origin',(41.5269922146558,258.1,27.4423447763876)) ;
#104257=CARTESIAN_POINT('',(42.7792030093369,258.1,29.4210603173112)) ;
#104258=CARTESIAN_POINT('',(43.0153697314369,258.1,29.7461159238265)) ;
#104259=CARTESIAN_POINT('',(41.4056396654995,258.1,27.5305125642315)) ;
#104260=CARTESIAN_POINT('Ctrl Pts',(43.0153697314369,258.1,29.7461159238265)) ;
#104261=CARTESIAN_POINT('Ctrl Pts',(43.0153697314369,258.119527473902,29.7461159238265)) ;
#104262=CARTESIAN_POINT('Ctrl Pts',(43.0185053818762,258.138867997726,29.7439443307668)) ;
#104263=CARTESIAN_POINT('Ctrl Pts',(43.0246016176919,258.156933541317,29.7397258512424)) ;
#104264=CARTESIAN_POINT('Ctrl Pts',(43.0306986048354,258.175001311387,29.7355068518134)) ;
#104265=CARTESIAN_POINT('Ctrl Pts',(43.0396402359576,258.191447886093,29.7293213516934)) ;
#104266=CARTESIAN_POINT('Ctrl Pts',(43.0509272551715,258.205348530944,29.721524159225)) ;
#104267=CARTESIAN_POINT('Ctrl Pts',(43.0622172951262,258.21925289602,29.7137248799967)) ;
#104268=CARTESIAN_POINT('Ctrl Pts',(43.0756380715528,258.230343922473,29.7044625134387)) ;
#104269=CARTESIAN_POINT('Ctrl Pts',(43.0904397012854,258.237998568188,29.6942670492262)) ;
#104270=CARTESIAN_POINT('Ctrl Pts',(43.1046379237509,258.245341162533,29.6844872160833)) ;
#104271=CARTESIAN_POINT('Ctrl Pts',(43.1198519783685,258.249390031724,29.674024663477)) ;
#104272=CARTESIAN_POINT('Ctrl Pts',(43.1352974935786,258.249936222763,29.6634280389875)) ;
#104273=CARTESIAN_POINT('Ctrl Pts',(43.1364997863788,258.249978738764,29.6626031882035)) ;
#104274=CARTESIAN_POINT('Ctrl Pts',(43.137702595176,258.25,29.6617781307852)) ;
#104275=CARTESIAN_POINT('Ctrl Pts',(43.1389055378432,258.25,29.6609531317894)) ;
#104276=CARTESIAN_POINT('Ctrl Pts',(42.8195384502335,258.25,29.2213820464098)) ;
#104277=CARTESIAN_POINT('Ctrl Pts',(42.8193876245684,258.25,29.2221562239442)) ;
#104278=CARTESIAN_POINT('Ctrl Pts',(42.8192367347592,258.249996669894,29.2229303947053)) ;
#104279=CARTESIAN_POINT('Ctrl Pts',(42.8151958369656,258.249818328848,29.2436540540713)) ;
#104280=CARTESIAN_POINT('Ctrl Pts',(42.8112483739603,258.247433157513,29.2636706102592)) ;
#104281=CARTESIAN_POINT('Ctrl Pts',(42.8036880492526,258.238259809032,29.3016077085601)) ;
#104282=CARTESIAN_POINT('Ctrl Pts',(42.8000344893985,258.231622782802,29.3197493931132)) ;
#104283=CARTESIAN_POINT('Ctrl Pts',(42.7928026283045,258.21278678422,29.3553524833537)) ;
#104284=CARTESIAN_POINT('Ctrl Pts',(42.7892433998272,258.199976451841,29.3726824256128)) ;
#104285=CARTESIAN_POINT('Ctrl Pts',(42.784042634516,258.171958342729,29.3978446898607)) ;
#104286=CARTESIAN_POINT('Ctrl Pts',(42.7821706832605,258.158041775475,29.4068396388929)) ;
#104287=CARTESIAN_POINT('Ctrl Pts',(42.7797983543528,258.129045309865,29.4182165512944)) ;
#104288=CARTESIAN_POINT('Ctrl Pts',(42.7792030093369,258.114679223254,29.4210603173112)) ;
#104289=CARTESIAN_POINT('Ctrl Pts',(42.7792030093369,258.1,29.4210603173112)) ;
#104290=CARTESIAN_POINT('Origin',(37.7789755671721,258.1,26.3483125582154)) ;
#104291=CARTESIAN_POINT('Ctrl Pts',(35.9999382971499,258.25,27.6408587937931)) ;
#104292=CARTESIAN_POINT('Ctrl Pts',(35.9991641196141,258.25,27.6407079681278)) ;
#104293=CARTESIAN_POINT('Ctrl Pts',(35.9983899488515,258.249996669894,27.6405570783182)) ;
#104294=CARTESIAN_POINT('Ctrl Pts',(35.9776662894848,258.249818328848,27.6365161805244)) ;
#104295=CARTESIAN_POINT('Ctrl Pts',(35.9576497332977,258.247433157512,27.6325687175194)) ;
#104296=CARTESIAN_POINT('Ctrl Pts',(35.9197126349983,258.238259809032,27.6250083928119)) ;
#104297=CARTESIAN_POINT('Ctrl Pts',(35.9015709504458,258.231622782802,27.621354832958)) ;
#104298=CARTESIAN_POINT('Ctrl Pts',(35.8659678602057,258.21278678422,27.6141229718641)) ;
#104299=CARTESIAN_POINT('Ctrl Pts',(35.8486379179467,258.199976451841,27.6105637433868)) ;
#104300=CARTESIAN_POINT('Ctrl Pts',(35.8234756536989,258.171958342729,27.6053629780756)) ;
#104301=CARTESIAN_POINT('Ctrl Pts',(35.8144807046667,258.158041775475,27.6034910268201)) ;
#104302=CARTESIAN_POINT('Ctrl Pts',(35.8031037922653,258.129045309865,27.6011186979124)) ;
#104303=CARTESIAN_POINT('Ctrl Pts',(35.8002600262485,258.114679223254,27.6005233528965)) ;
#104304=CARTESIAN_POINT('Ctrl Pts',(35.8002600262485,258.1,27.6005233528965)) ;
#104305=CARTESIAN_POINT('Ctrl Pts',(35.4752044197332,258.1,27.8366900749965)) ;
#104306=CARTESIAN_POINT('Ctrl Pts',(35.4752044197331,258.119527473902,27.8366900749965)) ;
#104307=CARTESIAN_POINT('Ctrl Pts',(35.4773760127932,258.138867997726,27.8398257254356)) ;
#104308=CARTESIAN_POINT('Ctrl Pts',(35.4815944923175,258.156933541317,27.8459219612513)) ;
#104309=CARTESIAN_POINT('Ctrl Pts',(35.4858134917465,258.175001311387,27.8520189483948)) ;
#104310=CARTESIAN_POINT('Ctrl Pts',(35.4919989918669,258.191447886093,27.8609605795168)) ;
#104311=CARTESIAN_POINT('Ctrl Pts',(35.4997961843353,258.205348530944,27.8722475987306)) ;
#104312=CARTESIAN_POINT('Ctrl Pts',(35.5075954635636,258.21925289602,27.8835376386854)) ;
#104313=CARTESIAN_POINT('Ctrl Pts',(35.5168578301215,258.230343922473,27.896958415112)) ;
#104314=CARTESIAN_POINT('Ctrl Pts',(35.5270532943343,258.237998568188,27.9117600448444)) ;
#104315=CARTESIAN_POINT('Ctrl Pts',(35.5368331274775,258.245341162533,27.9259582673097)) ;
#104316=CARTESIAN_POINT('Ctrl Pts',(35.547295680081,258.249390031724,27.9411723219293)) ;
#104317=CARTESIAN_POINT('Ctrl Pts',(35.5578923045725,258.249936222763,27.9566178371378)) ;
#104318=CARTESIAN_POINT('Ctrl Pts',(35.5587171553567,258.249978738764,27.957820129938)) ;
#104319=CARTESIAN_POINT('Ctrl Pts',(35.5595422127747,258.25,27.9590229387353)) ;
#104320=CARTESIAN_POINT('Ctrl Pts',(35.5603672117705,258.25,27.9602258814026)) ;
#104321=CARTESIAN_POINT('Origin',(40.2,258.1,25.0213203435596)) ;
#104322=CARTESIAN_POINT('Ctrl Pts',(35.6120145486888,258.25,26.8795155697285)) ;
#104323=CARTESIAN_POINT('Ctrl Pts',(35.611681519077,258.25,26.8802305456133)) ;
#104324=CARTESIAN_POINT('Ctrl Pts',(35.6113485453403,258.249996669894,26.8809455537216)) ;
#104325=CARTESIAN_POINT('Ctrl Pts',(35.6024366389787,258.249818328848,26.9000865264635)) ;
#104326=CARTESIAN_POINT('Ctrl Pts',(35.593864767106,258.247433157512,26.9186005211265)) ;
#104327=CARTESIAN_POINT('Ctrl Pts',(35.5776823313821,258.238259809032,26.9537361257336)) ;
#104328=CARTESIAN_POINT('Ctrl Pts',(35.5699747087623,258.231622782802,26.9705605654438)) ;
#104329=CARTESIAN_POINT('Ctrl Pts',(35.5548984359091,258.21278678422,27.0036148517977)) ;
#104330=CARTESIAN_POINT('Ctrl Pts',(35.5475916277511,258.199976451841,27.0197271316054)) ;
#104331=CARTESIAN_POINT('Ctrl Pts',(35.5370091274324,258.171958342729,27.0431407641495)) ;
#104332=CARTESIAN_POINT('Ctrl Pts',(35.5332364694246,258.158041775475,27.051518136121)) ;
#104333=CARTESIAN_POINT('Ctrl Pts',(35.5284685425009,258.129045309865,27.0621166715428)) ;
#104334=CARTESIAN_POINT('Ctrl Pts',(35.5272786630106,258.114679223254,27.0647672615988)) ;
#104335=CARTESIAN_POINT('Ctrl Pts',(35.5272786630106,258.1,27.0647672615988)) ;
#104336=CARTESIAN_POINT('Origin',(38.0378522089358,258.1,26.0913131340507)) ;
#104337=CARTESIAN_POINT('Ctrl Pts',(35.0952677460484,258.25,27.0474167838717)) ;
#104338=CARTESIAN_POINT('Ctrl Pts',(35.0957560248665,258.25,27.0487912940387)) ;
#104339=CARTESIAN_POINT('Ctrl Pts',(35.096244161041,258.249978738764,27.0501657727844)) ;
#104340=CARTESIAN_POINT('Ctrl Pts',(35.0967320012227,258.249936222763,27.0515397810631)) ;
#104341=CARTESIAN_POINT('Ctrl Pts',(35.1029991459195,258.249390031724,27.0691912764099)) ;
#104342=CARTESIAN_POINT('Ctrl Pts',(35.109157840533,258.245341162533,27.0865982562064)) ;
#104343=CARTESIAN_POINT('Ctrl Pts',(35.114896002106,258.237998568189,27.1028558131956)) ;
#104344=CARTESIAN_POINT('Ctrl Pts',(35.1208780285994,258.230343922473,27.1198042966759)) ;
#104345=CARTESIAN_POINT('Ctrl Pts',(35.1262913823413,258.21925289602,27.1351862430876)) ;
#104346=CARTESIAN_POINT('Ctrl Pts',(35.1308409152229,258.205348530944,27.1481321115103)) ;
#104347=CARTESIAN_POINT('Ctrl Pts',(35.1353892308406,258.191447886093,27.161074516162)) ;
#104348=CARTESIAN_POINT('Ctrl Pts',(35.1389874166276,258.175001311387,27.1713344497828)) ;
#104349=CARTESIAN_POINT('Ctrl Pts',(35.1414401171973,258.156933541317,27.1783314111464)) ;
#104350=CARTESIAN_POINT('Ctrl Pts',(35.1438925155223,258.138867997726,27.1853275102791)) ;
#104351=CARTESIAN_POINT('Ctrl Pts',(35.1451528796413,258.119527473902,27.1889274550539)) ;
#104352=CARTESIAN_POINT('Ctrl Pts',(35.1451528796413,258.1,27.1889274550539)) ;
#104353=CARTESIAN_POINT('Origin',(42.2101822863621,258.1,26.9137882607786)) ;
#104354=CARTESIAN_POINT('',(44.012562251598,258.1,28.4087041537722)) ;
#104355=CARTESIAN_POINT('',(44.3376178581133,258.1,28.6448708758722)) ;
#104356=CARTESIAN_POINT('',(42.1220144985182,258.1,27.0351408099348)) ;
#104357=CARTESIAN_POINT('Ctrl Pts',(44.3376178581132,258.1,28.6448708758722)) ;
#104358=CARTESIAN_POINT('Ctrl Pts',(44.3376178581133,258.119527473902,28.6448708758722)) ;
#104359=CARTESIAN_POINT('Ctrl Pts',(44.339928979736,258.138867997726,28.6418365988678)) ;
#104360=CARTESIAN_POINT('Ctrl Pts',(44.3444232626699,258.156933541317,28.6359407459585)) ;
#104361=CARTESIAN_POINT('Ctrl Pts',(44.3489180994996,258.175001311387,28.6300441664175)) ;
#104362=CARTESIAN_POINT('Ctrl Pts',(44.3555106713886,258.191447886093,28.6213982902472)) ;
#104363=CARTESIAN_POINT('Ctrl Pts',(44.3638357995803,258.205348530944,28.6104948387884)) ;
#104364=CARTESIAN_POINT('Ctrl Pts',(44.3721631558231,258.21925289602,28.5995884692428)) ;
#104365=CARTESIAN_POINT('Ctrl Pts',(44.382064844023,258.230343922473,28.5866321871781)) ;
#104366=CARTESIAN_POINT('Ctrl Pts',(44.3929914587245,258.237998568189,28.5723617693702)) ;
#104367=CARTESIAN_POINT('Ctrl Pts',(44.4034726360766,258.245341162533,28.5586731032994)) ;
#104368=CARTESIAN_POINT('Ctrl Pts',(44.414708955301,258.249390031724,28.5440212230371)) ;
#104369=CARTESIAN_POINT('Ctrl Pts',(44.4261239761384,258.249936222763,28.5291703075781)) ;
#104370=CARTESIAN_POINT('Ctrl Pts',(44.4270125316305,258.249978738764,28.5280142989574)) ;
#104371=CARTESIAN_POINT('Ctrl Pts',(44.4279015140117,258.25,28.5268579343646)) ;
#104372=CARTESIAN_POINT('Ctrl Pts',(44.4287906417641,258.25,28.5257015839662)) ;
#104373=CARTESIAN_POINT('Ctrl Pts',(43.9892195563843,258.25,28.2063344963563)) ;
#104374=CARTESIAN_POINT('Ctrl Pts',(43.9893153466677,258.25,28.2071173906402)) ;
#104375=CARTESIAN_POINT('Ctrl Pts',(43.9894110738533,258.249996669894,28.2079002983041)) ;
#104376=CARTESIAN_POINT('Ctrl Pts',(43.9919719146048,258.249818328848,28.2288583756768)) ;
#104377=CARTESIAN_POINT('Ctrl Pts',(43.9944031102216,258.247433157512,28.2491150850258)) ;
#104378=CARTESIAN_POINT('Ctrl Pts',(43.9989360222351,258.238259809032,28.2875316783904)) ;
#104379=CARTESIAN_POINT('Ctrl Pts',(44.0010673691616,258.231622782802,28.3059144577855)) ;
#104380=CARTESIAN_POINT('Ctrl Pts',(44.0051914204798,258.21278678422,28.3420097767374)) ;
#104381=CARTESIAN_POINT('Ctrl Pts',(44.0071616397131,258.199976451841,28.3595913933363)) ;
#104382=CARTESIAN_POINT('Ctrl Pts',(44.0099909852437,258.171958342729,28.3851292535789)) ;
#104383=CARTESIAN_POINT('Ctrl Pts',(44.0109902459184,258.158041775475,28.3942624232203)) ;
#104384=CARTESIAN_POINT('Ctrl Pts',(44.0122496863275,258.129045309865,28.4058155998437)) ;
#104385=CARTESIAN_POINT('Ctrl Pts',(44.012562251598,258.114679223254,28.4087041537722)) ;
#104386=CARTESIAN_POINT('Ctrl Pts',(44.012562251598,258.1,28.4087041537722)) ;
#104387=CARTESIAN_POINT('Origin',(37.4874057913173,258.1,25.5352272428401)) ;
#104388=CARTESIAN_POINT('Ctrl Pts',(35.3960220501219,258.25,26.2147590127358)) ;
#104389=CARTESIAN_POINT('Ctrl Pts',(35.3953323712255,258.25,26.2143763349887)) ;
#104390=CARTESIAN_POINT('Ctrl Pts',(35.3946427185925,258.249996669894,26.2139935983299)) ;
#104391=CARTESIAN_POINT('Ctrl Pts',(35.3761820534011,258.249818328848,26.2037465132217)) ;
#104392=CARTESIAN_POINT('Ctrl Pts',(35.3583650103588,258.247433157512,26.1938067967771)) ;
#104393=CARTESIAN_POINT('Ctrl Pts',(35.3246209546296,258.238259809032,26.1748932926071)) ;
#104394=CARTESIAN_POINT('Ctrl Pts',(35.3084961994042,258.231622782802,26.1658124618669)) ;
#104395=CARTESIAN_POINT('Ctrl Pts',(35.2768704164101,258.21278678422,26.1479325933122)) ;
#104396=CARTESIAN_POINT('Ctrl Pts',(35.2614885239839,258.199976451842,26.1391923192063)) ;
#104397=CARTESIAN_POINT('Ctrl Pts',(35.2391649134711,258.171958342729,26.1264705301978)) ;
#104398=CARTESIAN_POINT('Ctrl Pts',(35.2311886733309,258.158041775475,26.1219106066435)) ;
#104399=CARTESIAN_POINT('Ctrl Pts',(35.2211016766049,258.129045309865,26.1161387285016)) ;
#104400=CARTESIAN_POINT('Ctrl Pts',(35.2185810661312,258.114679223254,26.1146937497175)) ;
#104401=CARTESIAN_POINT('Ctrl Pts',(35.2185810661312,258.1,26.1146937497175)) ;
#104402=CARTESIAN_POINT('Ctrl Pts',(34.8364552827617,258.1,26.2388539431727)) ;
#104403=CARTESIAN_POINT('Ctrl Pts',(34.8364552827616,258.119527473902,26.2388539431727)) ;
#104404=CARTESIAN_POINT('Ctrl Pts',(34.837551621218,258.138867997726,26.242507183116)) ;
#104405=CARTESIAN_POINT('Ctrl Pts',(34.8396797931898,258.156933541317,26.2496086297769)) ;
#104406=CARTESIAN_POINT('Ctrl Pts',(34.8418082274472,258.175001311387,26.2567109516523)) ;
#104407=CARTESIAN_POINT('Ctrl Pts',(34.8449278716689,258.191447886093,26.2671263728531)) ;
#104408=CARTESIAN_POINT('Ctrl Pts',(34.848855561622,258.205348530944,26.2802704310072)) ;
#104409=CARTESIAN_POINT('Ctrl Pts',(34.8527843027412,258.21925289602,26.2934180069008)) ;
#104410=CARTESIAN_POINT('Ctrl Pts',(34.85744608882,258.230343922473,26.3090441524493)) ;
#104411=CARTESIAN_POINT('Ctrl Pts',(34.8625685963648,258.237998568189,26.3262719105653)) ;
#104412=CARTESIAN_POINT('Ctrl Pts',(34.8674822783726,258.245341162533,26.3427973572041)) ;
#104413=CARTESIAN_POINT('Ctrl Pts',(34.8727313557738,258.249390031724,26.3604998895481)) ;
#104414=CARTESIAN_POINT('Ctrl Pts',(34.8780364178575,258.249936222763,26.3784639844864)) ;
#104415=CARTESIAN_POINT('Ctrl Pts',(34.878449368663,258.249978738764,26.3798623257986)) ;
#104416=CARTESIAN_POINT('Ctrl Pts',(34.8788623565375,258.25,26.3812612217067)) ;
#104417=CARTESIAN_POINT('Ctrl Pts',(34.8792752474809,258.25,26.3826602268792)) ;
#104418=CARTESIAN_POINT('Origin',(40.2,258.1,25.0213203435596)) ;
#104419=CARTESIAN_POINT('Ctrl Pts',(35.2623526361106,258.25,25.3708035475559)) ;
#104420=CARTESIAN_POINT('Ctrl Pts',(35.2618149664292,258.25,25.3713806182205)) ;
#104421=CARTESIAN_POINT('Ctrl Pts',(35.2612773399305,258.249996669894,25.3719577367977)) ;
#104422=CARTESIAN_POINT('Ctrl Pts',(35.2468867274466,258.249818328848,25.3874079531342)) ;
#104423=CARTESIAN_POINT('Ctrl Pts',(35.2330132538606,258.247433157512,25.4023669543188)) ;
#104424=CARTESIAN_POINT('Ctrl Pts',(35.2067653439847,258.238259809032,25.4307822523853)) ;
#104425=CARTESIAN_POINT('Ctrl Pts',(35.1942359214756,258.231622782802,25.4444014590289)) ;
#104426=CARTESIAN_POINT('Ctrl Pts',(35.1696831977168,258.21278678422,25.4711791289339)) ;
#104427=CARTESIAN_POINT('Ctrl Pts',(35.1577550419262,258.199976451841,25.4842448897419)) ;
#104428=CARTESIAN_POINT('Ctrl Pts',(35.1404552756832,258.171958342729,25.5032424051016)) ;
#104429=CARTESIAN_POINT('Ctrl Pts',(35.1342785143937,258.158041775475,25.5100439438662)) ;
#104430=CARTESIAN_POINT('Ctrl Pts',(35.1264688188629,258.129045309865,25.5186503795949)) ;
#104431=CARTESIAN_POINT('Ctrl Pts',(35.1245180988476,258.114679223254,25.5208035475559)) ;
#104432=CARTESIAN_POINT('Ctrl Pts',(35.1245180988476,258.1,25.5208035475559)) ;
#104433=CARTESIAN_POINT('Origin',(37.8130292979948,258.1,25.3708035475559)) ;
#104434=CARTESIAN_POINT('Ctrl Pts',(34.7190128936385,258.25,25.3708035475559)) ;
#104435=CARTESIAN_POINT('Ctrl Pts',(34.7190525273897,258.25,25.3722616708597)) ;
#104436=CARTESIAN_POINT('Ctrl Pts',(34.7190920351885,258.249978738764,25.3737197202007)) ;
#104437=CARTESIAN_POINT('Ctrl Pts',(34.7191314068636,258.249936222763,25.3751772306343)) ;
#104438=CARTESIAN_POINT('Ctrl Pts',(34.7196372036263,258.249390031724,25.3939014545243)) ;
#104439=CARTESIAN_POINT('Ctrl Pts',(34.7201154176929,258.245341162533,25.4123596173872)) ;
#104440=CARTESIAN_POINT('Ctrl Pts',(34.720548872252,258.237998568188,25.4295946623432)) ;
#104441=CARTESIAN_POINT('Ctrl Pts',(34.7210007481052,258.230343922473,25.4475621758456)) ;
#104442=CARTESIAN_POINT('Ctrl Pts',(34.7213958706096,258.21925289602,25.4638640945166)) ;
#104443=CARTESIAN_POINT('Ctrl Pts',(34.7217222401531,258.205348530944,25.4775822300161)) ;
#104444=CARTESIAN_POINT('Ctrl Pts',(34.7220485223739,258.191447886093,25.4912966951182)) ;
#104445=CARTESIAN_POINT('Ctrl Pts',(34.7223001065631,258.175001311387,25.5021663724021)) ;
#104446=CARTESIAN_POINT('Ctrl Pts',(34.7224705834521,258.156933541317,25.5095788042595)) ;
#104447=CARTESIAN_POINT('Ctrl Pts',(34.7226410393334,258.138867997726,25.5169903226876)) ;
#104448=CARTESIAN_POINT('Ctrl Pts',(34.7227272727275,258.119527473902,25.5208035475559)) ;
#104449=CARTESIAN_POINT('Ctrl Pts',(34.7227272727275,258.1,25.5208035475559)) ;
#104450=CARTESIAN_POINT('Origin',(42.6966017101158,258.1,26.1999837998328)) ;
#104451=CARTESIAN_POINT('',(44.8727213369894,258.1,27.0647672615988)) ;
#104452=CARTESIAN_POINT('',(45.2548471203588,258.1,27.188927455054)) ;
#104453=CARTESIAN_POINT('',(42.6502491609595,258.1,26.3426422772771)) ;
#104454=CARTESIAN_POINT('Ctrl Pts',(45.2548471203589,258.1,27.188927455054)) ;
#104455=CARTESIAN_POINT('Ctrl Pts',(45.2548471203587,258.119527473902,27.1889274550539)) ;
#104456=CARTESIAN_POINT('Ctrl Pts',(45.2561074844781,258.138867997726,27.1853275102792)) ;
#104457=CARTESIAN_POINT('Ctrl Pts',(45.2585598828031,258.156933541317,27.1783314111465)) ;
#104458=CARTESIAN_POINT('Ctrl Pts',(45.2610125833727,258.175001311387,27.1713344497829)) ;
#104459=CARTESIAN_POINT('Ctrl Pts',(45.2646107691594,258.191447886093,27.1610745161619)) ;
#104460=CARTESIAN_POINT('Ctrl Pts',(45.2691590847769,258.205348530944,27.1481321115102)) ;
#104461=CARTESIAN_POINT('Ctrl Pts',(45.2737086176586,258.21925289602,27.1351862430874)) ;
#104462=CARTESIAN_POINT('Ctrl Pts',(45.2791219714006,258.230343922473,27.1198042966759)) ;
#104463=CARTESIAN_POINT('Ctrl Pts',(45.2851039978943,258.237998568188,27.1028558131957)) ;
#104464=CARTESIAN_POINT('Ctrl Pts',(45.2908421594676,258.245341162533,27.0865982562065)) ;
#104465=CARTESIAN_POINT('Ctrl Pts',(45.2970008540775,258.249390031724,27.0691912764082)) ;
#104466=CARTESIAN_POINT('Ctrl Pts',(45.3032679987774,258.249936222763,27.051539781063)) ;
#104467=CARTESIAN_POINT('Ctrl Pts',(45.3037558389593,258.249978738764,27.0501657727844)) ;
#104468=CARTESIAN_POINT('Ctrl Pts',(45.3042439751347,258.25,27.0487912940391)) ;
#104469=CARTESIAN_POINT('Ctrl Pts',(45.3047322539528,258.25,27.0474167838722)) ;
#104470=CARTESIAN_POINT('Ctrl Pts',(44.7879854513112,258.25,26.8795155697285)) ;
#104471=CARTESIAN_POINT('Ctrl Pts',(44.7883184809236,258.25,26.8802305456146)) ;
#104472=CARTESIAN_POINT('Ctrl Pts',(44.7886514546609,258.249996669894,26.8809455537241)) ;
#104473=CARTESIAN_POINT('Ctrl Pts',(44.7975633610227,258.249818328848,26.9000865264659)) ;
#104474=CARTESIAN_POINT('Ctrl Pts',(44.8061352328951,258.247433157512,26.9186005211289)) ;
#104475=CARTESIAN_POINT('Ctrl Pts',(44.8223176686183,258.238259809031,26.9537361257345)) ;
#104476=CARTESIAN_POINT('Ctrl Pts',(44.8300252912379,258.231622782802,26.9705605654442)) ;
#104477=CARTESIAN_POINT('Ctrl Pts',(44.845101564091,258.21278678422,27.0036148517979)) ;
#104478=CARTESIAN_POINT('Ctrl Pts',(44.8524083722489,258.199976451841,27.0197271316054)) ;
#104479=CARTESIAN_POINT('Ctrl Pts',(44.8629908725676,258.171958342729,27.0431407641494)) ;
#104480=CARTESIAN_POINT('Ctrl Pts',(44.8667635305755,258.158041775475,27.051518136121)) ;
#104481=CARTESIAN_POINT('Ctrl Pts',(44.8715314574991,258.129045309865,27.0621166715428)) ;
#104482=CARTESIAN_POINT('Ctrl Pts',(44.8727213369894,258.114679223254,27.0647672615988)) ;
#104483=CARTESIAN_POINT('Ctrl Pts',(44.8727213369894,258.1,27.0647672615988)) ;
#104484=CARTESIAN_POINT('Origin',(37.4613636363637,258.1,24.6718371395634)) ;
#104485=CARTESIAN_POINT('Ctrl Pts',(35.2623526361106,258.25,24.6718371395634)) ;
#104486=CARTESIAN_POINT('Ctrl Pts',(35.2618149664301,258.25,24.6712600688998)) ;
#104487=CARTESIAN_POINT('Ctrl Pts',(35.2612773399324,258.249996669894,24.6706829503236)) ;
#104488=CARTESIAN_POINT('Ctrl Pts',(35.2468867274488,258.249818328848,24.6552327339874)) ;
#104489=CARTESIAN_POINT('Ctrl Pts',(35.2330132538624,258.247433157513,24.6402737328024)) ;
#104490=CARTESIAN_POINT('Ctrl Pts',(35.2067653439856,258.238259809032,24.611858434735)) ;
#104491=CARTESIAN_POINT('Ctrl Pts',(35.1942359214761,258.231622782802,24.5982392280908)) ;
#104492=CARTESIAN_POINT('Ctrl Pts',(35.1696831977168,258.21278678422,24.5714615581854)) ;
#104493=CARTESIAN_POINT('Ctrl Pts',(35.1577550419262,258.199976451841,24.5583957973774)) ;
#104494=CARTESIAN_POINT('Ctrl Pts',(35.1404552756832,258.171958342729,24.5393982820177)) ;
#104495=CARTESIAN_POINT('Ctrl Pts',(35.1342785143937,258.158041775475,24.5325967432531)) ;
#104496=CARTESIAN_POINT('Ctrl Pts',(35.1264688188629,258.129045309865,24.5239903075244)) ;
#104497=CARTESIAN_POINT('Ctrl Pts',(35.1245180988476,258.114679223254,24.5218371395634)) ;
#104498=CARTESIAN_POINT('Ctrl Pts',(35.1245180988476,258.1,24.5218371395634)) ;
#104499=CARTESIAN_POINT('Ctrl Pts',(34.7227272727271,258.1,24.5218371395634)) ;
#104500=CARTESIAN_POINT('Ctrl Pts',(34.7227272727271,258.119527473902,24.5218371395634)) ;
#104501=CARTESIAN_POINT('Ctrl Pts',(34.722641039333,258.138867997726,24.5256503644317)) ;
#104502=CARTESIAN_POINT('Ctrl Pts',(34.7224705834517,258.156933541317,24.5330618828598)) ;
#104503=CARTESIAN_POINT('Ctrl Pts',(34.7223001065627,258.175001311387,24.5404743147172)) ;
#104504=CARTESIAN_POINT('Ctrl Pts',(34.7220485223736,258.191447886093,24.5513439920011)) ;
#104505=CARTESIAN_POINT('Ctrl Pts',(34.7217222401528,258.205348530944,24.5650584571032)) ;
#104506=CARTESIAN_POINT('Ctrl Pts',(34.7213958706093,258.21925289602,24.5787765926027)) ;
#104507=CARTESIAN_POINT('Ctrl Pts',(34.7210007481061,258.230343922473,24.5950785112738)) ;
#104508=CARTESIAN_POINT('Ctrl Pts',(34.7205488722535,258.237998568189,24.6130460247761)) ;
#104509=CARTESIAN_POINT('Ctrl Pts',(34.720115417695,258.245341162533,24.6302810697322)) ;
#104510=CARTESIAN_POINT('Ctrl Pts',(34.7196372036259,258.249390031724,24.6487392325953)) ;
#104511=CARTESIAN_POINT('Ctrl Pts',(34.7191314068632,258.249936222763,24.6674634564849)) ;
#104512=CARTESIAN_POINT('Ctrl Pts',(34.7190920351881,258.249978738764,24.6689209669185)) ;
#104513=CARTESIAN_POINT('Ctrl Pts',(34.7190525273894,258.25,24.6703790162596)) ;
#104514=CARTESIAN_POINT('Ctrl Pts',(34.7190128936382,258.25,24.6718371395634)) ;
#104515=CARTESIAN_POINT('Origin',(40.2,258.1,25.0213203435596)) ;
#104516=CARTESIAN_POINT('Ctrl Pts',(35.3960220501219,258.25,23.8278816743835)) ;
#104517=CARTESIAN_POINT('Ctrl Pts',(35.3953323712255,258.25,23.8282643521305)) ;
#104518=CARTESIAN_POINT('Ctrl Pts',(35.3946427185925,258.249996669894,23.8286470887893)) ;
#104519=CARTESIAN_POINT('Ctrl Pts',(35.3761820534012,258.249818328848,23.8388941738976)) ;
#104520=CARTESIAN_POINT('Ctrl Pts',(35.3583650103588,258.247433157512,23.8488338903421)) ;
#104521=CARTESIAN_POINT('Ctrl Pts',(35.3246209546295,258.238259809032,23.8677473945122)) ;
#104522=CARTESIAN_POINT('Ctrl Pts',(35.3084961994041,258.231622782802,23.8768282252524)) ;
#104523=CARTESIAN_POINT('Ctrl Pts',(35.27687041641,258.21278678422,23.8947080938071)) ;
#104524=CARTESIAN_POINT('Ctrl Pts',(35.2614885239839,258.199976451841,23.903448367913)) ;
#104525=CARTESIAN_POINT('Ctrl Pts',(35.2391649134711,258.171958342729,23.9161701569215)) ;
#104526=CARTESIAN_POINT('Ctrl Pts',(35.2311886733309,258.158041775475,23.9207300804757)) ;
#104527=CARTESIAN_POINT('Ctrl Pts',(35.2211016766049,258.129045309865,23.9265019586177)) ;
#104528=CARTESIAN_POINT('Ctrl Pts',(35.2185810661312,258.114679223254,23.9279469374017)) ;
#104529=CARTESIAN_POINT('Ctrl Pts',(35.2185810661312,258.1,23.9279469374017)) ;
#104530=CARTESIAN_POINT('Origin',(37.8218597103689,258.1,24.6160841100613)) ;
#104531=CARTESIAN_POINT('Ctrl Pts',(34.8792752474813,258.25,23.6599804602402)) ;
#104532=CARTESIAN_POINT('Ctrl Pts',(34.8788623565378,258.25,23.6613794654126)) ;
#104533=CARTESIAN_POINT('Ctrl Pts',(34.8784493686632,258.249978738764,23.6627783613207)) ;
#104534=CARTESIAN_POINT('Ctrl Pts',(34.8780364178576,258.249936222763,23.6641767026329)) ;
#104535=CARTESIAN_POINT('Ctrl Pts',(34.8727313557735,258.249390031724,23.6821407975715)) ;
#104536=CARTESIAN_POINT('Ctrl Pts',(34.8674822783725,258.245341162533,23.6998433299152)) ;
#104537=CARTESIAN_POINT('Ctrl Pts',(34.8625685963647,258.237998568189,23.716368776554)) ;
#104538=CARTESIAN_POINT('Ctrl Pts',(34.85744608882,258.230343922473,23.7335965346698)) ;
#104539=CARTESIAN_POINT('Ctrl Pts',(34.852784302741,258.21925289602,23.7492226802184)) ;
#104540=CARTESIAN_POINT('Ctrl Pts',(34.8488555616218,258.205348530944,23.762370256112)) ;
#104541=CARTESIAN_POINT('Ctrl Pts',(34.8449278716688,258.191447886093,23.7755143142661)) ;
#104542=CARTESIAN_POINT('Ctrl Pts',(34.841808227447,258.175001311387,23.7859297354669)) ;
#104543=CARTESIAN_POINT('Ctrl Pts',(34.8396797931897,258.156933541317,23.7930320573423)) ;
#104544=CARTESIAN_POINT('Ctrl Pts',(34.8375516212179,258.138867997726,23.8001335040032)) ;
#104545=CARTESIAN_POINT('Ctrl Pts',(34.8364552827619,258.119527473902,23.8037867439466)) ;
#104546=CARTESIAN_POINT('Ctrl Pts',(34.8364552827619,258.1,23.8037867439466)) ;
#104547=CARTESIAN_POINT('Origin',(42.9386363636364,258.1,25.3708035475559)) ;
#104548=CARTESIAN_POINT('',(45.2754819011524,258.1,25.5208035475559)) ;
#104549=CARTESIAN_POINT('',(45.6772727272728,258.1,25.5208035475559)) ;
#104550=CARTESIAN_POINT('',(42.9386363636364,258.1,25.5208035475559)) ;
#104551=CARTESIAN_POINT('Ctrl Pts',(45.6772727272728,258.1,25.5208035475559)) ;
#104552=CARTESIAN_POINT('Ctrl Pts',(45.6772727272728,258.119527473902,25.5208035475559)) ;
#104553=CARTESIAN_POINT('Ctrl Pts',(45.6773589606669,258.138867997726,25.5169903226876)) ;
#104554=CARTESIAN_POINT('Ctrl Pts',(45.6775294165481,258.156933541317,25.5095788042595)) ;
#104555=CARTESIAN_POINT('Ctrl Pts',(45.6776998934371,258.175001311387,25.5021663724021)) ;
#104556=CARTESIAN_POINT('Ctrl Pts',(45.6779514776262,258.191447886093,25.4912966951182)) ;
#104557=CARTESIAN_POINT('Ctrl Pts',(45.6782777598469,258.205348530944,25.4775822300161)) ;
#104558=CARTESIAN_POINT('Ctrl Pts',(45.6786041293904,258.21925289602,25.4638640945166)) ;
#104559=CARTESIAN_POINT('Ctrl Pts',(45.6789992518937,258.230343922473,25.4475621758455)) ;
#104560=CARTESIAN_POINT('Ctrl Pts',(45.6794511277462,258.237998568189,25.4295946623431)) ;
#104561=CARTESIAN_POINT('Ctrl Pts',(45.6798845823047,258.245341162533,25.4123596173871)) ;
#104562=CARTESIAN_POINT('Ctrl Pts',(45.6803627963736,258.249390031724,25.3939014545241)) ;
#104563=CARTESIAN_POINT('Ctrl Pts',(45.6808685931367,258.249936222763,25.3751772306343)) ;
#104564=CARTESIAN_POINT('Ctrl Pts',(45.6809079648118,258.249978738764,25.3737197202007)) ;
#104565=CARTESIAN_POINT('Ctrl Pts',(45.6809474726105,258.25,25.3722616708597)) ;
#104566=CARTESIAN_POINT('Ctrl Pts',(45.6809871063617,258.25,25.3708035475559)) ;
#104567=CARTESIAN_POINT('Ctrl Pts',(45.1376473638895,258.25,25.3708035475559)) ;
#104568=CARTESIAN_POINT('Ctrl Pts',(45.1381850335699,258.25,25.3713806182195)) ;
#104569=CARTESIAN_POINT('Ctrl Pts',(45.1387226600676,258.249996669894,25.3719577367957)) ;
#104570=CARTESIAN_POINT('Ctrl Pts',(45.1531132725512,258.249818328848,25.3874079531319)) ;
#104571=CARTESIAN_POINT('Ctrl Pts',(45.1669867461377,258.247433157513,25.4023669543169)) ;
#104572=CARTESIAN_POINT('Ctrl Pts',(45.1932346560144,258.238259809032,25.4307822523842)) ;
#104573=CARTESIAN_POINT('Ctrl Pts',(45.205764078524,258.231622782802,25.4444014590284)) ;
#104574=CARTESIAN_POINT('Ctrl Pts',(45.2303168022832,258.21278678422,25.4711791289339)) ;
#104575=CARTESIAN_POINT('Ctrl Pts',(45.2422449580739,258.199976451841,25.4842448897419)) ;
#104576=CARTESIAN_POINT('Ctrl Pts',(45.2595447243168,258.171958342729,25.5032424051016)) ;
#104577=CARTESIAN_POINT('Ctrl Pts',(45.2657214856064,258.158041775475,25.5100439438662)) ;
#104578=CARTESIAN_POINT('Ctrl Pts',(45.2735311811371,258.129045309865,25.5186503795949)) ;
#104579=CARTESIAN_POINT('Ctrl Pts',(45.2754819011524,258.114679223254,25.5208035475559)) ;
#104580=CARTESIAN_POINT('Ctrl Pts',(45.2754819011524,258.1,25.5208035475559)) ;
#104581=CARTESIAN_POINT('Origin',(37.7033982898842,258.1,23.8426568872864)) ;
#104582=CARTESIAN_POINT('Ctrl Pts',(35.6120145486888,258.25,23.1631251173908)) ;
#104583=CARTESIAN_POINT('Ctrl Pts',(35.611681519077,258.25,23.162410141506)) ;
#104584=CARTESIAN_POINT('Ctrl Pts',(35.6113485453403,258.249996669894,23.1616951333977)) ;
#104585=CARTESIAN_POINT('Ctrl Pts',(35.6024366389787,258.249818328848,23.1425541606558)) ;
#104586=CARTESIAN_POINT('Ctrl Pts',(35.593864767106,258.247433157512,23.1240401659927)) ;
#104587=CARTESIAN_POINT('Ctrl Pts',(35.5776823313822,258.238259809032,23.0889045613858)) ;
#104588=CARTESIAN_POINT('Ctrl Pts',(35.5699747087623,258.231622782802,23.0720801216756)) ;
#104589=CARTESIAN_POINT('Ctrl Pts',(35.5548984359091,258.21278678422,23.0390258353215)) ;
#104590=CARTESIAN_POINT('Ctrl Pts',(35.5475916277511,258.199976451841,23.0229135555139)) ;
#104591=CARTESIAN_POINT('Ctrl Pts',(35.5370091274324,258.171958342729,22.9994999229698)) ;
#104592=CARTESIAN_POINT('Ctrl Pts',(35.5332364694246,258.158041775475,22.9911225509982)) ;
#104593=CARTESIAN_POINT('Ctrl Pts',(35.5284685425009,258.129045309865,22.9805240155765)) ;
#104594=CARTESIAN_POINT('Ctrl Pts',(35.5272786630106,258.114679223254,22.9778734255204)) ;
#104595=CARTESIAN_POINT('Ctrl Pts',(35.5272786630106,258.1,22.9778734255204)) ;
#104596=CARTESIAN_POINT('Ctrl Pts',(35.1451528796411,258.1,22.8537132320652)) ;
#104597=CARTESIAN_POINT('Ctrl Pts',(35.1451528796411,258.119527473902,22.8537132320652)) ;
#104598=CARTESIAN_POINT('Ctrl Pts',(35.1438925155222,258.138867997726,22.8573131768401)) ;
#104599=CARTESIAN_POINT('Ctrl Pts',(35.1414401171971,258.156933541317,22.8643092759728)) ;
#104600=CARTESIAN_POINT('Ctrl Pts',(35.1389874166274,258.175001311387,22.8713062373364)) ;
#104601=CARTESIAN_POINT('Ctrl Pts',(35.1353892308407,258.191447886093,22.8815661709573)) ;
#104602=CARTESIAN_POINT('Ctrl Pts',(35.1308409152232,258.205348530944,22.894508575609)) ;
#104603=CARTESIAN_POINT('Ctrl Pts',(35.1262913823417,258.21925289602,22.9074544440319)) ;
#104604=CARTESIAN_POINT('Ctrl Pts',(35.1208780285999,258.230343922473,22.9228363904437)) ;
#104605=CARTESIAN_POINT('Ctrl Pts',(35.1148960021068,258.237998568189,22.9397848739239)) ;
#104606=CARTESIAN_POINT('Ctrl Pts',(35.109157840534,258.245341162533,22.9560424309131)) ;
#104607=CARTESIAN_POINT('Ctrl Pts',(35.1029991459193,258.249390031724,22.9734494107092)) ;
#104608=CARTESIAN_POINT('Ctrl Pts',(35.0967320012226,258.249936222763,22.9911009060562)) ;
#104609=CARTESIAN_POINT('Ctrl Pts',(35.0962441610409,258.249978738764,22.992474914335)) ;
#104610=CARTESIAN_POINT('Ctrl Pts',(35.0957560248659,258.25,22.9938493930803)) ;
#104611=CARTESIAN_POINT('Ctrl Pts',(35.0952677460478,258.25,22.9952239032473)) ;
#104612=CARTESIAN_POINT('Origin',(40.2,258.1,25.0213203435596)) ;
#104613=CARTESIAN_POINT('Ctrl Pts',(35.9999382971499,258.25,22.4017818933262)) ;
#104614=CARTESIAN_POINT('Ctrl Pts',(35.9991641196141,258.25,22.4019327189915)) ;
#104615=CARTESIAN_POINT('Ctrl Pts',(35.9983899488515,258.249996669894,22.402083608801)) ;
#104616=CARTESIAN_POINT('Ctrl Pts',(35.9776662894848,258.249818328848,22.4061245065949)) ;
#104617=CARTESIAN_POINT('Ctrl Pts',(35.9576497332977,258.247433157512,22.4100719696)) ;
#104618=CARTESIAN_POINT('Ctrl Pts',(35.9197126349982,258.238259809032,22.4176322943074)) ;
#104619=CARTESIAN_POINT('Ctrl Pts',(35.9015709504457,258.231622782802,22.4212858541613)) ;
#104620=CARTESIAN_POINT('Ctrl Pts',(35.8659678602058,258.21278678422,22.4285177152552)) ;
#104621=CARTESIAN_POINT('Ctrl Pts',(35.8486379179467,258.199976451841,22.4320769437325)) ;
#104622=CARTESIAN_POINT('Ctrl Pts',(35.823475653699,258.171958342729,22.4372777090437)) ;
#104623=CARTESIAN_POINT('Ctrl Pts',(35.8144807046667,258.158041775475,22.4391496602992)) ;
#104624=CARTESIAN_POINT('Ctrl Pts',(35.8031037922653,258.129045309865,22.4415219892068)) ;
#104625=CARTESIAN_POINT('Ctrl Pts',(35.8002600262485,258.114679223254,22.4421173342227)) ;
#104626=CARTESIAN_POINT('Ctrl Pts',(35.8002600262485,258.1,22.4421173342227)) ;
#104627=CARTESIAN_POINT('Origin',(38.0634790637697,258.1,23.9010320185483)) ;
#104628=CARTESIAN_POINT('Ctrl Pts',(35.5603672117703,258.25,22.0824148057165)) ;
#104629=CARTESIAN_POINT('Ctrl Pts',(35.5595422127744,258.25,22.0836177483838)) ;
#104630=CARTESIAN_POINT('Ctrl Pts',(35.5587171553568,258.249978738764,22.0848205571812)) ;
#104631=CARTESIAN_POINT('Ctrl Pts',(35.5578923045725,258.249936222763,22.0860228499814)) ;
#104632=CARTESIAN_POINT('Ctrl Pts',(35.54729568008,258.249390031724,22.1014683651895)) ;
#104633=CARTESIAN_POINT('Ctrl Pts',(35.5368331274791,258.245341162533,22.1166824198106)) ;
#104634=CARTESIAN_POINT('Ctrl Pts',(35.5270532943355,258.237998568189,22.1308806422756)) ;
#104635=CARTESIAN_POINT('Ctrl Pts',(35.5168578301224,258.230343922473,22.1456822720076)) ;
#104636=CARTESIAN_POINT('Ctrl Pts',(35.5075954635632,258.21925289602,22.1591030484335)) ;
#104637=CARTESIAN_POINT('Ctrl Pts',(35.4997961843348,258.205348530944,22.1703930883883)) ;
#104638=CARTESIAN_POINT('Ctrl Pts',(35.4919989918663,258.191447886093,22.1816801076021)) ;
#104639=CARTESIAN_POINT('Ctrl Pts',(35.4858134917463,258.175001311387,22.1906217387244)) ;
#104640=CARTESIAN_POINT('Ctrl Pts',(35.4815944923173,258.156933541317,22.1967187258679)) ;
#104641=CARTESIAN_POINT('Ctrl Pts',(35.477376012793,258.138867997726,22.2028149616836)) ;
#104642=CARTESIAN_POINT('Ctrl Pts',(35.4752044197329,258.119527473902,22.2059506121226)) ;
#104643=CARTESIAN_POINT('Ctrl Pts',(35.475204419733,258.1,22.2059506121227)) ;
#104644=CARTESIAN_POINT('Origin',(42.9125942086827,258.1,24.5074134442792)) ;
#104645=CARTESIAN_POINT('',(45.1814189338688,258.1,23.9279469374017)) ;
#104646=CARTESIAN_POINT('',(45.5635447172382,258.1,23.8037867439466)) ;
#104647=CARTESIAN_POINT('',(42.9589467578389,258.1,24.6500719217234)) ;
#104648=CARTESIAN_POINT('Ctrl Pts',(45.5635447172382,258.1,23.8037867439466)) ;
#104649=CARTESIAN_POINT('Ctrl Pts',(45.5635447172384,258.119527473902,23.8037867439465)) ;
#104650=CARTESIAN_POINT('Ctrl Pts',(45.5624483787821,258.138867997726,23.8001335040032)) ;
#104651=CARTESIAN_POINT('Ctrl Pts',(45.5603202068104,258.156933541317,23.7930320573423)) ;
#104652=CARTESIAN_POINT('Ctrl Pts',(45.5581917725532,258.175001311387,23.7859297354669)) ;
#104653=CARTESIAN_POINT('Ctrl Pts',(45.5550721283311,258.191447886093,23.7755143142662)) ;
#104654=CARTESIAN_POINT('Ctrl Pts',(45.551144438378,258.205348530944,23.7623702561121)) ;
#104655=CARTESIAN_POINT('Ctrl Pts',(45.5472156972587,258.21925289602,23.7492226802186)) ;
#104656=CARTESIAN_POINT('Ctrl Pts',(45.5425539111806,258.230343922473,23.7335965346699)) ;
#104657=CARTESIAN_POINT('Ctrl Pts',(45.5374314036356,258.237998568189,23.716368776554)) ;
#104658=CARTESIAN_POINT('Ctrl Pts',(45.5325177216277,258.245341162533,23.6998433299152)) ;
#104659=CARTESIAN_POINT('Ctrl Pts',(45.5272686442365,258.249390031724,23.6821407975691)) ;
#104660=CARTESIAN_POINT('Ctrl Pts',(45.5219635821412,258.249936222763,23.6641767026333)) ;
#104661=CARTESIAN_POINT('Ctrl Pts',(45.5215506313346,258.249978738764,23.6627783613209)) ;
#104662=CARTESIAN_POINT('Ctrl Pts',(45.5211376434632,258.25,23.6613794654128)) ;
#104663=CARTESIAN_POINT('Ctrl Pts',(45.5207247525196,258.25,23.65998046024)) ;
#104664=CARTESIAN_POINT('Ctrl Pts',(45.0039779498781,258.25,23.8278816743835)) ;
#104665=CARTESIAN_POINT('Ctrl Pts',(45.0046676287764,258.25,23.8282643521315)) ;
#104666=CARTESIAN_POINT('Ctrl Pts',(45.0053572814057,258.249996669895,23.8286470887883)) ;
#104667=CARTESIAN_POINT('Ctrl Pts',(45.0238179465998,258.249818328848,23.8388941738985)) ;
#104668=CARTESIAN_POINT('Ctrl Pts',(45.0416349896415,258.247433157512,23.8488338903423)) ;
#104669=CARTESIAN_POINT('Ctrl Pts',(45.0753790453705,258.238259809032,23.8677473945122)) ;
#104670=CARTESIAN_POINT('Ctrl Pts',(45.091503800596,258.231622782802,23.8768282252524)) ;
#104671=CARTESIAN_POINT('Ctrl Pts',(45.1231295835901,258.21278678422,23.8947080938071)) ;
#104672=CARTESIAN_POINT('Ctrl Pts',(45.1385114760162,258.199976451841,23.903448367913)) ;
#104673=CARTESIAN_POINT('Ctrl Pts',(45.1608350865288,258.171958342729,23.9161701569214)) ;
#104674=CARTESIAN_POINT('Ctrl Pts',(45.1688113266691,258.158041775475,23.9207300804757)) ;
#104675=CARTESIAN_POINT('Ctrl Pts',(45.1788983233951,258.129045309865,23.9265019586177)) ;
#104676=CARTESIAN_POINT('Ctrl Pts',(45.1814189338688,258.114679223254,23.9279469374017)) ;
#104677=CARTESIAN_POINT('Ctrl Pts',(45.1814189338688,258.1,23.9279469374017)) ;
#104678=CARTESIAN_POINT('Origin',(38.1898177136379,258.1,23.1288524263407)) ;
#104679=CARTESIAN_POINT('Ctrl Pts',(36.4107804436157,258.25,21.836306190763)) ;
#104680=CARTESIAN_POINT('Ctrl Pts',(36.410684653332,258.25,21.835523296477)) ;
#104681=CARTESIAN_POINT('Ctrl Pts',(36.410588926147,258.249996669895,21.8347403888173)) ;
#104682=CARTESIAN_POINT('Ctrl Pts',(36.4080280853953,258.249818328848,21.8137823114415)) ;
#104683=CARTESIAN_POINT('Ctrl Pts',(36.4055968897784,258.247433157512,21.7935256020932)) ;
#104684=CARTESIAN_POINT('Ctrl Pts',(36.4010639777649,258.238259809032,21.7551090087287)) ;
#104685=CARTESIAN_POINT('Ctrl Pts',(36.3989326308384,258.231622782802,21.7367262293337)) ;
#104686=CARTESIAN_POINT('Ctrl Pts',(36.3948085795202,258.21278678422,21.7006309103817)) ;
#104687=CARTESIAN_POINT('Ctrl Pts',(36.392838360287,258.199976451841,21.6830492937829)) ;
#104688=CARTESIAN_POINT('Ctrl Pts',(36.3900090147564,258.171958342729,21.6575114335404)) ;
#104689=CARTESIAN_POINT('Ctrl Pts',(36.3890097540817,258.158041775475,21.648378263899)) ;
#104690=CARTESIAN_POINT('Ctrl Pts',(36.3877503136725,258.129045309865,21.6368250872756)) ;
#104691=CARTESIAN_POINT('Ctrl Pts',(36.3874377484021,258.114679223254,21.633936533347)) ;
#104692=CARTESIAN_POINT('Ctrl Pts',(36.3874377484021,258.1,21.633936533347)) ;
#104693=CARTESIAN_POINT('Ctrl Pts',(36.0623821418867,258.1,21.3977698112471)) ;
#104694=CARTESIAN_POINT('Ctrl Pts',(36.0623821418865,258.119527473902,21.3977698112469)) ;
#104695=CARTESIAN_POINT('Ctrl Pts',(36.060071020264,258.138867997726,21.4008040882515)) ;
#104696=CARTESIAN_POINT('Ctrl Pts',(36.05557673733,258.156933541317,21.4066999411607)) ;
#104697=CARTESIAN_POINT('Ctrl Pts',(36.0510819005001,258.175001311387,21.4125965207016)) ;
#104698=CARTESIAN_POINT('Ctrl Pts',(36.0444893286114,258.191447886093,21.421242396872)) ;
#104699=CARTESIAN_POINT('Ctrl Pts',(36.0361642004197,258.205348530944,21.4321458483309)) ;
#104700=CARTESIAN_POINT('Ctrl Pts',(36.0278368441769,258.21925289602,21.4430522178765)) ;
#104701=CARTESIAN_POINT('Ctrl Pts',(36.0179351559774,258.230343922473,21.4560084999414)) ;
#104702=CARTESIAN_POINT('Ctrl Pts',(36.0070085412762,258.237998568188,21.4702789177496)) ;
#104703=CARTESIAN_POINT('Ctrl Pts',(35.9965273639244,258.245341162533,21.4839675838205)) ;
#104704=CARTESIAN_POINT('Ctrl Pts',(35.9852910446948,258.249390031724,21.4986194640775)) ;
#104705=CARTESIAN_POINT('Ctrl Pts',(35.9738760238622,258.249936222763,21.5134703795415)) ;
#104706=CARTESIAN_POINT('Ctrl Pts',(35.9729874683704,258.249978738764,21.5146263881627)) ;
#104707=CARTESIAN_POINT('Ctrl Pts',(35.9720984859888,258.25,21.5157827527548)) ;
#104708=CARTESIAN_POINT('Ctrl Pts',(35.9712093582363,258.25,21.5169391031534)) ;
#104709=CARTESIAN_POINT('Origin',(40.2,258.1,25.0213203435596)) ;
#104710=CARTESIAN_POINT('Ctrl Pts',(37.0149858472034,258.25,21.2321007871753)) ;
#104711=CARTESIAN_POINT('Ctrl Pts',(37.0142029529195,258.25,21.2320049968919)) ;
#104712=CARTESIAN_POINT('Ctrl Pts',(37.0134200452556,258.249996669894,21.2319092697064)) ;
#104713=CARTESIAN_POINT('Ctrl Pts',(36.9924619678836,258.249818328848,21.2293484289546)) ;
#104714=CARTESIAN_POINT('Ctrl Pts',(36.972205258534,258.247433157512,21.226917233338)) ;
#104715=CARTESIAN_POINT('Ctrl Pts',(36.9337886651695,258.238259809032,21.2223843213245)) ;
#104716=CARTESIAN_POINT('Ctrl Pts',(36.9154058857743,258.231622782802,21.220252974398)) ;
#104717=CARTESIAN_POINT('Ctrl Pts',(36.8793105668222,258.21278678422,21.2161289230798)) ;
#104718=CARTESIAN_POINT('Ctrl Pts',(36.8617289502234,258.199976451841,21.2141587038466)) ;
#104719=CARTESIAN_POINT('Ctrl Pts',(36.8361910899808,258.171958342729,21.211329358316)) ;
#104720=CARTESIAN_POINT('Ctrl Pts',(36.8270579203394,258.158041775475,21.2103300976413)) ;
#104721=CARTESIAN_POINT('Ctrl Pts',(36.815504743716,258.129045309865,21.2090706572321)) ;
#104722=CARTESIAN_POINT('Ctrl Pts',(36.8126161897874,258.114679223254,21.2087580919617)) ;
#104723=CARTESIAN_POINT('Ctrl Pts',(36.8126161897874,258.1,21.2087580919617)) ;
#104724=CARTESIAN_POINT('Origin',(38.5142359724255,258.1,23.2956415537952)) ;
#104725=CARTESIAN_POINT('Ctrl Pts',(36.6956187595937,258.25,20.7925297017959)) ;
#104726=CARTESIAN_POINT('Ctrl Pts',(36.6944624091956,258.25,20.7934188295481)) ;
#104727=CARTESIAN_POINT('Ctrl Pts',(36.6933060446015,258.249978738764,20.7943078119286)) ;
#104728=CARTESIAN_POINT('Ctrl Pts',(36.6921500359814,258.249936222763,20.795196367421)) ;
#104729=CARTESIAN_POINT('Ctrl Pts',(36.6772991205284,258.249390031724,20.8066113882632)) ;
#104730=CARTESIAN_POINT('Ctrl Pts',(36.6626472402613,258.245341162533,20.8178477074839)) ;
#104731=CARTESIAN_POINT('Ctrl Pts',(36.6489585741903,258.237998568189,20.8283288848361)) ;
#104732=CARTESIAN_POINT('Ctrl Pts',(36.6346881563824,258.230343922473,20.8392554995376)) ;
#104733=CARTESIAN_POINT('Ctrl Pts',(36.6217318743171,258.21925289602,20.8491571877367)) ;
#104734=CARTESIAN_POINT('Ctrl Pts',(36.6108255047715,258.205348530944,20.8574845439796)) ;
#104735=CARTESIAN_POINT('Ctrl Pts',(36.5999220533126,258.191447886093,20.8658096721713)) ;
#104736=CARTESIAN_POINT('Ctrl Pts',(36.5912761771423,258.175001311387,20.8724022440602)) ;
#104737=CARTESIAN_POINT('Ctrl Pts',(36.5853795976013,258.156933541317,20.8768970808899)) ;
#104738=CARTESIAN_POINT('Ctrl Pts',(36.5794837446919,258.138867997726,20.8813913638238)) ;
#104739=CARTESIAN_POINT('Ctrl Pts',(36.5764494676877,258.119527473902,20.8837024854467)) ;
#104740=CARTESIAN_POINT('Ctrl Pts',(36.5764494676876,258.1,20.8837024854466)) ;
#104741=CARTESIAN_POINT('Origin',(42.621024432828,258.1,23.6943281289039)) ;
#104742=CARTESIAN_POINT('',(44.5997399737516,258.1,22.4421173342227)) ;
#104743=CARTESIAN_POINT('',(44.9247955802669,258.1,22.2059506121228)) ;
#104744=CARTESIAN_POINT('',(42.7091922206719,258.1,23.8156806780601)) ;
#104745=CARTESIAN_POINT('Ctrl Pts',(44.9247955802669,258.1,22.2059506121228)) ;
#104746=CARTESIAN_POINT('Ctrl Pts',(44.9247955802668,258.119527473902,22.2059506121229)) ;
#104747=CARTESIAN_POINT('Ctrl Pts',(44.922623987207,258.138867997726,22.2028149616837)) ;
#104748=CARTESIAN_POINT('Ctrl Pts',(44.9184055076825,258.156933541317,22.196718725868)) ;
#104749=CARTESIAN_POINT('Ctrl Pts',(44.9141865082535,258.175001311387,22.1906217387246)) ;
#104750=CARTESIAN_POINT('Ctrl Pts',(44.9080010081334,258.191447886093,22.1816801076024)) ;
#104751=CARTESIAN_POINT('Ctrl Pts',(44.9002038156649,258.205348530944,22.1703930883885)) ;
#104752=CARTESIAN_POINT('Ctrl Pts',(44.8924045364365,258.21925289602,22.1591030484337)) ;
#104753=CARTESIAN_POINT('Ctrl Pts',(44.8831421698776,258.230343922473,22.1456822720076)) ;
#104754=CARTESIAN_POINT('Ctrl Pts',(44.872946705665,258.237998568189,22.1308806422754)) ;
#104755=CARTESIAN_POINT('Ctrl Pts',(44.8631668725217,258.245341162533,22.1166824198098)) ;
#104756=CARTESIAN_POINT('Ctrl Pts',(44.8527043199125,258.249390031724,22.101468365193)) ;
#104757=CARTESIAN_POINT('Ctrl Pts',(44.8421076954281,258.249936222763,22.086022849981)) ;
#104758=CARTESIAN_POINT('Ctrl Pts',(44.8412828446445,258.249978738764,22.0848205571807)) ;
#104759=CARTESIAN_POINT('Ctrl Pts',(44.8404577872252,258.25,22.0836177483837)) ;
#104760=CARTESIAN_POINT('Ctrl Pts',(44.8396327882295,258.25,22.0824148057166)) ;
#104761=CARTESIAN_POINT('Ctrl Pts',(44.4000617028502,258.25,22.4017818933262)) ;
#104762=CARTESIAN_POINT('Ctrl Pts',(44.400835880386,258.25,22.4019327189915)) ;
#104763=CARTESIAN_POINT('Ctrl Pts',(44.4016100511485,258.249996669894,22.4020836088011)) ;
#104764=CARTESIAN_POINT('Ctrl Pts',(44.4223337105146,258.249818328848,22.4061245065945)) ;
#104765=CARTESIAN_POINT('Ctrl Pts',(44.4423502667022,258.247433157512,22.4100719695999)) ;
#104766=CARTESIAN_POINT('Ctrl Pts',(44.4802873650017,258.238259809032,22.4176322943074)) ;
#104767=CARTESIAN_POINT('Ctrl Pts',(44.4984290495542,258.231622782802,22.4212858541613)) ;
#104768=CARTESIAN_POINT('Ctrl Pts',(44.5340321397943,258.21278678422,22.4285177152552)) ;
#104769=CARTESIAN_POINT('Ctrl Pts',(44.5513620820533,258.199976451841,22.4320769437325)) ;
#104770=CARTESIAN_POINT('Ctrl Pts',(44.5765243463011,258.171958342729,22.4372777090437)) ;
#104771=CARTESIAN_POINT('Ctrl Pts',(44.5855192953333,258.158041775475,22.4391496602992)) ;
#104772=CARTESIAN_POINT('Ctrl Pts',(44.5968962077348,258.129045309865,22.4415219892068)) ;
#104773=CARTESIAN_POINT('Ctrl Pts',(44.5997399737516,258.114679223254,22.4421173342227)) ;
#104774=CARTESIAN_POINT('Ctrl Pts',(44.5997399737516,258.1,22.4421173342227)) ;
#104775=CARTESIAN_POINT('Origin',(38.8730077853443,258.1,22.6002959107317)) ;
#104776=CARTESIAN_POINT('Ctrl Pts',(37.5804615497666,258.25,20.8212586407095)) ;
#104777=CARTESIAN_POINT('Ctrl Pts',(37.5806123754319,258.25,20.8204844631737)) ;
#104778=CARTESIAN_POINT('Ctrl Pts',(37.5807632652414,258.249996669894,20.8197102924111)) ;
#104779=CARTESIAN_POINT('Ctrl Pts',(37.5848041630348,258.249818328848,20.7989866330451)) ;
#104780=CARTESIAN_POINT('Ctrl Pts',(37.5887516260403,258.247433157512,20.7789700768575)) ;
#104781=CARTESIAN_POINT('Ctrl Pts',(37.5963119507477,258.238259809032,20.7410329785581)) ;
#104782=CARTESIAN_POINT('Ctrl Pts',(37.5999655106017,258.231622782802,20.7228912940055)) ;
#104783=CARTESIAN_POINT('Ctrl Pts',(37.6071973716956,258.21278678422,20.6872882037655)) ;
#104784=CARTESIAN_POINT('Ctrl Pts',(37.6107566001728,258.199976451841,20.6699582615064)) ;
#104785=CARTESIAN_POINT('Ctrl Pts',(37.615957365484,258.171958342729,20.6447959972586)) ;
#104786=CARTESIAN_POINT('Ctrl Pts',(37.6178293167396,258.158041775475,20.6358010482264)) ;
#104787=CARTESIAN_POINT('Ctrl Pts',(37.6202016456472,258.129045309865,20.6244241358249)) ;
#104788=CARTESIAN_POINT('Ctrl Pts',(37.6207969906631,258.114679223254,20.6215803698081)) ;
#104789=CARTESIAN_POINT('Ctrl Pts',(37.6207969906631,258.1,20.6215803698081)) ;
#104790=CARTESIAN_POINT('Ctrl Pts',(37.384630268563,258.1,20.2965247632925)) ;
#104791=CARTESIAN_POINT('Ctrl Pts',(37.384630268563,258.119527473902,20.2965247632926)) ;
#104792=CARTESIAN_POINT('Ctrl Pts',(37.3814946181239,258.138867997726,20.2986963563525)) ;
#104793=CARTESIAN_POINT('Ctrl Pts',(37.3753983823082,258.156933541317,20.302914835877)) ;
#104794=CARTESIAN_POINT('Ctrl Pts',(37.3693013951648,258.175001311387,20.307133835306)) ;
#104795=CARTESIAN_POINT('Ctrl Pts',(37.3603597640427,258.191447886093,20.3133193354261)) ;
#104796=CARTESIAN_POINT('Ctrl Pts',(37.3490727448288,258.205348530944,20.3211165278946)) ;
#104797=CARTESIAN_POINT('Ctrl Pts',(37.337782704874,258.21925289602,20.328915807123)) ;
#104798=CARTESIAN_POINT('Ctrl Pts',(37.324361928448,258.230343922473,20.338178173682)) ;
#104799=CARTESIAN_POINT('Ctrl Pts',(37.3095602987158,258.237998568189,20.3483736378947)) ;
#104800=CARTESIAN_POINT('Ctrl Pts',(37.2953620762502,258.245341162533,20.358153471038)) ;
#104801=CARTESIAN_POINT('Ctrl Pts',(37.280148021633,258.249390031724,20.3686160236467)) ;
#104802=CARTESIAN_POINT('Ctrl Pts',(37.2647025064213,258.249936222763,20.3792126481315)) ;
#104803=CARTESIAN_POINT('Ctrl Pts',(37.263500213621,258.249978738764,20.3800374989151)) ;
#104804=CARTESIAN_POINT('Ctrl Pts',(37.262297404824,258.25,20.3808625563344)) ;
#104805=CARTESIAN_POINT('Ctrl Pts',(37.261094462157,258.25,20.3816875553301)) ;
#104806=CARTESIAN_POINT('Origin',(40.2,258.1,25.0213203435596)) ;
#104807=CARTESIAN_POINT('Ctrl Pts',(38.3418047738312,258.25,20.4333348922484)) ;
#104808=CARTESIAN_POINT('Ctrl Pts',(38.3410897979463,258.25,20.4330018626367)) ;
#104809=CARTESIAN_POINT('Ctrl Pts',(38.3403747898381,258.249996669894,20.4326688888999)) ;
#104810=CARTESIAN_POINT('Ctrl Pts',(38.3212338170963,258.249818328848,20.4237569825383)) ;
#104811=CARTESIAN_POINT('Ctrl Pts',(38.3027198224331,258.247433157512,20.4151851106656)) ;
#104812=CARTESIAN_POINT('Ctrl Pts',(38.267584217826,258.238259809032,20.3990026749417)) ;
#104813=CARTESIAN_POINT('Ctrl Pts',(38.2507597781159,258.231622782802,20.3912950523219)) ;
#104814=CARTESIAN_POINT('Ctrl Pts',(38.2177054917619,258.21278678422,20.3762187794687)) ;
#104815=CARTESIAN_POINT('Ctrl Pts',(38.2015932119542,258.199976451841,20.3689119713107)) ;
#104816=CARTESIAN_POINT('Ctrl Pts',(38.1781795794102,258.171958342729,20.3583294709921)) ;
#104817=CARTESIAN_POINT('Ctrl Pts',(38.1698022074386,258.158041775475,20.3545568129842)) ;
#104818=CARTESIAN_POINT('Ctrl Pts',(38.1592036720168,258.129045309865,20.3497888860605)) ;
#104819=CARTESIAN_POINT('Ctrl Pts',(38.1565530819608,258.114679223254,20.3485990065702)) ;
#104820=CARTESIAN_POINT('Ctrl Pts',(38.1565530819608,258.1,20.3485990065702)) ;
#104821=CARTESIAN_POINT('Origin',(39.1300072095089,258.1,22.8591725524954)) ;
#104822=CARTESIAN_POINT('Ctrl Pts',(38.1739035596879,258.25,19.9165880896081)) ;
#104823=CARTESIAN_POINT('Ctrl Pts',(38.172529049521,258.25,19.9170763684262)) ;
#104824=CARTESIAN_POINT('Ctrl Pts',(38.1711545707754,258.249978738764,19.9175645046008)) ;
#104825=CARTESIAN_POINT('Ctrl Pts',(38.1697805624967,258.249936222763,19.9180523447825)) ;
#104826=CARTESIAN_POINT('Ctrl Pts',(38.1521290671494,258.249390031724,19.9243194894788)) ;
#104827=CARTESIAN_POINT('Ctrl Pts',(38.1347220873532,258.245341162533,19.9304781840928)) ;
#104828=CARTESIAN_POINT('Ctrl Pts',(38.1184645303641,258.237998568189,19.9362163456658)) ;
#104829=CARTESIAN_POINT('Ctrl Pts',(38.1015160468838,258.230343922473,19.9421983721592)) ;
#104830=CARTESIAN_POINT('Ctrl Pts',(38.0861341004721,258.21925289602,19.9476117259011)) ;
#104831=CARTESIAN_POINT('Ctrl Pts',(38.0731882320494,258.205348530944,19.9521612587827)) ;
#104832=CARTESIAN_POINT('Ctrl Pts',(38.0602458273977,258.191447886093,19.9567095744004)) ;
#104833=CARTESIAN_POINT('Ctrl Pts',(38.0499858937768,258.175001311387,19.9603077601871)) ;
#104834=CARTESIAN_POINT('Ctrl Pts',(38.0429889324132,258.156933541317,19.9627604607569)) ;
#104835=CARTESIAN_POINT('Ctrl Pts',(38.0359928332805,258.138867997726,19.9652128590819)) ;
#104836=CARTESIAN_POINT('Ctrl Pts',(38.0323928885057,258.119527473902,19.9664732232009)) ;
#104837=CARTESIAN_POINT('Ctrl Pts',(38.0323928885057,258.1,19.9664732232009)) ;
#104838=CARTESIAN_POINT('Origin',(42.0924679172189,258.1,23.0111380571975)) ;
#104839=CARTESIAN_POINT('',(43.5873838102126,258.1,21.2087580919617)) ;
#104840=CARTESIAN_POINT('',(43.8235505323125,258.1,20.8837024854464)) ;
#104841=CARTESIAN_POINT('',(42.2138204663752,258.1,23.0993058450414)) ;
#104842=CARTESIAN_POINT('Ctrl Pts',(43.8235505323125,258.1,20.8837024854464)) ;
#104843=CARTESIAN_POINT('Ctrl Pts',(43.8235505323124,258.119527473902,20.8837024854464)) ;
#104844=CARTESIAN_POINT('Ctrl Pts',(43.8205162553077,258.138867997726,20.8813913638241)) ;
#104845=CARTESIAN_POINT('Ctrl Pts',(43.8146204023984,258.156933541317,20.8768970808903)) ;
#104846=CARTESIAN_POINT('Ctrl Pts',(43.8087238228574,258.175001311387,20.8724022440606)) ;
#104847=CARTESIAN_POINT('Ctrl Pts',(43.8000779466875,258.191447886093,20.8658096721712)) ;
#104848=CARTESIAN_POINT('Ctrl Pts',(43.7891744952286,258.205348530944,20.8574845439795)) ;
#104849=CARTESIAN_POINT('Ctrl Pts',(43.7782681256829,258.21925289602,20.8491571877368)) ;
#104850=CARTESIAN_POINT('Ctrl Pts',(43.7653118436174,258.230343922473,20.8392554995377)) ;
#104851=CARTESIAN_POINT('Ctrl Pts',(43.7510414258095,258.237998568189,20.8283288848364)) ;
#104852=CARTESIAN_POINT('Ctrl Pts',(43.7373527597384,258.245341162533,20.8178477074844)) ;
#104853=CARTESIAN_POINT('Ctrl Pts',(43.7227008794732,258.249390031724,20.8066113882618)) ;
#104854=CARTESIAN_POINT('Ctrl Pts',(43.7078499640187,258.249936222763,20.7951963674209)) ;
#104855=CARTESIAN_POINT('Ctrl Pts',(43.7066939553985,258.249978738764,20.7943078119287)) ;
#104856=CARTESIAN_POINT('Ctrl Pts',(43.7055375908041,258.25,20.7934188295486)) ;
#104857=CARTESIAN_POINT('Ctrl Pts',(43.7043812404059,258.25,20.7925297017964)) ;
#104858=CARTESIAN_POINT('Ctrl Pts',(43.3850141527966,258.25,21.2321007871753)) ;
#104859=CARTESIAN_POINT('Ctrl Pts',(43.3857970470805,258.25,21.2320049968919)) ;
#104860=CARTESIAN_POINT('Ctrl Pts',(43.3865799547445,258.249996669894,21.2319092697064)) ;
#104861=CARTESIAN_POINT('Ctrl Pts',(43.4075380321166,258.249818328848,21.2293484289546)) ;
#104862=CARTESIAN_POINT('Ctrl Pts',(43.4277947414661,258.247433157512,21.226917233338)) ;
#104863=CARTESIAN_POINT('Ctrl Pts',(43.4662113348306,258.238259809032,21.2223843213245)) ;
#104864=CARTESIAN_POINT('Ctrl Pts',(43.4845941142257,258.231622782802,21.220252974398)) ;
#104865=CARTESIAN_POINT('Ctrl Pts',(43.5206894331777,258.21278678422,21.2161289230799)) ;
#104866=CARTESIAN_POINT('Ctrl Pts',(43.5382710497766,258.199976451841,21.2141587038466)) ;
#104867=CARTESIAN_POINT('Ctrl Pts',(43.5638089100192,258.171958342729,21.211329358316)) ;
#104868=CARTESIAN_POINT('Ctrl Pts',(43.5729420796606,258.158041775475,21.2103300976413)) ;
#104869=CARTESIAN_POINT('Ctrl Pts',(43.584495256284,258.129045309865,21.2090706572321)) ;
#104870=CARTESIAN_POINT('Ctrl Pts',(43.5873838102126,258.114679223254,21.2087580919617)) ;
#104871=CARTESIAN_POINT('Ctrl Pts',(43.5873838102126,258.1,21.2087580919617)) ;
#104872=CARTESIAN_POINT('Origin',(39.6860931007195,258.1,22.3087261348769)) ;
#104873=CARTESIAN_POINT('Ctrl Pts',(39.0065613308239,258.25,20.2173423936815)) ;
#104874=CARTESIAN_POINT('Ctrl Pts',(39.0069440085709,258.25,20.2166527147851)) ;
#104875=CARTESIAN_POINT('Ctrl Pts',(39.0073267452297,258.249996669894,20.2159630621521)) ;
#104876=CARTESIAN_POINT('Ctrl Pts',(39.0175738303378,258.249818328848,20.197502396961)) ;
#104877=CARTESIAN_POINT('Ctrl Pts',(39.0275135467826,258.247433157512,20.1796853539185)) ;
#104878=CARTESIAN_POINT('Ctrl Pts',(39.0464270509528,258.238259809032,20.1459412981889)) ;
#104879=CARTESIAN_POINT('Ctrl Pts',(39.0555078816928,258.231622782802,20.1298165429636)) ;
#104880=CARTESIAN_POINT('Ctrl Pts',(39.0733877502474,258.21278678422,20.0981907599697)) ;
#104881=CARTESIAN_POINT('Ctrl Pts',(39.0821280243534,258.199976451841,20.0828088675435)) ;
#104882=CARTESIAN_POINT('Ctrl Pts',(39.0948498133619,258.171958342729,20.0604852570307)) ;
#104883=CARTESIAN_POINT('Ctrl Pts',(39.0994097369161,258.158041775475,20.0525090168905)) ;
#104884=CARTESIAN_POINT('Ctrl Pts',(39.1051816150581,258.129045309865,20.0424220201645)) ;
#104885=CARTESIAN_POINT('Ctrl Pts',(39.1066265938421,258.114679223254,20.0399014096908)) ;
#104886=CARTESIAN_POINT('Ctrl Pts',(39.1066265938421,258.1,20.0399014096908)) ;
#104887=CARTESIAN_POINT('Ctrl Pts',(38.982466400387,258.1,19.6577756263215)) ;
#104888=CARTESIAN_POINT('Ctrl Pts',(38.9824664003869,258.119527473902,19.6577756263214)) ;
#104889=CARTESIAN_POINT('Ctrl Pts',(38.9788131604436,258.138867997726,19.6588719647777)) ;
#104890=CARTESIAN_POINT('Ctrl Pts',(38.9717117137828,258.156933541317,19.6610001367495)) ;
#104891=CARTESIAN_POINT('Ctrl Pts',(38.9646093919074,258.175001311387,19.6631285710069)) ;
#104892=CARTESIAN_POINT('Ctrl Pts',(38.9541939707066,258.191447886093,19.6662482152287)) ;
#104893=CARTESIAN_POINT('Ctrl Pts',(38.9410499125525,258.205348530944,19.6701759051818)) ;
#104894=CARTESIAN_POINT('Ctrl Pts',(38.9279023366589,258.21925289602,19.674104646301)) ;
#104895=CARTESIAN_POINT('Ctrl Pts',(38.9122761911104,258.230343922473,19.6787664323798)) ;
#104896=CARTESIAN_POINT('Ctrl Pts',(38.8950484329945,258.237998568189,19.6838889399248)) ;
#104897=CARTESIAN_POINT('Ctrl Pts',(38.8785229863557,258.245341162533,19.6888026219327)) ;
#104898=CARTESIAN_POINT('Ctrl Pts',(38.8608204540116,258.249390031724,19.6940516993334)) ;
#104899=CARTESIAN_POINT('Ctrl Pts',(38.8428563590732,258.249936222763,19.6993567614171)) ;
#104900=CARTESIAN_POINT('Ctrl Pts',(38.841458017761,258.249978738764,19.6997697122226)) ;
#104901=CARTESIAN_POINT('Ctrl Pts',(38.8400591218529,258.25,19.7001827000972)) ;
#104902=CARTESIAN_POINT('Ctrl Pts',(38.8386601166805,258.25,19.7005955910407)) ;
#104903=CARTESIAN_POINT('Origin',(40.2,258.1,25.0213203435596)) ;
#104904=CARTESIAN_POINT('Ctrl Pts',(39.8505167960037,258.25,20.0836729796702)) ;
#104905=CARTESIAN_POINT('Ctrl Pts',(39.8499397253391,258.25,20.0831353099888)) ;
#104906=CARTESIAN_POINT('Ctrl Pts',(39.8493626067619,258.249996669894,20.0825976834901)) ;
#104907=CARTESIAN_POINT('Ctrl Pts',(39.8339123904255,258.249818328848,20.0682070710063)) ;
#104908=CARTESIAN_POINT('Ctrl Pts',(39.8189533892408,258.247433157512,20.0543335974202)) ;
#104909=CARTESIAN_POINT('Ctrl Pts',(39.7905380911743,258.238259809032,20.0280856875442)) ;
#104910=CARTESIAN_POINT('Ctrl Pts',(39.7769188845308,258.231622782802,20.0155562650352)) ;
#104911=CARTESIAN_POINT('Ctrl Pts',(39.7501412146257,258.21278678422,19.9910035412763)) ;
#104912=CARTESIAN_POINT('Ctrl Pts',(39.7370754538178,258.199976451841,19.9790753854857)) ;
#104913=CARTESIAN_POINT('Ctrl Pts',(39.7180779384581,258.171958342729,19.9617756192428)) ;
#104914=CARTESIAN_POINT('Ctrl Pts',(39.7112763996935,258.158041775475,19.9555988579533)) ;
#104915=CARTESIAN_POINT('Ctrl Pts',(39.7026699639648,258.129045309865,19.9477891624225)) ;
#104916=CARTESIAN_POINT('Ctrl Pts',(39.7005167960037,258.114679223254,19.9458384424072)) ;
#104917=CARTESIAN_POINT('Ctrl Pts',(39.7005167960037,258.1,19.9458384424072)) ;
#104918=CARTESIAN_POINT('Origin',(39.8505167960037,258.1,22.6343496415544)) ;
#104919=CARTESIAN_POINT('Ctrl Pts',(39.8505167960037,258.25,19.5403332371979)) ;
#104920=CARTESIAN_POINT('Ctrl Pts',(39.8490586726999,258.25,19.5403728709491)) ;
#104921=CARTESIAN_POINT('Ctrl Pts',(39.8476006233589,258.249978738764,19.5404123787479)) ;
#104922=CARTESIAN_POINT('Ctrl Pts',(39.8461431129253,258.249936222763,19.540451750423)) ;
#104923=CARTESIAN_POINT('Ctrl Pts',(39.8274188890355,258.249390031724,19.5409575471857)) ;
#104924=CARTESIAN_POINT('Ctrl Pts',(39.8089607261725,258.245341162533,19.5414357612546)) ;
#104925=CARTESIAN_POINT('Ctrl Pts',(39.7917256812165,258.237998568189,19.5418692158132)) ;
#104926=CARTESIAN_POINT('Ctrl Pts',(39.773758167714,258.230343922473,19.5423210916658)) ;
#104927=CARTESIAN_POINT('Ctrl Pts',(39.757456249043,258.21925289602,19.5427162141691)) ;
#104928=CARTESIAN_POINT('Ctrl Pts',(39.7437381135436,258.205348530944,19.5430425837128)) ;
#104929=CARTESIAN_POINT('Ctrl Pts',(39.7300236484415,258.191447886093,19.5433688659337)) ;
#104930=CARTESIAN_POINT('Ctrl Pts',(39.7191539711575,258.175001311387,19.5436204501225)) ;
#104931=CARTESIAN_POINT('Ctrl Pts',(39.7117415393001,258.156933541317,19.5437909270115)) ;
#104932=CARTESIAN_POINT('Ctrl Pts',(39.704330020872,258.138867997726,19.5439613828928)) ;
#104933=CARTESIAN_POINT('Ctrl Pts',(39.7005167960037,258.119527473902,19.5440476162869)) ;
#104934=CARTESIAN_POINT('Ctrl Pts',(39.7005167960037,258.1,19.5440476162869)) ;
#104935=CARTESIAN_POINT('Origin',(41.3786634562732,258.1,22.5247186334439)) ;
#104936=CARTESIAN_POINT('Ctrl Pts',(42.3676071114945,258.1,19.9664732232005)) ;
#104937=CARTESIAN_POINT('Ctrl Pts',(42.3676071114945,258.119527473902,19.9664732232005)) ;
#104938=CARTESIAN_POINT('Ctrl Pts',(42.3640071667196,258.138867997726,19.9652128590816)) ;
#104939=CARTESIAN_POINT('Ctrl Pts',(42.357011067587,258.156933541317,19.9627604607565)) ;
#104940=CARTESIAN_POINT('Ctrl Pts',(42.3500141062233,258.175001311387,19.9603077601868)) ;
#104941=CARTESIAN_POINT('Ctrl Pts',(42.3397541726022,258.191447886093,19.9567095744005)) ;
#104942=CARTESIAN_POINT('Ctrl Pts',(42.3268117679506,258.205348530944,19.9521612587828)) ;
#104943=CARTESIAN_POINT('Ctrl Pts',(42.3138658995279,258.21925289602,19.9476117259012)) ;
#104944=CARTESIAN_POINT('Ctrl Pts',(42.2984839531161,258.230343922473,19.9421983721593)) ;
#104945=CARTESIAN_POINT('Ctrl Pts',(42.2815354696358,258.237998568189,19.9362163456661)) ;
#104946=CARTESIAN_POINT('Ctrl Pts',(42.2652779126467,258.245341162533,19.9304781840933)) ;
#104947=CARTESIAN_POINT('Ctrl Pts',(42.2478709328508,258.249390031724,19.9243194894782)) ;
#104948=CARTESIAN_POINT('Ctrl Pts',(42.2302194375034,258.249936222763,19.9180523447823)) ;
#104949=CARTESIAN_POINT('Ctrl Pts',(42.2288454292246,258.249978738764,19.9175645046006)) ;
#104950=CARTESIAN_POINT('Ctrl Pts',(42.2274709504794,258.25,19.9170763684254)) ;
#104951=CARTESIAN_POINT('Ctrl Pts',(42.2260964403124,258.25,19.9165880896073)) ;
#104952=CARTESIAN_POINT('Ctrl Pts',(42.0581952261685,258.25,20.4333348922483)) ;
#104953=CARTESIAN_POINT('Ctrl Pts',(42.0589102020544,258.25,20.433001862636)) ;
#104954=CARTESIAN_POINT('Ctrl Pts',(42.0596252101647,258.249996669894,20.4326688888986)) ;
#104955=CARTESIAN_POINT('Ctrl Pts',(42.0787661829066,258.249818328848,20.423756982537)) ;
#104956=CARTESIAN_POINT('Ctrl Pts',(42.0972801775694,258.247433157512,20.4151851106646)) ;
#104957=CARTESIAN_POINT('Ctrl Pts',(42.1324157821755,258.238259809031,20.3990026749411)) ;
#104958=CARTESIAN_POINT('Ctrl Pts',(42.1492402218848,258.231622782802,20.3912950523216)) ;
#104959=CARTESIAN_POINT('Ctrl Pts',(42.1822945082381,258.21278678422,20.3762187794687)) ;
#104960=CARTESIAN_POINT('Ctrl Pts',(42.1984067880458,258.199976451841,20.3689119713107)) ;
#104961=CARTESIAN_POINT('Ctrl Pts',(42.2218204205898,258.171958342729,20.3583294709921)) ;
#104962=CARTESIAN_POINT('Ctrl Pts',(42.2301977925614,258.158041775475,20.3545568129842)) ;
#104963=CARTESIAN_POINT('Ctrl Pts',(42.2407963279832,258.129045309865,20.3497888860605)) ;
#104964=CARTESIAN_POINT('Ctrl Pts',(42.2434469180392,258.114679223254,20.3485990065702)) ;
#104965=CARTESIAN_POINT('Ctrl Pts',(42.2434469180392,258.1,20.3485990065702)) ;
#104966=CARTESIAN_POINT('Origin',(40.5494832039963,258.1,22.2826839799233)) ;
#104967=CARTESIAN_POINT('Ctrl Pts',(40.5494832039963,258.25,20.0836729796702)) ;
#104968=CARTESIAN_POINT('Ctrl Pts',(40.5500602746609,258.25,20.0831353099888)) ;
#104969=CARTESIAN_POINT('Ctrl Pts',(40.5506373932381,258.249996669894,20.0825976834901)) ;
#104970=CARTESIAN_POINT('Ctrl Pts',(40.5660876095746,258.249818328848,20.0682070710062)) ;
#104971=CARTESIAN_POINT('Ctrl Pts',(40.5810466107592,258.247433157512,20.0543335974202)) ;
#104972=CARTESIAN_POINT('Ctrl Pts',(40.6094619088255,258.238259809032,20.0280856875444)) ;
#104973=CARTESIAN_POINT('Ctrl Pts',(40.6230811154692,258.231622782802,20.0155562650353)) ;
#104974=CARTESIAN_POINT('Ctrl Pts',(40.6498587853742,258.21278678422,19.9910035412764)) ;
#104975=CARTESIAN_POINT('Ctrl Pts',(40.6629245461822,258.199976451841,19.9790753854858)) ;
#104976=CARTESIAN_POINT('Ctrl Pts',(40.681922061542,258.171958342729,19.9617756192429)) ;
#104977=CARTESIAN_POINT('Ctrl Pts',(40.6887236003065,258.158041775475,19.9555988579533)) ;
#104978=CARTESIAN_POINT('Ctrl Pts',(40.6973300360353,258.129045309865,19.9477891624225)) ;
#104979=CARTESIAN_POINT('Ctrl Pts',(40.6994832039963,258.114679223254,19.9458384424072)) ;
#104980=CARTESIAN_POINT('Ctrl Pts',(40.6994832039963,258.1,19.9458384424072)) ;
#104981=CARTESIAN_POINT('Ctrl Pts',(40.6994832039963,258.1,19.5440476162867)) ;
#104982=CARTESIAN_POINT('Ctrl Pts',(40.6994832039963,258.119527473902,19.5440476162867)) ;
#104983=CARTESIAN_POINT('Ctrl Pts',(40.695669979128,258.138867997726,19.5439613828925)) ;
#104984=CARTESIAN_POINT('Ctrl Pts',(40.6882584606999,258.156933541317,19.5437909270112)) ;
#104985=CARTESIAN_POINT('Ctrl Pts',(40.6808460288425,258.175001311387,19.5436204501222)) ;
#104986=CARTESIAN_POINT('Ctrl Pts',(40.6699763515586,258.191447886093,19.5433688659334)) ;
#104987=CARTESIAN_POINT('Ctrl Pts',(40.6562618864565,258.205348530944,19.5430425837125)) ;
#104988=CARTESIAN_POINT('Ctrl Pts',(40.642543750957,258.21925289602,19.5427162141689)) ;
#104989=CARTESIAN_POINT('Ctrl Pts',(40.626241832286,258.230343922473,19.5423210916655)) ;
#104990=CARTESIAN_POINT('Ctrl Pts',(40.6082743187836,258.237998568189,19.5418692158129)) ;
#104991=CARTESIAN_POINT('Ctrl Pts',(40.5910392738275,258.245341162533,19.5414357612543)) ;
#104992=CARTESIAN_POINT('Ctrl Pts',(40.5725811109643,258.249390031724,19.5409575471862)) ;
#104993=CARTESIAN_POINT('Ctrl Pts',(40.5538568870747,258.249936222763,19.5404517504227)) ;
#104994=CARTESIAN_POINT('Ctrl Pts',(40.5523993766411,258.249978738764,19.5404123787476)) ;
#104995=CARTESIAN_POINT('Ctrl Pts',(40.5509413273001,258.25,19.5403728709489)) ;
#104996=CARTESIAN_POINT('Ctrl Pts',(40.5494832039963,258.25,19.5403332371977)) ;
#104997=CARTESIAN_POINT('Origin',(40.2,258.1,25.0213203435596)) ;
#104998=CARTESIAN_POINT('Ctrl Pts',(41.3934386691762,258.25,20.2173423936815)) ;
#104999=CARTESIAN_POINT('Ctrl Pts',(41.3930559914298,258.25,20.2166527147863)) ;
#105000=CARTESIAN_POINT('Ctrl Pts',(41.3926732547717,258.249996669894,20.2159630621546)) ;
#105001=CARTESIAN_POINT('Ctrl Pts',(41.3824261696639,258.249818328848,20.1975023969641)) ;
#105002=CARTESIAN_POINT('Ctrl Pts',(41.3724864532189,258.247433157513,20.1796853539209)) ;
#105003=CARTESIAN_POINT('Ctrl Pts',(41.353572949048,258.238259809032,20.1459412981901)) ;
#105004=CARTESIAN_POINT('Ctrl Pts',(41.3444921183075,258.231622782802,20.1298165429642)) ;
#105005=CARTESIAN_POINT('Ctrl Pts',(41.3266122497526,258.21278678422,20.0981907599697)) ;
#105006=CARTESIAN_POINT('Ctrl Pts',(41.3178719756467,258.199976451841,20.0828088675435)) ;
#105007=CARTESIAN_POINT('Ctrl Pts',(41.3051501866382,258.171958342729,20.0604852570307)) ;
#105008=CARTESIAN_POINT('Ctrl Pts',(41.3005902630839,258.158041775475,20.0525090168905)) ;
#105009=CARTESIAN_POINT('Ctrl Pts',(41.294818384942,258.129045309865,20.0424220201645)) ;
#105010=CARTESIAN_POINT('Ctrl Pts',(41.2933734061579,258.114679223254,20.0399014096908)) ;
#105011=CARTESIAN_POINT('Ctrl Pts',(41.2933734061579,258.1,20.0399014096908)) ;
#105012=CARTESIAN_POINT('Origin',(40.6052362334984,258.1,22.6431800539285)) ;
#105013=CARTESIAN_POINT('Ctrl Pts',(41.5613398833194,258.25,19.700595591041)) ;
#105014=CARTESIAN_POINT('Ctrl Pts',(41.559940878147,258.25,19.7001827000975)) ;
#105015=CARTESIAN_POINT('Ctrl Pts',(41.5585419822389,258.249978738764,19.699769712223)) ;
#105016=CARTESIAN_POINT('Ctrl Pts',(41.5571436409267,258.249936222763,19.6993567614174)) ;
#105017=CARTESIAN_POINT('Ctrl Pts',(41.5391795459882,258.249390031724,19.6940516993328)) ;
#105018=CARTESIAN_POINT('Ctrl Pts',(41.5214770136451,258.245341162533,19.6888026219299)) ;
#105019=CARTESIAN_POINT('Ctrl Pts',(41.5049515670062,258.237998568188,19.6838889399227)) ;
#105020=CARTESIAN_POINT('Ctrl Pts',(41.4877238088901,258.230343922473,19.6787664323785)) ;
#105021=CARTESIAN_POINT('Ctrl Pts',(41.4720976633413,258.21925289602,19.6741046463007)) ;
#105022=CARTESIAN_POINT('Ctrl Pts',(41.4589500874477,258.205348530944,19.6701759051814)) ;
#105023=CARTESIAN_POINT('Ctrl Pts',(41.4458060292936,258.191447886093,19.6662482152285)) ;
#105024=CARTESIAN_POINT('Ctrl Pts',(41.4353906080926,258.175001311387,19.6631285710071)) ;
#105025=CARTESIAN_POINT('Ctrl Pts',(41.4282882862172,258.156933541317,19.6610001367497)) ;
#105026=CARTESIAN_POINT('Ctrl Pts',(41.4211868395564,258.138867997726,19.6588719647779)) ;
#105027=CARTESIAN_POINT('Ctrl Pts',(41.4175335996131,258.119527473902,19.6577756263216)) ;
#105028=CARTESIAN_POINT('Ctrl Pts',(41.4175335996131,258.1,19.6577756263216)) ;
#105029=CARTESIAN_POINT('Origin',(41.8995934690622,258.1,19.7905095039363)) ;
#105030=CARTESIAN_POINT('Origin',(40.2,258.1,19.5213203435596)) ;
#105031=CARTESIAN_POINT('Origin',(40.2,258.1,25.0213203435596)) ;
#105032=CARTESIAN_POINT('',(42.7792030093369,258.1,20.6215803698081)) ;
#105033=CARTESIAN_POINT('Origin',(40.2,258.1,25.0213203435596)) ;
#105034=CARTESIAN_POINT('Ctrl Pts',(42.8195384502335,258.25,20.8212586407095)) ;
#105035=CARTESIAN_POINT('Ctrl Pts',(42.8193876245682,258.25,20.8204844631737)) ;
#105036=CARTESIAN_POINT('Ctrl Pts',(42.8192367347586,258.249996669894,20.8197102924112)) ;
#105037=CARTESIAN_POINT('Ctrl Pts',(42.8151958369648,258.249818328848,20.7989866330445)) ;
#105038=CARTESIAN_POINT('Ctrl Pts',(42.8112483739597,258.247433157512,20.7789700768574)) ;
#105039=CARTESIAN_POINT('Ctrl Pts',(42.8036880492523,258.238259809032,20.7410329785579)) ;
#105040=CARTESIAN_POINT('Ctrl Pts',(42.8000344893984,258.231622782802,20.7228912940054)) ;
#105041=CARTESIAN_POINT('Ctrl Pts',(42.7928026283045,258.21278678422,20.6872882037655)) ;
#105042=CARTESIAN_POINT('Ctrl Pts',(42.7892433998272,258.199976451841,20.6699582615064)) ;
#105043=CARTESIAN_POINT('Ctrl Pts',(42.784042634516,258.171958342729,20.6447959972585)) ;
#105044=CARTESIAN_POINT('Ctrl Pts',(42.7821706832604,258.158041775475,20.6358010482263)) ;
#105045=CARTESIAN_POINT('Ctrl Pts',(42.7797983543528,258.129045309865,20.6244241358249)) ;
#105046=CARTESIAN_POINT('Ctrl Pts',(42.7792030093369,258.114679223254,20.6215803698081)) ;
#105047=CARTESIAN_POINT('Ctrl Pts',(42.7792030093369,258.1,20.6215803698081)) ;
#105048=CARTESIAN_POINT('Origin',(41.3202883250113,258.1,22.8847994073294)) ;
#105049=CARTESIAN_POINT('',(43.0153697314369,258.1,20.2965247632928)) ;
#105050=CARTESIAN_POINT('',(41.1989357758551,258.1,22.7966316194855)) ;
#105051=CARTESIAN_POINT('Ctrl Pts',(43.1389055378432,258.25,20.3816875553299)) ;
#105052=CARTESIAN_POINT('Ctrl Pts',(43.137702595176,258.25,20.3808625563341)) ;
#105053=CARTESIAN_POINT('Ctrl Pts',(43.1364997863787,258.249978738764,20.3800374989159)) ;
#105054=CARTESIAN_POINT('Ctrl Pts',(43.1352974935785,258.249936222763,20.3792126481319)) ;
#105055=CARTESIAN_POINT('Ctrl Pts',(43.1198519783687,258.249390031724,20.368616023642)) ;
#105056=CARTESIAN_POINT('Ctrl Pts',(43.1046379237506,258.245341162533,20.3581534710365)) ;
#105057=CARTESIAN_POINT('Ctrl Pts',(43.0904397012851,258.237998568188,20.3483736378934)) ;
#105058=CARTESIAN_POINT('Ctrl Pts',(43.0756380715526,258.230343922473,20.3381781736809)) ;
#105059=CARTESIAN_POINT('Ctrl Pts',(43.0622172951261,258.21925289602,20.3289158071227)) ;
#105060=CARTESIAN_POINT('Ctrl Pts',(43.0509272551714,258.205348530944,20.3211165278944)) ;
#105061=CARTESIAN_POINT('Ctrl Pts',(43.0396402359575,258.191447886093,20.3133193354259)) ;
#105062=CARTESIAN_POINT('Ctrl Pts',(43.0306986048352,258.175001311387,20.3071338353061)) ;
#105063=CARTESIAN_POINT('Ctrl Pts',(43.0246016176917,258.156933541317,20.3029148358772)) ;
#105064=CARTESIAN_POINT('Ctrl Pts',(43.0185053818759,258.138867997726,20.2986963563528)) ;
#105065=CARTESIAN_POINT('Ctrl Pts',(43.0153697314369,258.119527473902,20.2965247632927)) ;
#105066=CARTESIAN_POINT('Ctrl Pts',(43.0153697314369,258.1,20.2965247632927)) ;
#105067=CARTESIAN_POINT('Origin',(43.4328188876086,258.1,20.5717268744974)) ;
#105068=CARTESIAN_POINT('Origin',(43.4328188876086,258.1,20.5717268744974)) ;
#105069=CARTESIAN_POINT('Origin',(38.5004065309378,258.1,19.7905095039363)) ;
#105070=CARTESIAN_POINT('Origin',(40.2,258.1,25.0213203435596)) ;
#105071=CARTESIAN_POINT('',(44.012562251598,258.1,21.6339365333471)) ;
#105072=CARTESIAN_POINT('Origin',(40.2,258.1,25.0213203435596)) ;
#105073=CARTESIAN_POINT('Ctrl Pts',(43.9892195563843,258.25,21.836306190763)) ;
#105074=CARTESIAN_POINT('Ctrl Pts',(43.9893153466675,258.25,21.8355232964805)) ;
#105075=CARTESIAN_POINT('Ctrl Pts',(43.9894110738529,258.249996669894,21.8347403888179)) ;
#105076=CARTESIAN_POINT('Ctrl Pts',(43.9919719146049,258.249818328848,21.8137823114479)) ;
#105077=CARTESIAN_POINT('Ctrl Pts',(43.9944031102213,258.247433157513,21.7935256020966)) ;
#105078=CARTESIAN_POINT('Ctrl Pts',(43.998936022235,258.238259809032,21.7551090087302)) ;
#105079=CARTESIAN_POINT('Ctrl Pts',(44.0010673691616,258.231622782802,21.7367262293345)) ;
#105080=CARTESIAN_POINT('Ctrl Pts',(44.0051914204798,258.21278678422,21.7006309103821)) ;
#105081=CARTESIAN_POINT('Ctrl Pts',(44.007161639713,258.199976451842,21.6830492937831)) ;
#105082=CARTESIAN_POINT('Ctrl Pts',(44.0099909852436,258.171958342729,21.6575114335403)) ;
#105083=CARTESIAN_POINT('Ctrl Pts',(44.0109902459184,258.158041775475,21.648378263899)) ;
#105084=CARTESIAN_POINT('Ctrl Pts',(44.0122496863275,258.129045309865,21.6368250872756)) ;
#105085=CARTESIAN_POINT('Ctrl Pts',(44.012562251598,258.114679223254,21.6339365333471)) ;
#105086=CARTESIAN_POINT('Ctrl Pts',(44.012562251598,258.1,21.6339365333471)) ;
#105087=CARTESIAN_POINT('Origin',(41.9256787897644,258.1,23.3355563159851)) ;
#105088=CARTESIAN_POINT('',(44.3376178581133,258.1,21.3977698112471)) ;
#105089=CARTESIAN_POINT('',(41.8375110019206,258.1,23.2142037668289)) ;
#105090=CARTESIAN_POINT('Ctrl Pts',(44.428790641764,258.25,21.5169391031532)) ;
#105091=CARTESIAN_POINT('Ctrl Pts',(44.4279015140119,258.25,21.5157827527552)) ;
#105092=CARTESIAN_POINT('Ctrl Pts',(44.4270125316316,258.249978738765,21.5146263881606)) ;
#105093=CARTESIAN_POINT('Ctrl Pts',(44.426123976139,258.249936222763,21.5134703795409)) ;
#105094=CARTESIAN_POINT('Ctrl Pts',(44.4147089552931,258.249390031725,21.4986194640922)) ;
#105095=CARTESIAN_POINT('Ctrl Pts',(44.4034726360758,258.245341162534,21.4839675838213)) ;
#105096=CARTESIAN_POINT('Ctrl Pts',(44.3929914587233,258.237998568189,21.4702789177501)) ;
#105097=CARTESIAN_POINT('Ctrl Pts',(44.3820648440218,258.230343922473,21.4560084999423)) ;
#105098=CARTESIAN_POINT('Ctrl Pts',(44.3721631558235,258.21925289602,21.4430522178764)) ;
#105099=CARTESIAN_POINT('Ctrl Pts',(44.3638357995807,258.205348530944,21.4321458483306)) ;
#105100=CARTESIAN_POINT('Ctrl Pts',(44.355510671389,258.191447886093,21.4212423968717)) ;
#105101=CARTESIAN_POINT('Ctrl Pts',(44.3489180994998,258.175001311387,21.4125965207017)) ;
#105102=CARTESIAN_POINT('Ctrl Pts',(44.3444232626702,258.156933541317,21.4066999411606)) ;
#105103=CARTESIAN_POINT('Ctrl Pts',(44.3399289797364,258.138867997726,21.4008040882511)) ;
#105104=CARTESIAN_POINT('Ctrl Pts',(44.3376178581132,258.119527473902,21.3977698112471)) ;
#105105=CARTESIAN_POINT('Ctrl Pts',(44.3376178581134,258.1,21.397769811247)) ;
#105106=CARTESIAN_POINT('Origin',(44.6495934690622,258.1,21.788501455951)) ;
#105107=CARTESIAN_POINT('Origin',(44.6495934690622,258.1,21.788501455951)) ;
#105108=CARTESIAN_POINT('Origin',(36.9671811123914,258.1,20.5717268744974)) ;
#105109=CARTESIAN_POINT('Origin',(40.2,258.1,25.0213203435596)) ;
#105110=CARTESIAN_POINT('',(44.8727213369894,258.1,22.9778734255204)) ;
#105111=CARTESIAN_POINT('Origin',(40.2,258.1,25.0213203435596)) ;
#105112=CARTESIAN_POINT('Ctrl Pts',(44.7879854513112,258.25,23.1631251173908)) ;
#105113=CARTESIAN_POINT('Ctrl Pts',(44.788318480923,258.25,23.162410141506)) ;
#105114=CARTESIAN_POINT('Ctrl Pts',(44.7886514546598,258.249996669894,23.1616951333976)) ;
#105115=CARTESIAN_POINT('Ctrl Pts',(44.7975633610212,258.249818328848,23.1425541606572)) ;
#105116=CARTESIAN_POINT('Ctrl Pts',(44.8061352328939,258.247433157512,23.1240401659929)) ;
#105117=CARTESIAN_POINT('Ctrl Pts',(44.8223176686178,258.238259809032,23.0889045613858)) ;
#105118=CARTESIAN_POINT('Ctrl Pts',(44.8300252912377,258.231622782802,23.0720801216756)) ;
#105119=CARTESIAN_POINT('Ctrl Pts',(44.845101564091,258.21278678422,23.0390258353215)) ;
#105120=CARTESIAN_POINT('Ctrl Pts',(44.8524083722489,258.199976451841,23.0229135555138)) ;
#105121=CARTESIAN_POINT('Ctrl Pts',(44.8629908725676,258.171958342729,22.9994999229698)) ;
#105122=CARTESIAN_POINT('Ctrl Pts',(44.8667635305755,258.158041775475,22.9911225509982)) ;
#105123=CARTESIAN_POINT('Ctrl Pts',(44.8715314574991,258.129045309865,22.9805240155764)) ;
#105124=CARTESIAN_POINT('Ctrl Pts',(44.8727213369894,258.114679223254,22.9778734255204)) ;
#105125=CARTESIAN_POINT('Ctrl Pts',(44.8727213369894,258.1,22.9778734255204)) ;
#105126=CARTESIAN_POINT('Origin',(42.3621477910643,258.1,23.9513275530686)) ;
#105127=CARTESIAN_POINT('',(45.2548471203588,258.1,22.8537132320653)) ;
#105128=CARTESIAN_POINT('',(42.315795241908,258.1,23.8086690756243)) ;
#105129=CARTESIAN_POINT('Ctrl Pts',(45.3047322539521,258.25,22.9952239032473)) ;
#105130=CARTESIAN_POINT('Ctrl Pts',(45.3042439751341,258.25,22.9938493930806)) ;
#105131=CARTESIAN_POINT('Ctrl Pts',(45.3037558389596,258.249978738764,22.9924749143347)) ;
#105132=CARTESIAN_POINT('Ctrl Pts',(45.3032679987775,258.249936222763,22.9911009060563)) ;
#105133=CARTESIAN_POINT('Ctrl Pts',(45.2970008540754,258.249390031724,22.9734494107125)) ;
#105134=CARTESIAN_POINT('Ctrl Pts',(45.2908421594689,258.245341162533,22.9560424309124)) ;
#105135=CARTESIAN_POINT('Ctrl Pts',(45.2851039978952,258.237998568188,22.9397848739232)) ;
#105136=CARTESIAN_POINT('Ctrl Pts',(45.2791219714012,258.230343922473,22.9228363904432)) ;
#105137=CARTESIAN_POINT('Ctrl Pts',(45.2737086176589,258.21925289602,22.9074544440317)) ;
#105138=CARTESIAN_POINT('Ctrl Pts',(45.2691590847773,258.205348530944,22.8945085756089)) ;
#105139=CARTESIAN_POINT('Ctrl Pts',(45.2646107691597,258.191447886093,22.8815661709572)) ;
#105140=CARTESIAN_POINT('Ctrl Pts',(45.2610125833727,258.175001311387,22.8713062373364)) ;
#105141=CARTESIAN_POINT('Ctrl Pts',(45.2585598828031,258.156933541317,22.8643092759727)) ;
#105142=CARTESIAN_POINT('Ctrl Pts',(45.2561074844783,258.138867997726,22.85731317684)) ;
#105143=CARTESIAN_POINT('Ctrl Pts',(45.2548471203588,258.119527473902,22.8537132320654)) ;
#105144=CARTESIAN_POINT('Ctrl Pts',(45.254847120359,258.1,22.8537132320653)) ;
#105145=CARTESIAN_POINT('Origin',(45.4308108396234,258.1,23.3217268744974)) ;
#105146=CARTESIAN_POINT('Origin',(45.4308108396234,258.1,23.3217268744974)) ;
#105147=CARTESIAN_POINT('Origin',(35.7504065309378,258.1,21.788501455951)) ;
#105148=CARTESIAN_POINT('Origin',(40.2,258.1,25.0213203435596)) ;
#105149=CARTESIAN_POINT('',(45.2754819011524,258.1,24.5218371395634)) ;
#105150=CARTESIAN_POINT('Origin',(40.2,258.1,25.0213203435596)) ;
#105151=CARTESIAN_POINT('Ctrl Pts',(45.1376473638895,258.25,24.6718371395634)) ;
#105152=CARTESIAN_POINT('Ctrl Pts',(45.1381850335709,258.25,24.6712600688988)) ;
#105153=CARTESIAN_POINT('Ctrl Pts',(45.1387226600695,258.249996669894,24.6706829503216)) ;
#105154=CARTESIAN_POINT('Ctrl Pts',(45.1531132725535,258.249818328848,24.655232733985)) ;
#105155=CARTESIAN_POINT('Ctrl Pts',(45.1669867461395,258.247433157512,24.6402737328004)) ;
#105156=CARTESIAN_POINT('Ctrl Pts',(45.1932346560154,258.238259809032,24.611858434734)) ;
#105157=CARTESIAN_POINT('Ctrl Pts',(45.2057640785244,258.231622782802,24.5982392280904)) ;
#105158=CARTESIAN_POINT('Ctrl Pts',(45.2303168022832,258.21278678422,24.5714615581854)) ;
#105159=CARTESIAN_POINT('Ctrl Pts',(45.2422449580739,258.199976451841,24.5583957973774)) ;
#105160=CARTESIAN_POINT('Ctrl Pts',(45.2595447243168,258.171958342729,24.5393982820176)) ;
#105161=CARTESIAN_POINT('Ctrl Pts',(45.2657214856064,258.158041775475,24.5325967432531)) ;
#105162=CARTESIAN_POINT('Ctrl Pts',(45.2735311811371,258.129045309865,24.5239903075244)) ;
#105163=CARTESIAN_POINT('Ctrl Pts',(45.2754819011524,258.114679223254,24.5218371395634)) ;
#105164=CARTESIAN_POINT('Ctrl Pts',(45.2754819011524,258.1,24.5218371395634)) ;
#105165=CARTESIAN_POINT('Origin',(42.5869707020053,258.1,24.6718371395634)) ;
#105166=CARTESIAN_POINT('',(45.6772727272728,258.1,24.5218371395634)) ;
#105167=CARTESIAN_POINT('',(42.5869707020053,258.1,24.5218371395634)) ;
#105168=CARTESIAN_POINT('Ctrl Pts',(45.6809871063617,258.25,24.6718371395634)) ;
#105169=CARTESIAN_POINT('Ctrl Pts',(45.6809474726105,258.25,24.6703790162596)) ;
#105170=CARTESIAN_POINT('Ctrl Pts',(45.6809079648117,258.249978738764,24.6689209669186)) ;
#105171=CARTESIAN_POINT('Ctrl Pts',(45.6808685931366,258.249936222763,24.667463456485)) ;
#105172=CARTESIAN_POINT('Ctrl Pts',(45.6803627963739,258.249390031724,24.6487392325953)) ;
#105173=CARTESIAN_POINT('Ctrl Pts',(45.6798845823058,258.245341162533,24.6302810697322)) ;
#105174=CARTESIAN_POINT('Ctrl Pts',(45.6794511277471,258.237998568189,24.6130460247761)) ;
#105175=CARTESIAN_POINT('Ctrl Pts',(45.6789992518944,258.230343922473,24.5950785112736)) ;
#105176=CARTESIAN_POINT('Ctrl Pts',(45.678604129391,258.21925289602,24.5787765926027)) ;
#105177=CARTESIAN_POINT('Ctrl Pts',(45.6782777598474,258.205348530944,24.5650584571032)) ;
#105178=CARTESIAN_POINT('Ctrl Pts',(45.6779514776265,258.191447886093,24.5513439920011)) ;
#105179=CARTESIAN_POINT('Ctrl Pts',(45.6776998934372,258.175001311387,24.5404743147172)) ;
#105180=CARTESIAN_POINT('Ctrl Pts',(45.6775294165482,258.156933541317,24.5330618828598)) ;
#105181=CARTESIAN_POINT('Ctrl Pts',(45.6773589606669,258.138867997726,24.5256503644317)) ;
#105182=CARTESIAN_POINT('Ctrl Pts',(45.6772727272727,258.119527473902,24.5218371395634)) ;
#105183=CARTESIAN_POINT('Ctrl Pts',(45.6772727272727,258.1,24.5218371395634)) ;
#105184=CARTESIAN_POINT('Origin',(45.7,258.1,25.0213203435596)) ;
#105185=CARTESIAN_POINT('Origin',(45.7,258.1,25.0213203435596)) ;
#105186=CARTESIAN_POINT('Origin',(34.9691891603767,258.1,23.3217268744974)) ;
#105187=CARTESIAN_POINT('Origin',(40.2,258.1,25.0213203435596)) ;
#105188=CARTESIAN_POINT('',(45.1814189338688,258.1,26.1146937497175)) ;
#105189=CARTESIAN_POINT('Origin',(40.2,258.1,25.0213203435596)) ;
#105190=CARTESIAN_POINT('Ctrl Pts',(45.0039779498781,258.25,26.2147590127358)) ;
#105191=CARTESIAN_POINT('Ctrl Pts',(45.0046676287764,258.25,26.2143763349877)) ;
#105192=CARTESIAN_POINT('Ctrl Pts',(45.0053572814057,258.249996669895,26.213993598331)) ;
#105193=CARTESIAN_POINT('Ctrl Pts',(45.0238179465998,258.249818328848,26.2037465132206)) ;
#105194=CARTESIAN_POINT('Ctrl Pts',(45.0416349896415,258.247433157512,26.1938067967769)) ;
#105195=CARTESIAN_POINT('Ctrl Pts',(45.0753790453709,258.238259809032,26.1748932926068)) ;
#105196=CARTESIAN_POINT('Ctrl Pts',(45.0915038005962,258.231622782802,26.1658124618668)) ;
#105197=CARTESIAN_POINT('Ctrl Pts',(45.1231295835901,258.21278678422,26.1479325933121)) ;
#105198=CARTESIAN_POINT('Ctrl Pts',(45.1385114760162,258.199976451841,26.1391923192062)) ;
#105199=CARTESIAN_POINT('Ctrl Pts',(45.1608350865289,258.171958342729,26.1264705301978)) ;
#105200=CARTESIAN_POINT('Ctrl Pts',(45.1688113266691,258.158041775475,26.1219106066435)) ;
#105201=CARTESIAN_POINT('Ctrl Pts',(45.1788983233951,258.129045309865,26.1161387285016)) ;
#105202=CARTESIAN_POINT('Ctrl Pts',(45.1814189338688,258.114679223254,26.1146937497175)) ;
#105203=CARTESIAN_POINT('Ctrl Pts',(45.1814189338688,258.1,26.1146937497175)) ;
#105204=CARTESIAN_POINT('Origin',(42.5781402896312,258.1,25.426556577058)) ;
#105205=CARTESIAN_POINT('',(45.5635447172382,258.1,26.2388539431727)) ;
#105206=CARTESIAN_POINT('',(42.6244928387874,258.1,25.2838980996137)) ;
#105207=CARTESIAN_POINT('Ctrl Pts',(45.5207247525189,258.25,26.3826602268791)) ;
#105208=CARTESIAN_POINT('Ctrl Pts',(45.5211376434625,258.25,26.3812612217063)) ;
#105209=CARTESIAN_POINT('Ctrl Pts',(45.5215506313345,258.249978738764,26.3798623257983)) ;
#105210=CARTESIAN_POINT('Ctrl Pts',(45.5219635821412,258.249936222763,26.3784639844859)) ;
#105211=CARTESIAN_POINT('Ctrl Pts',(45.527268644238,258.249390031724,26.3604998895502)) ;
#105212=CARTESIAN_POINT('Ctrl Pts',(45.5325177216272,258.245341162533,26.3427973572038)) ;
#105213=CARTESIAN_POINT('Ctrl Pts',(45.5374314036352,258.237998568189,26.3262719105652)) ;
#105214=CARTESIAN_POINT('Ctrl Pts',(45.5425539111803,258.230343922473,26.3090441524495)) ;
#105215=CARTESIAN_POINT('Ctrl Pts',(45.5472156972587,258.21925289602,26.2934180069008)) ;
#105216=CARTESIAN_POINT('Ctrl Pts',(45.551144438378,258.205348530944,26.2802704310072)) ;
#105217=CARTESIAN_POINT('Ctrl Pts',(45.5550721283311,258.191447886093,26.2671263728531)) ;
#105218=CARTESIAN_POINT('Ctrl Pts',(45.5581917725533,258.175001311387,26.2567109516524)) ;
#105219=CARTESIAN_POINT('Ctrl Pts',(45.5603202068105,258.156933541317,26.249608629777)) ;
#105220=CARTESIAN_POINT('Ctrl Pts',(45.5624483787821,258.138867997726,26.2425071831161)) ;
#105221=CARTESIAN_POINT('Ctrl Pts',(45.5635447172386,258.119527473902,26.2388539431728)) ;
#105222=CARTESIAN_POINT('Ctrl Pts',(45.5635447172384,258.1,26.2388539431728)) ;
#105223=CARTESIAN_POINT('Origin',(45.4308108396234,258.1,26.7209138126218)) ;
#105224=CARTESIAN_POINT('Origin',(45.4308108396234,258.1,26.7209138126218)) ;
#105225=CARTESIAN_POINT('Origin',(34.7,258.1,25.0213203435596)) ;
#105226=CARTESIAN_POINT('Origin',(40.2,258.1,25.0213203435596)) ;
#105227=CARTESIAN_POINT('',(44.5997399737516,258.1,27.6005233528965)) ;
#105228=CARTESIAN_POINT('Origin',(40.2,258.1,25.0213203435596)) ;
#105229=CARTESIAN_POINT('Ctrl Pts',(44.4000617028502,258.25,27.6408587937931)) ;
#105230=CARTESIAN_POINT('Ctrl Pts',(44.400835880388,258.25,27.6407079681274)) ;
#105231=CARTESIAN_POINT('Ctrl Pts',(44.4016100511464,258.249996669895,27.6405570783186)) ;
#105232=CARTESIAN_POINT('Ctrl Pts',(44.4223337105158,258.249818328848,27.6365161805241)) ;
#105233=CARTESIAN_POINT('Ctrl Pts',(44.4423502667025,258.247433157512,27.6325687175193)) ;
#105234=CARTESIAN_POINT('Ctrl Pts',(44.4802873650018,258.238259809032,27.6250083928119)) ;
#105235=CARTESIAN_POINT('Ctrl Pts',(44.4984290495543,258.231622782802,27.621354832958)) ;
#105236=CARTESIAN_POINT('Ctrl Pts',(44.5340321397943,258.21278678422,27.6141229718641)) ;
#105237=CARTESIAN_POINT('Ctrl Pts',(44.5513620820533,258.199976451841,27.6105637433868)) ;
#105238=CARTESIAN_POINT('Ctrl Pts',(44.5765243463011,258.171958342729,27.6053629780756)) ;
#105239=CARTESIAN_POINT('Ctrl Pts',(44.5855192953333,258.158041775475,27.6034910268201)) ;
#105240=CARTESIAN_POINT('Ctrl Pts',(44.5968962077348,258.129045309865,27.6011186979124)) ;
#105241=CARTESIAN_POINT('Ctrl Pts',(44.5997399737516,258.114679223254,27.6005233528965)) ;
#105242=CARTESIAN_POINT('Ctrl Pts',(44.5997399737516,258.1,27.6005233528965)) ;
#105243=CARTESIAN_POINT('Origin',(42.3365209362303,258.1,26.1416086685709)) ;
#105244=CARTESIAN_POINT('',(44.9247955802669,258.1,27.8366900749965)) ;
#105245=CARTESIAN_POINT('',(42.4246887240742,258.1,26.0202561194147)) ;
#105246=CARTESIAN_POINT('Ctrl Pts',(44.8396327882299,258.25,27.9602258814029)) ;
#105247=CARTESIAN_POINT('Ctrl Pts',(44.8404577872258,258.25,27.9590229387355)) ;
#105248=CARTESIAN_POINT('Ctrl Pts',(44.8412828446427,258.249978738764,27.9578201299378)) ;
#105249=CARTESIAN_POINT('Ctrl Pts',(44.8421076954273,258.249936222763,27.9566178371377)) ;
#105250=CARTESIAN_POINT('Ctrl Pts',(44.8527043199227,258.249390031724,27.9411723219305)) ;
#105251=CARTESIAN_POINT('Ctrl Pts',(44.8631668725218,258.245341162533,27.9259582673091)) ;
#105252=CARTESIAN_POINT('Ctrl Pts',(44.8729467056653,258.237998568189,27.911760044844)) ;
#105253=CARTESIAN_POINT('Ctrl Pts',(44.8831421698783,258.230343922473,27.8969584151118)) ;
#105254=CARTESIAN_POINT('Ctrl Pts',(44.8924045364365,258.21925289602,27.8835376386854)) ;
#105255=CARTESIAN_POINT('Ctrl Pts',(44.9002038156649,258.205348530944,27.8722475987307)) ;
#105256=CARTESIAN_POINT('Ctrl Pts',(44.9080010081334,258.191447886093,27.8609605795169)) ;
#105257=CARTESIAN_POINT('Ctrl Pts',(44.9141865082541,258.175001311387,27.8520189483951)) ;
#105258=CARTESIAN_POINT('Ctrl Pts',(44.918405507683,258.156933541317,27.8459219612516)) ;
#105259=CARTESIAN_POINT('Ctrl Pts',(44.9226239872073,258.138867997726,27.8398257254358)) ;
#105260=CARTESIAN_POINT('Ctrl Pts',(44.9247955802671,258.119527473902,27.8366900749966)) ;
#105261=CARTESIAN_POINT('Ctrl Pts',(44.924795580267,258.1,27.8366900749965)) ;
#105262=CARTESIAN_POINT('Origin',(44.6495934690622,258.1,28.2541392311682)) ;
#105263=CARTESIAN_POINT('Origin',(44.6495934690622,258.1,28.2541392311682)) ;
#105264=CARTESIAN_POINT('Origin',(34.9691891603767,258.1,26.7209138126218)) ;
#105265=CARTESIAN_POINT('Origin',(40.2,258.1,25.0213203435596)) ;
#105266=CARTESIAN_POINT('',(43.5873838102126,258.1,28.8338825951576)) ;
#105267=CARTESIAN_POINT('Origin',(40.2,258.1,25.0213203435596)) ;
#105268=CARTESIAN_POINT('Ctrl Pts',(43.3850141527966,258.25,28.8105398999439)) ;
#105269=CARTESIAN_POINT('Ctrl Pts',(43.3857970470841,258.25,28.8106356902278)) ;
#105270=CARTESIAN_POINT('Ctrl Pts',(43.3865799547451,258.249996669895,28.810731417413)) ;
#105271=CARTESIAN_POINT('Ctrl Pts',(43.4075380321218,258.249818328848,28.8132922581646)) ;
#105272=CARTESIAN_POINT('Ctrl Pts',(43.4277947414691,258.247433157512,28.8157234537816)) ;
#105273=CARTESIAN_POINT('Ctrl Pts',(43.4662113348325,258.238259809031,28.8202563657949)) ;
#105274=CARTESIAN_POINT('Ctrl Pts',(43.4845941142266,258.231622782802,28.8223877127214)) ;
#105275=CARTESIAN_POINT('Ctrl Pts',(43.5206894331777,258.21278678422,28.8265117640394)) ;
#105276=CARTESIAN_POINT('Ctrl Pts',(43.5382710497767,258.199976451841,28.8284819832727)) ;
#105277=CARTESIAN_POINT('Ctrl Pts',(43.5638089100193,258.171958342729,28.8313113288033)) ;
#105278=CARTESIAN_POINT('Ctrl Pts',(43.5729420796607,258.158041775475,28.832310589478)) ;
#105279=CARTESIAN_POINT('Ctrl Pts',(43.584495256284,258.129045309865,28.8335700298871)) ;
#105280=CARTESIAN_POINT('Ctrl Pts',(43.5873838102126,258.114679223254,28.8338825951576)) ;
#105281=CARTESIAN_POINT('Ctrl Pts',(43.5873838102126,258.1,28.8338825951576)) ;
#105282=CARTESIAN_POINT('Origin',(41.8857640275745,258.1,26.746999133324)) ;
#105283=CARTESIAN_POINT('',(43.8235505323126,258.1,29.1589382016729)) ;
#105284=CARTESIAN_POINT('',(42.0071165767308,258.1,26.6588313454802)) ;
#105285=CARTESIAN_POINT('Ctrl Pts',(43.7043812404062,258.25,29.2501109853232)) ;
#105286=CARTESIAN_POINT('Ctrl Pts',(43.7055375908047,258.25,29.2492218575707)) ;
#105287=CARTESIAN_POINT('Ctrl Pts',(43.7066939553966,258.249978738764,29.2483328751888)) ;
#105288=CARTESIAN_POINT('Ctrl Pts',(43.7078499640179,258.249936222763,29.2474443196972)) ;
#105289=CARTESIAN_POINT('Ctrl Pts',(43.7227008794821,258.249390031724,29.2360292988668)) ;
#105290=CARTESIAN_POINT('Ctrl Pts',(43.737352759739,258.245341162533,29.2247929796352)) ;
#105291=CARTESIAN_POINT('Ctrl Pts',(43.75104142581,258.237998568188,29.2143118022834)) ;
#105292=CARTESIAN_POINT('Ctrl Pts',(43.7653118436182,258.230343922473,29.2033851875822)) ;
#105293=CARTESIAN_POINT('Ctrl Pts',(43.7782681256832,258.21925289602,29.1934834993828)) ;
#105294=CARTESIAN_POINT('Ctrl Pts',(43.7891744952288,258.205348530944,29.18515614314)) ;
#105295=CARTESIAN_POINT('Ctrl Pts',(43.8000779466878,258.191447886093,29.1768310149483)) ;
#105296=CARTESIAN_POINT('Ctrl Pts',(43.808723822858,258.175001311387,29.1702384430595)) ;
#105297=CARTESIAN_POINT('Ctrl Pts',(43.8146204023989,258.156933541317,29.1657436062296)) ;
#105298=CARTESIAN_POINT('Ctrl Pts',(43.8205162553081,258.138867997726,29.1612493232955)) ;
#105299=CARTESIAN_POINT('Ctrl Pts',(43.8235505323127,258.119527473902,29.1589382016731)) ;
#105300=CARTESIAN_POINT('Ctrl Pts',(43.8235505323126,258.1,29.1589382016729)) ;
#105301=CARTESIAN_POINT('Origin',(43.4328188876086,258.1,29.4709138126218)) ;
#105302=CARTESIAN_POINT('Origin',(43.4328188876086,258.1,29.4709138126218)) ;
#105303=CARTESIAN_POINT('Origin',(35.7504065309378,258.1,28.2541392311682)) ;
#105304=CARTESIAN_POINT('Origin',(40.2,258.1,25.0213203435596)) ;
#105305=CARTESIAN_POINT('',(42.2434469180392,258.1,29.694041680549)) ;
#105306=CARTESIAN_POINT('Origin',(40.2,258.1,25.0213203435596)) ;
#105307=CARTESIAN_POINT('Ctrl Pts',(42.0581952261689,258.25,29.6093057948708)) ;
#105308=CARTESIAN_POINT('Ctrl Pts',(42.0589102020537,258.25,29.6096388244826)) ;
#105309=CARTESIAN_POINT('Ctrl Pts',(42.059625210162,258.249996669894,29.6099717982194)) ;
#105310=CARTESIAN_POINT('Ctrl Pts',(42.0787661829036,258.249818328848,29.6188837045809)) ;
#105311=CARTESIAN_POINT('Ctrl Pts',(42.0972801775669,258.247433157512,29.6274555764535)) ;
#105312=CARTESIAN_POINT('Ctrl Pts',(42.1324157821741,258.238259809032,29.6436380121775)) ;
#105313=CARTESIAN_POINT('Ctrl Pts',(42.1492402218842,258.231622782802,29.6513456347974)) ;
#105314=CARTESIAN_POINT('Ctrl Pts',(42.1822945082383,258.21278678422,29.6664219076506)) ;
#105315=CARTESIAN_POINT('Ctrl Pts',(42.1984067880459,258.199976451841,29.6737287158086)) ;
#105316=CARTESIAN_POINT('Ctrl Pts',(42.2218204205899,258.171958342729,29.6843112161272)) ;
#105317=CARTESIAN_POINT('Ctrl Pts',(42.2301977925615,258.158041775475,29.6880838741351)) ;
#105318=CARTESIAN_POINT('Ctrl Pts',(42.2407963279833,258.129045309865,29.6928518010587)) ;
#105319=CARTESIAN_POINT('Ctrl Pts',(42.2434469180392,258.114679223254,29.694041680549)) ;
#105320=CARTESIAN_POINT('Ctrl Pts',(42.2434469180392,258.1,29.694041680549)) ;
#105321=CARTESIAN_POINT('Origin',(41.2699927904911,258.1,27.1834681346239)) ;
#105322=CARTESIAN_POINT('',(42.3676071114944,258.1,30.0761674639184)) ;
#105323=CARTESIAN_POINT('',(41.4126512679354,258.1,27.1371155854676)) ;
#105324=CARTESIAN_POINT('Ctrl Pts',(42.2260964403121,258.25,30.1260525975113)) ;
#105325=CARTESIAN_POINT('Ctrl Pts',(42.2274709504791,258.25,30.1255643186932)) ;
#105326=CARTESIAN_POINT('Ctrl Pts',(42.2288454292248,258.249978738764,30.1250761825189)) ;
#105327=CARTESIAN_POINT('Ctrl Pts',(42.2302194375035,258.249936222763,30.1245883423371)) ;
#105328=CARTESIAN_POINT('Ctrl Pts',(42.24787093285,258.249390031724,30.1183211976397)) ;
#105329=CARTESIAN_POINT('Ctrl Pts',(42.2652779126467,258.245341162533,30.112162503026)) ;
#105330=CARTESIAN_POINT('Ctrl Pts',(42.2815354696359,258.237998568188,30.1064243414531)) ;
#105331=CARTESIAN_POINT('Ctrl Pts',(42.298483953116,258.230343922473,30.1004423149599)) ;
#105332=CARTESIAN_POINT('Ctrl Pts',(42.3138658995278,258.21925289602,30.095028961218)) ;
#105333=CARTESIAN_POINT('Ctrl Pts',(42.3268117679506,258.205348530944,30.0904794283365)) ;
#105334=CARTESIAN_POINT('Ctrl Pts',(42.3397541726023,258.191447886093,30.085931112719)) ;
#105335=CARTESIAN_POINT('Ctrl Pts',(42.3500141062232,258.175001311387,30.0823329269323)) ;
#105336=CARTESIAN_POINT('Ctrl Pts',(42.3570110675869,258.156933541317,30.0798802263626)) ;
#105337=CARTESIAN_POINT('Ctrl Pts',(42.3640071667196,258.138867997726,30.0774278280376)) ;
#105338=CARTESIAN_POINT('Ctrl Pts',(42.3676071114944,258.119527473902,30.0761674639185)) ;
#105339=CARTESIAN_POINT('Ctrl Pts',(42.3676071114944,258.1,30.0761674639186)) ;
#105340=CARTESIAN_POINT('Origin',(41.8995934690622,258.1,30.252131183183)) ;
#105341=CARTESIAN_POINT('Origin',(41.8995934690622,258.1,30.252131183183)) ;
#105342=CARTESIAN_POINT('Origin',(36.9671811123914,258.1,29.4709138126218)) ;
#105343=CARTESIAN_POINT('Origin',(40.2,258.1,25.0213203435596)) ;
#105344=CARTESIAN_POINT('',(40.6994832039963,258.1,30.096802244712)) ;
#105345=CARTESIAN_POINT('Origin',(40.2,258.1,25.0213203435596)) ;
#105346=CARTESIAN_POINT('Ctrl Pts',(40.5494832039963,258.25,29.9589677074491)) ;
#105347=CARTESIAN_POINT('Ctrl Pts',(40.5500602746609,258.25,29.9595053771305)) ;
#105348=CARTESIAN_POINT('Ctrl Pts',(40.5506373932381,258.249996669894,29.9600430036291)) ;
#105349=CARTESIAN_POINT('Ctrl Pts',(40.5660876095745,258.249818328848,29.974433616113)) ;
#105350=CARTESIAN_POINT('Ctrl Pts',(40.5810466107592,258.247433157512,29.9883070896991)) ;
#105351=CARTESIAN_POINT('Ctrl Pts',(40.6094619088257,258.238259809032,30.014554999575)) ;
#105352=CARTESIAN_POINT('Ctrl Pts',(40.6230811154693,258.231622782802,30.027084422084)) ;
#105353=CARTESIAN_POINT('Ctrl Pts',(40.6498587853742,258.21278678422,30.0516371458428)) ;
#105354=CARTESIAN_POINT('Ctrl Pts',(40.6629245461822,258.199976451841,30.0635653016335)) ;
#105355=CARTESIAN_POINT('Ctrl Pts',(40.681922061542,258.171958342729,30.0808650678764)) ;
#105356=CARTESIAN_POINT('Ctrl Pts',(40.6887236003065,258.158041775475,30.087041829166)) ;
#105357=CARTESIAN_POINT('Ctrl Pts',(40.6973300360353,258.129045309865,30.0948515246968)) ;
#105358=CARTESIAN_POINT('Ctrl Pts',(40.6994832039963,258.114679223254,30.096802244712)) ;
#105359=CARTESIAN_POINT('Ctrl Pts',(40.6994832039963,258.1,30.096802244712)) ;
#105360=CARTESIAN_POINT('Origin',(40.5494832039963,258.1,27.4082910455649)) ;
#105361=CARTESIAN_POINT('',(40.6994832039963,258.1,30.4985930708324)) ;
#105362=CARTESIAN_POINT('',(40.6994832039963,258.1,27.4082910455649)) ;
#105363=CARTESIAN_POINT('Ctrl Pts',(40.5494832039963,258.25,30.5023074499214)) ;
#105364=CARTESIAN_POINT('Ctrl Pts',(40.5509413273001,258.25,30.5022678161702)) ;
#105365=CARTESIAN_POINT('Ctrl Pts',(40.5523993766411,258.249978738764,30.5022283083715)) ;
#105366=CARTESIAN_POINT('Ctrl Pts',(40.5538568870747,258.249936222763,30.5021889366964)) ;
#105367=CARTESIAN_POINT('Ctrl Pts',(40.5725811109644,258.249390031724,30.501683139933)) ;
#105368=CARTESIAN_POINT('Ctrl Pts',(40.5910392738276,258.245341162533,30.5012049258673)) ;
#105369=CARTESIAN_POINT('Ctrl Pts',(40.6082743187837,258.237998568188,30.5007714713081)) ;
#105370=CARTESIAN_POINT('Ctrl Pts',(40.6262418322861,258.230343922473,30.5003195954549)) ;
#105371=CARTESIAN_POINT('Ctrl Pts',(40.642543750957,258.21925289602,30.4999244729506)) ;
#105372=CARTESIAN_POINT('Ctrl Pts',(40.6562618864565,258.205348530944,30.499598103407)) ;
#105373=CARTESIAN_POINT('Ctrl Pts',(40.6699763515586,258.191447886093,30.4992718211862)) ;
#105374=CARTESIAN_POINT('Ctrl Pts',(40.6808460288425,258.175001311387,30.4990202369969)) ;
#105375=CARTESIAN_POINT('Ctrl Pts',(40.6882584606999,258.156933541317,30.4988497601079)) ;
#105376=CARTESIAN_POINT('Ctrl Pts',(40.695669979128,258.138867997726,30.4986793042266)) ;
#105377=CARTESIAN_POINT('Ctrl Pts',(40.6994832039963,258.119527473902,30.4985930708323)) ;
#105378=CARTESIAN_POINT('Ctrl Pts',(40.6994832039963,258.1,30.4985930708323)) ;
#105379=CARTESIAN_POINT('Origin',(40.2,258.1,30.5213203435596)) ;
#105380=CARTESIAN_POINT('Origin',(40.2,258.1,30.5213203435596)) ;
#105381=CARTESIAN_POINT('Origin',(38.5004065309378,258.1,30.252131183183)) ;
#105382=CARTESIAN_POINT('Origin',(38.5004065309378,258.1,30.252131183183)) ;
#105383=CARTESIAN_POINT('Origin',(40.2,258.25,25.0213203435596)) ;
#105384=CARTESIAN_POINT('',(39.7005167960037,258.25,30.096802244712)) ;
#105385=CARTESIAN_POINT('',(39.1066265938421,258.25,30.0027392774284)) ;
#105386=CARTESIAN_POINT('Origin',(39.1998077319512,258.25,29.7159572226947)) ;
#105387=CARTESIAN_POINT('',(38.982466400387,258.25,30.3848650607978)) ;
#105388=CARTESIAN_POINT('Origin',(38.5004065309378,258.25,30.252131183183)) ;
#105389=CARTESIAN_POINT('',(38.0323928885057,258.25,30.0761674639184)) ;
#105390=CARTESIAN_POINT('Origin',(38.0323928885057,258.25,30.0761674639184)) ;
#105391=CARTESIAN_POINT('Origin',(42.601961952148,258.25,20.8655317564881)) ;
#105392=CARTESIAN_POINT('',(42.7792030093369,258.25,20.6215803698081)) ;
#105393=CARTESIAN_POINT('',(43.0153697314369,258.25,20.2965247632928)) ;
#105394=CARTESIAN_POINT('Origin',(43.8235505323125,258.25,20.8837024854464)) ;
#105395=CARTESIAN_POINT('',(43.8235505323125,258.25,20.8837024854464)) ;
#105396=CARTESIAN_POINT('',(43.5873838102126,258.25,21.2087580919617)) ;
#105397=CARTESIAN_POINT('Origin',(43.4328188876086,258.25,20.5717268744974)) ;
#105398=CARTESIAN_POINT('Origin',(43.7686108649179,258.25,21.811177590536)) ;
#105399=CARTESIAN_POINT('',(44.012562251598,258.25,21.6339365333471)) ;
#105400=CARTESIAN_POINT('',(44.3376178581133,258.25,21.3977698112471)) ;
#105401=CARTESIAN_POINT('Origin',(44.9247955802669,258.25,22.2059506121228)) ;
#105402=CARTESIAN_POINT('',(44.9247955802669,258.25,22.2059506121228)) ;
#105403=CARTESIAN_POINT('',(44.5997399737516,258.25,22.4421173342227)) ;
#105404=CARTESIAN_POINT('Origin',(44.6495934690622,258.25,21.788501455951)) ;
#105405=CARTESIAN_POINT('Origin',(44.5859392822557,258.25,23.0710545636296)) ;
#105406=CARTESIAN_POINT('',(44.8727213369894,258.25,22.9778734255204)) ;
#105407=CARTESIAN_POINT('',(45.2548471203588,258.25,22.8537132320653)) ;
#105408=CARTESIAN_POINT('Origin',(45.5635447172382,258.25,23.8037867439466)) ;
#105409=CARTESIAN_POINT('',(45.5635447172382,258.25,23.8037867439466)) ;
#105410=CARTESIAN_POINT('',(45.1814189338688,258.25,23.9279469374017)) ;
#105411=CARTESIAN_POINT('Origin',(45.4308108396234,258.25,23.3217268744974)) ;
#105412=CARTESIAN_POINT('Origin',(44.9739414040105,258.25,24.5218371395634)) ;
#105413=CARTESIAN_POINT('',(45.2754819011524,258.25,24.5218371395634)) ;
#105414=CARTESIAN_POINT('',(45.6772727272728,258.25,24.5218371395634)) ;
#105415=CARTESIAN_POINT('Origin',(45.6772727272728,258.25,25.5208035475559)) ;
#105416=CARTESIAN_POINT('',(45.6772727272728,258.25,25.5208035475559)) ;
#105417=CARTESIAN_POINT('',(45.2754819011524,258.25,25.5208035475559)) ;
#105418=CARTESIAN_POINT('Origin',(45.7,258.25,25.0213203435596)) ;
#105419=CARTESIAN_POINT('Origin',(44.8946368791351,258.25,26.0215126116084)) ;
#105420=CARTESIAN_POINT('',(45.1814189338688,258.25,26.1146937497175)) ;
#105421=CARTESIAN_POINT('',(45.5635447172382,258.25,26.2388539431727)) ;
#105422=CARTESIAN_POINT('Origin',(45.2548471203588,258.25,27.188927455054)) ;
#105423=CARTESIAN_POINT('',(45.2548471203588,258.25,27.188927455054)) ;
#105424=CARTESIAN_POINT('',(44.8727213369894,258.25,27.0647672615988)) ;
#105425=CARTESIAN_POINT('Origin',(45.4308108396234,258.25,26.7209138126218)) ;
#105426=CARTESIAN_POINT('Origin',(44.3557885870715,258.25,27.4232822957076)) ;
#105427=CARTESIAN_POINT('',(44.5997399737516,258.25,27.6005233528965)) ;
#105428=CARTESIAN_POINT('',(44.9247955802669,258.25,27.8366900749965)) ;
#105429=CARTESIAN_POINT('Origin',(44.3376178581133,258.25,28.6448708758722)) ;
#105430=CARTESIAN_POINT('',(44.3376178581133,258.25,28.6448708758722)) ;
#105431=CARTESIAN_POINT('',(44.012562251598,258.25,28.4087041537722)) ;
#105432=CARTESIAN_POINT('Origin',(44.6495934690622,258.25,28.2541392311682)) ;
#105433=CARTESIAN_POINT('Origin',(43.4101427530237,258.25,28.5899312084775)) ;
#105434=CARTESIAN_POINT('',(43.5873838102126,258.25,28.8338825951576)) ;
#105435=CARTESIAN_POINT('',(43.8235505323126,258.25,29.1589382016729)) ;
#105436=CARTESIAN_POINT('Origin',(43.0153697314369,258.25,29.7461159238265)) ;
#105437=CARTESIAN_POINT('',(43.0153697314369,258.25,29.7461159238265)) ;
#105438=CARTESIAN_POINT('',(42.7792030093369,258.25,29.4210603173112)) ;
#105439=CARTESIAN_POINT('Origin',(43.4328188876086,258.25,29.4709138126218)) ;
#105440=CARTESIAN_POINT('Origin',(42.1502657799301,258.25,29.4072596258153)) ;
#105441=CARTESIAN_POINT('',(42.2434469180392,258.25,29.694041680549)) ;
#105442=CARTESIAN_POINT('',(42.3676071114944,258.25,30.0761674639184)) ;
#105443=CARTESIAN_POINT('Origin',(41.4175335996131,258.25,30.3848650607978)) ;
#105444=CARTESIAN_POINT('',(41.4175335996131,258.25,30.3848650607978)) ;
#105445=CARTESIAN_POINT('',(41.293373406158,258.25,30.0027392774284)) ;
#105446=CARTESIAN_POINT('Origin',(41.8995934690622,258.25,30.252131183183)) ;
#105447=CARTESIAN_POINT('Origin',(40.6994832039963,258.25,29.7952617475701)) ;
#105448=CARTESIAN_POINT('',(40.6994832039963,258.25,30.096802244712)) ;
#105449=CARTESIAN_POINT('',(40.6994832039963,258.25,30.4985930708324)) ;
#105450=CARTESIAN_POINT('Origin',(39.7005167960037,258.25,30.4985930708324)) ;
#105451=CARTESIAN_POINT('',(39.7005167960037,258.25,30.4985930708324)) ;
#105452=CARTESIAN_POINT('Origin',(40.2,258.25,30.5213203435596)) ;
#105453=CARTESIAN_POINT('Origin',(40.2,258.25,25.0213203435596)) ;
#105454=CARTESIAN_POINT('Origin',(40.2,258.25,25.0213203435596)) ;
#105455=CARTESIAN_POINT('Origin',(40.2,258.25,25.0213203435596)) ;
#105456=CARTESIAN_POINT('Origin',(40.2,258.25,25.0213203435596)) ;
#105457=CARTESIAN_POINT('Origin',(40.2,258.25,25.0213203435596)) ;
#105458=CARTESIAN_POINT('Origin',(40.2,258.25,25.0213203435596)) ;
#105459=CARTESIAN_POINT('Origin',(40.2,258.25,25.0213203435596)) ;
#105460=CARTESIAN_POINT('Origin',(40.2,258.25,25.0213203435596)) ;
#105461=CARTESIAN_POINT('Origin',(40.2,258.25,25.0213203435596)) ;
#105462=CARTESIAN_POINT('Origin',(40.2,258.75,25.0213203435596)) ;
#105463=CARTESIAN_POINT('',(42.2,258.75,25.0213203435596)) ;
#117144=UNCERTAINTY_MEASURE_WITH_UNIT(LENGTH_MEASURE(0.01),#117171,
'DISTANCE_ACCURACY_VALUE',
'Maximum model space distance between geometric entities at asserted c
onnectivities') ;
#117147=UNCERTAINTY_MEASURE_WITH_UNIT(LENGTH_MEASURE(0.01),#117171,
'DISTANCE_ACCURACY_VALUE',
'Maximum model space distance between geometric entities at asserted c
onnectivities') ;
#117167=(
GEOMETRIC_REPRESENTATION_CONTEXT(3)
GLOBAL_UNCERTAINTY_ASSIGNED_CONTEXT((#117144))
GLOBAL_UNIT_ASSIGNED_CONTEXT((#117171,#117173,#117174))
REPRESENTATION_CONTEXT('','3D')
) ;
#117170=(
GEOMETRIC_REPRESENTATION_CONTEXT(3)
GLOBAL_UNCERTAINTY_ASSIGNED_CONTEXT((#117147))
GLOBAL_UNIT_ASSIGNED_CONTEXT((#117171,#117173,#117174))
REPRESENTATION_CONTEXT('','3D')
) ;
#117171=(
LENGTH_UNIT()
NAMED_UNIT(*)
SI_UNIT(.MILLI.,.METRE.)
) ;
#117173=(
NAMED_UNIT(*)
PLANE_ANGLE_UNIT()
SI_UNIT($,.RADIAN.)
) ;
#117174=(
NAMED_UNIT(*)
SI_UNIT($,.STERADIAN.)
SOLID_ANGLE_UNIT()
) ;
#117194=SHAPE_DEFINITION_REPRESENTATION(#117216,#117259) ;
#117216=PRODUCT_DEFINITION_SHAPE('',$,#117282) ;
#117259=SHAPE_REPRESENTATION('',(#54042),#117167) ;
#117262=PRODUCT_DEFINITION_CONTEXT('part definition',#117330,'design') ;
#117282=PRODUCT_DEFINITION('Knob_Grip_1','Knob_Grip_1',#117304,#117262) ;
#117304=PRODUCT_DEFINITION_FORMATION('',$,#117351) ;
#117330=APPLICATION_CONTEXT(
'Core Data for Automotive Mechanical Design Process') ;
#117331=PRODUCT_CONTEXT('part definition',#117330,'mechanical') ;
#117351=PRODUCT('Knob_Grip_1','Knob_Grip_1',$,(#117331)) ;
#117355=PRESENTATION_STYLE_ASSIGNMENT((#117357)) ;
#117357=SURFACE_STYLE_USAGE(.BOTH.,#117359) ;
#117359=SURFACE_SIDE_STYLE('',(#117361)) ;
#117361=SURFACE_STYLE_FILL_AREA(#117363) ;
#117363=FILL_AREA_STYLE('Opaque(160,160,160)',(#117365)) ;
#117365=FILL_AREA_STYLE_COLOUR('Opaque(160,160,160)',#117367) ;
#117367=COLOUR_RGB('Opaque(160,160,160)', 0.09019608, 0.27058824, 0.51372549) ;
ENDSEC;
END-ISO-10303-21;
